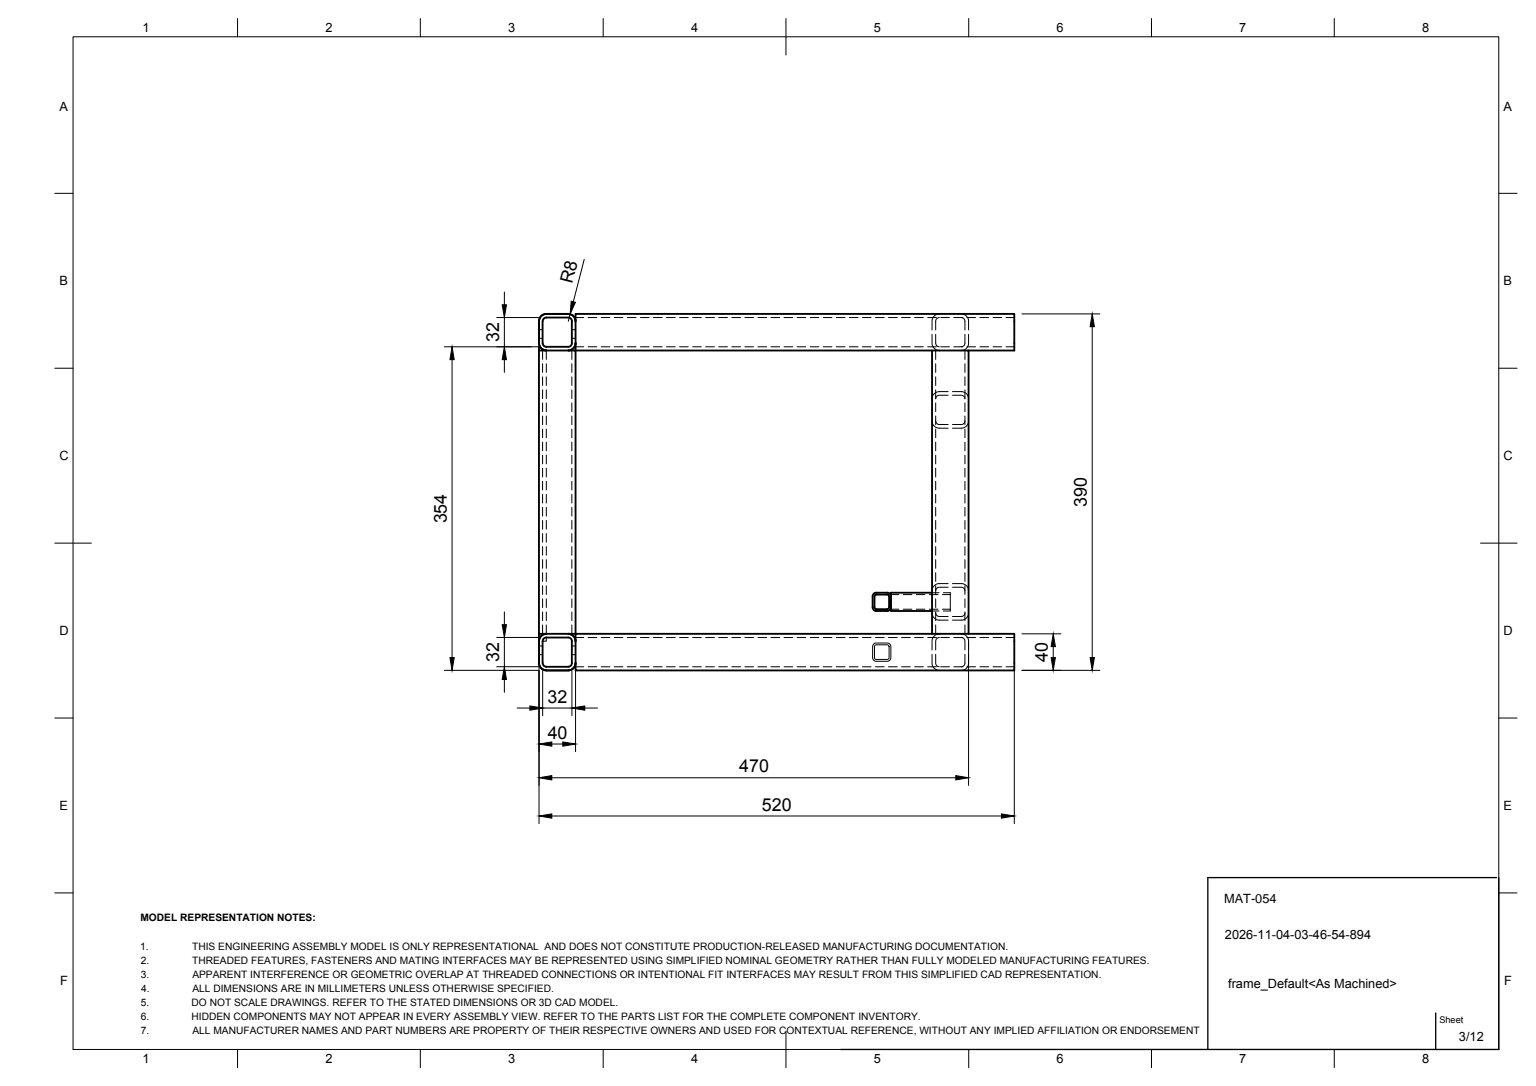
ISO-10303-21;
HEADER;
FILE_DESCRIPTION (('STEP AP214'),
    '1' );
FILE_NAME ('frame_Default<As Machined>.step',
    '2026-10-21T17:50:41',
    ( '' ),
    ( '' ),
    'SwSTEP 2.0',
    'SolidWorks 2026',
    '' );
FILE_SCHEMA (( 'AUTOMOTIVE_DESIGN' ));
ENDSEC;

DATA;
#1=CARTESIAN_POINT ( 'NONE',  ( -499.9999999999999432, -137.0000000000000000, -155.0000000000000000 ) ) ;
#4=CARTESIAN_POINT ( 'NONE',  ( -19.99999999999998934, 134.9999999999999432, -162.9999999999999432 ) ) ;
#6=DIRECTION ( 'NONE',  ( -0.000000000000000000, 0.000000000000000000, -1.000000000000000000 ) ) ;
#10=LINE ( 'NONE', #8370, #25873 ) ;
#17=CIRCLE ( 'NONE', #34681, 7.999999999999979572 ) ;
#21=LINE ( 'NONE', #19262, #12243 ) ;
#22=EDGE_CURVE ( 'NONE', #26361, #15713, #881, .T. ) ;
#25=LINE ( 'NONE', #27253, #34000 ) ;
#26=AXIS2_PLACEMENT_3D ( 'NONE', #32504, #14502, #28009 ) ;
#28=ORIENTED_EDGE ( 'NONE', *, *, #27270, .T. ) ;
#29=LINE ( 'NONE', #564, #14605 ) ;
#34=CARTESIAN_POINT ( 'NONE',  ( -449.9999999999999432, 137.0000000000000000, -175.0000000000000000 ) ) ;
#35=VERTEX_POINT ( 'NONE', #17374 ) ;
#37=DIRECTION ( 'NONE',  ( 0.000000000000000000, 1.000000000000000000, -3.421138828918010427E-49 ) ) ;
#39=ADVANCED_FACE ( 'NONE', ( #31052 ), #33181, .F. ) ;
#42=DIRECTION ( 'NONE',  ( 0.000000000000000000, -1.000000000000000000, -2.465190328815662439E-32 ) ) ;
#43=AXIS2_PLACEMENT_3D ( 'NONE', #14582, #6360, #9220 ) ;
#45=DIRECTION ( 'NONE',  ( 0.000000000000000000, -5.053935297177146739E-49, -1.000000000000000000 ) ) ;
#47=SHAPE_REPRESENTATION ( 'frame_Default<As Machined>', ( #28566 ), #4098 ) ;
#49=EDGE_LOOP ( 'NONE', ( #24690, #13383, #3512, #29102 ) ) ;
#51=CARTESIAN_POINT ( 'NONE',  ( 11.99999999999999645, 124.9999999999999716, 194.9999999999999716 ) ) ;
#52=DIRECTION ( 'NONE',  ( 1.000000000000000000, 0.000000000000000000, -1.848892746611746966E-32 ) ) ;
#60=ORIENTED_EDGE ( 'NONE', *, *, #3732, .F. ) ;
#61=DIRECTION ( 'NONE',  ( 0.000000000000000000, 6.123233995736766036E-17, 1.000000000000000000 ) ) ;
#63=ORIENTED_EDGE ( 'NONE', *, *, #23072, .F. ) ;
#68=EDGE_CURVE ( 'NONE', #14854, #22599, #23039, .T. ) ;
#73=ORIENTED_EDGE ( 'NONE', *, *, #26819, .F. ) ;
#74=DIRECTION ( 'NONE',  ( 0.000000000000000000, 0.000000000000000000, -1.000000000000000000 ) ) ;
#79=DIRECTION ( 'NONE',  ( 1.000000000000000000, 0.000000000000000000, -1.848892746611746966E-32 ) ) ;
#80=CIRCLE ( 'NONE', #11440, 7.999999999999979572 ) ;
#81=CARTESIAN_POINT ( 'NONE',  ( -365.0000000000000000, 118.9999999999999716, 130.0000000000000000 ) ) ;
#83=AXIS2_PLACEMENT_3D ( 'NONE', #4281, #34723, #15702 ) ;
#84=AXIS2_PLACEMENT_3D ( 'NONE', #29650, #6301, #461 ) ;
#87=DIRECTION ( 'NONE',  ( 0.000000000000000000, 1.310824597558155437E-49, 1.000000000000000000 ) ) ;
#90=ORIENTED_EDGE ( 'NONE', *, *, #18503, .T. ) ;
#91=FACE_OUTER_BOUND ( 'NONE', #10797, .T. ) ;
#93=CARTESIAN_POINT ( 'NONE',  ( -418.0000000000000000, -112.9999999999999858, -174.9999999999999716 ) ) ;
#94=CARTESIAN_POINT ( 'NONE',  ( -499.9999999999999432, 112.9999999999999574, 159.0000000000000000 ) ) ;
#96=VECTOR ( 'NONE', #6013, 1000.000000000000000 ) ;
#97=ORIENTED_EDGE ( 'NONE', *, *, #12534, .F. ) ;
#100=MANIFOLD_SOLID_BREP ( 'Square tube 40 X 40 X 4(1)[12]', #34815 ) ;
#101=ORIENTED_EDGE ( 'NONE', *, *, #29088, .F. ) ;
#103=AXIS2_PLACEMENT_3D ( 'NONE', #2451, #30043, #5636 ) ;
#104=AXIS2_PLACEMENT_3D ( 'NONE', #26124, #29507, #9931 ) ;
#106=CARTESIAN_POINT ( 'NONE',  ( -449.9999999999999432, -112.9999999999999858, -155.0000000000000000 ) ) ;
#108=VERTEX_POINT ( 'NONE', #26214 ) ;
#118=ORIENTED_EDGE ( 'NONE', *, *, #1367, .F. ) ;
#120=CARTESIAN_POINT ( 'NONE',  ( -418.0000000000000000, -105.0000000000000142, -73.99999999999998579 ) ) ;
#127=CARTESIAN_POINT ( 'NONE',  ( 11.99999999999999645, 124.9999999999999716, 190.9999999999999716 ) ) ;
#128=EDGE_LOOP ( 'NONE', ( #27295, #34610, #28913, #17445 ) ) ;
#130=EDGE_CURVE ( 'NONE', #18108, #30234, #23613, .T. ) ;
#132=CARTESIAN_POINT ( 'NONE',  ( -499.9999999999999432, 140.9999999999999716, -162.9999999999999716 ) ) ;
#135=CARTESIAN_POINT ( 'NONE',  ( -441.9999999999999432, -104.9999999999999716, -190.9999999999999716 ) ) ;
#139=ORIENTED_EDGE ( 'NONE', *, *, #14829, .T. ) ;
#140=CARTESIAN_POINT ( 'NONE',  ( -12.00000000000001066, -124.9999999999999432, -162.9999999999999432 ) ) ;
#143=VERTEX_POINT ( 'NONE', #21234 ) ;
#160=ORIENTED_EDGE ( 'NONE', *, *, #17632, .T. ) ;
#162=ORIENTED_EDGE ( 'NONE', *, *, #7088, .T. ) ;
#165=ADVANCED_FACE ( 'NONE', ( #4848 ), #1498, .F. ) ;
#166=DIRECTION ( 'NONE',  ( 1.000000000000000000, 0.000000000000000000, -1.232595164407831220E-32 ) ) ;
#169=VERTEX_POINT ( 'NONE', #10028 ) ;
#170=ADVANCED_FACE ( 'NONE', ( #26571 ), #17893, .T. ) ;
#172=DIRECTION ( 'NONE',  ( 0.000000000000000000, 1.310824597558155437E-49, 1.000000000000000000 ) ) ;
#173=VERTEX_POINT ( 'NONE', #23733 ) ;
#174=DIRECTION ( 'NONE',  ( -0.000000000000000000, 1.000000000000000000, -0.000000000000000000 ) ) ;
#178=ORIENTED_EDGE ( 'NONE', *, *, #30215, .F. ) ;
#181=VERTEX_POINT ( 'NONE', #21756 ) ;
#196=VERTEX_POINT ( 'NONE', #27097 ) ;
#203=CARTESIAN_POINT ( 'NONE',  ( -349.0000000000000000, 134.9999999999999716, 113.9999999999999858 ) ) ;
#204=FACE_OUTER_BOUND ( 'NONE', #17444, .T. ) ;
#208=ADVANCED_FACE ( 'NONE', ( #18929 ), #2537, .T. ) ;
#209=EDGE_CURVE ( 'NONE', #25754, #24825, #34950, .T. ) ;
#210=AXIS2_PLACEMENT_3D ( 'NONE', #14613, #8714, #19766 ) ;
#211=CARTESIAN_POINT ( 'NONE',  ( -15.99999999999998579, 124.9999999999999716, 162.9999999999999716 ) ) ;
#213=CYLINDRICAL_SURFACE ( 'NONE', #21558, 7.999999999999979572 ) ;
#216=ORIENTED_EDGE ( 'NONE', *, *, #5166, .F. ) ;
#217=CYLINDRICAL_SURFACE ( 'NONE', #9558, 3.999999999999976019 ) ;
#219=CARTESIAN_POINT ( 'NONE',  ( -500.0000000000000000, -137.0000000000000000, 190.9999999999999716 ) ) ;
#221=( NAMED_UNIT ( * ) PLANE_ANGLE_UNIT ( ) SI_UNIT ( $, .RADIAN. ) );
#228=ORIENTED_EDGE ( 'NONE', *, *, #6017, .T. ) ;
#229=DIRECTION ( 'NONE',  ( 1.000000000000000000, 0.000000000000000000, 0.000000000000000000 ) ) ;
#231=EDGE_CURVE ( 'NONE', #21456, #4465, #34436, .T. ) ;
#234=EDGE_CURVE ( 'NONE', #30170, #27211, #3153, .T. ) ;
#235=CIRCLE ( 'NONE', #12751, 3.999999999999976019 ) ;
#236=ORIENTED_EDGE ( 'NONE', *, *, #29739, .F. ) ;
#239=AXIS2_PLACEMENT_3D ( 'NONE', #27640, #18947, #27283 ) ;
#240=EDGE_CURVE ( 'NONE', #16352, #20441, #2589, .T. ) ;
#241=ORIENTED_EDGE ( 'NONE', *, *, #17416, .F. ) ;
#242=ORIENTED_EDGE ( 'NONE', *, *, #21753, .F. ) ;
#248=AXIS2_PLACEMENT_3D ( 'NONE', #6880, #17771, #4383 ) ;
#249=DIRECTION ( 'NONE',  ( -1.000000000000000000, 0.000000000000000000, 0.000000000000000000 ) ) ;
#250=CARTESIAN_POINT ( 'NONE',  ( -500.0000000000000000, 112.9999999999999574, 155.0000000000000000 ) ) ;
#259=ORIENTED_EDGE ( 'NONE', *, *, #5135, .T. ) ;
#260=ORIENTED_EDGE ( 'NONE', *, *, #32935, .F. ) ;
#262=VECTOR ( 'NONE', #31181, 1000.000000000000000 ) ;
#265=EDGE_LOOP ( 'NONE', ( #34746, #139, #23845, #12635, #26310, #31196, #6266, #393 ) ) ;
#266=CARTESIAN_POINT ( 'NONE',  ( 15.99999999999998579, 4.559999999999908127, 168.2400000000000091 ) ) ;
#281=CARTESIAN_POINT ( 'NONE',  ( -499.9999999999999432, -137.0000000000000000, -190.9999999999999716 ) ) ;
#284=EDGE_LOOP ( 'NONE', ( #25209, #30307, #21311, #18042 ) ) ;
#285=VECTOR ( 'NONE', #12711, 1000.000000000000000 ) ;
#287=VECTOR ( 'NONE', #30917, 1000.000000000000000 ) ;
#290=CARTESIAN_POINT ( 'NONE',  ( -418.0000000000000000, 113.0000000000000000, 154.9999999999999716 ) ) ;
#295=CARTESIAN_POINT ( 'NONE',  ( -445.9999999999999432, -137.0000000000000000, 154.9999999999999716 ) ) ;
#296=DIRECTION ( 'NONE',  ( 0.000000000000000000, 1.000000000000000000, 0.000000000000000000 ) ) ;
#299=ORIENTED_EDGE ( 'NONE', *, *, #29304, .T. ) ;
#300=DIRECTION ( 'NONE',  ( 1.000000000000000000, 3.040835319149746528E-31, 1.232595164407830946E-32 ) ) ;
#302=CARTESIAN_POINT ( 'NONE',  ( -12.00000000000001066, -109.0000000000000142, 155.0000000000000000 ) ) ;
#304=VECTOR ( 'NONE', #8203, 1000.000000000000000 ) ;
#309=VECTOR ( 'NONE', #16304, 1000.000000000000000 ) ;
#313=ORIENTED_EDGE ( 'NONE', *, *, #17871, .T. ) ;
#315=ORIENTED_EDGE ( 'NONE', *, *, #26179, .T. ) ;
#316=VECTOR ( 'NONE', #20254, 1000.000000000000000 ) ;
#317=VECTOR ( 'NONE', #9866, 1000.000000000000000 ) ;
#321=CARTESIAN_POINT ( 'NONE',  ( 11.99999999999999645, -124.9999999999999432, -154.9999999999999716 ) ) ;
#322=AXIS2_PLACEMENT_3D ( 'NONE', #10565, #32080, #10742 ) ;
#330=DIRECTION ( 'NONE',  ( 0.000000000000000000, -1.224646799147353207E-16, 1.000000000000000000 ) ) ;
#333=EDGE_LOOP ( 'NONE', ( #9601, #2215, #28741, #29275, #5602, #22316, #13085, #21357 ) ) ;
#337=AXIS2_PLACEMENT_3D ( 'NONE', #12188, #9323, #17539 ) ;
#338=PLANE ( 'NONE',  #21235 ) ;
#345=ORIENTED_EDGE ( 'NONE', *, *, #32175, .T. ) ;
#347=DIRECTION ( 'NONE',  ( 0.000000000000000000, -1.000000000000000000, -2.465190328815662439E-32 ) ) ;
#351=ORIENTED_EDGE ( 'NONE', *, *, #29532, .T. ) ;
#352=ORIENTED_EDGE ( 'NONE', *, *, #24437, .F. ) ;
#354=ORIENTED_EDGE ( 'NONE', *, *, #15930, .T. ) ;
#355=CARTESIAN_POINT ( 'NONE',  ( -20.00000000000007461, 104.9999999999999858, -162.9999999999999716 ) ) ;
#356=CARTESIAN_POINT ( 'NONE',  ( -414.0000000000000568, -124.9999999999999858, -77.99999999999997158 ) ) ;
#358=EDGE_LOOP ( 'NONE', ( #6537, #22025, #25095, #26334 ) ) ;
#359=CIRCLE ( 'NONE', #19122, 3.999999999999976019 ) ;
#362=DIRECTION ( 'NONE',  ( -0.000000000000000000, 1.000000000000000000, -0.000000000000000000 ) ) ;
#365=DIRECTION ( 'NONE',  ( 0.000000000000000000, 1.000000000000000000, 5.145227585319922065E-49 ) ) ;
#366=DIRECTION ( 'NONE',  ( 0.000000000000000000, 0.000000000000000000, 1.000000000000000000 ) ) ;
#367=EDGE_CURVE ( 'NONE', #31738, #21426, #28743, .T. ) ;
#368=LINE ( 'NONE', #5152, #16717 ) ;
#370=CARTESIAN_POINT ( 'NONE',  ( -19.99999999999998934, 144.9999999999999147, 162.9999999999999716 ) ) ;
#372=PLANE ( 'NONE',  #748 ) ;
#373=EDGE_CURVE ( 'NONE', #12936, #16352, #14295, .T. ) ;
#377=LINE ( 'NONE', #5513, #1804 ) ;
#386=CARTESIAN_POINT ( 'NONE',  ( -349.0000000000000000, -125.0000000000000284, 168.9999999999999716 ) ) ;
#387=AXIS2_PLACEMENT_3D ( 'NONE', #34628, #13273, #5228 ) ;
#388=CARTESIAN_POINT ( 'NONE',  ( -499.9999999999999432, 136.9999999999999432, -159.0000000000000000 ) ) ;
#390=DIRECTION ( 'NONE',  ( 0.000000000000000000, 0.000000000000000000, -1.000000000000000000 ) ) ;
#392=VERTEX_POINT ( 'NONE', #6605 ) ;
#393=ORIENTED_EDGE ( 'NONE', *, *, #6508, .T. ) ;
#395=CARTESIAN_POINT ( 'NONE',  ( -355.0000000000000000, 132.9999999999999716, 113.9999999999999858 ) ) ;
#396=AXIS2_PLACEMENT_3D ( 'NONE', #7173, #18412, #15218 ) ;
#397=LINE ( 'NONE', #6768, #1059 ) ;
#398=CARTESIAN_POINT ( 'NONE',  ( -499.9999999999999432, -137.0000000000000000, -159.0000000000000000 ) ) ;
#402=CARTESIAN_POINT ( 'NONE',  ( -363.0000000000000000, -135.0000000000000000, 114.0000000000000000 ) ) ;
#406=VECTOR ( 'NONE', #1614, 1000.000000000000000 ) ;
#407=DIRECTION ( 'NONE',  ( 0.000000000000000000, 6.123233995736766036E-17, 1.000000000000000000 ) ) ;
#411=CARTESIAN_POINT ( 'NONE',  ( -20.00000000000004619, -124.9999999999999432, -194.9999999999999432 ) ) ;
#413=DIRECTION ( 'NONE',  ( 1.000000000000000000, -0.000000000000000000, 0.000000000000000000 ) ) ;
#414=FACE_OUTER_BOUND ( 'NONE', #24829, .T. ) ;
#418=EDGE_CURVE ( 'NONE', #32157, #25965, #6244, .T. ) ;
#421=ORIENTED_EDGE ( 'NONE', *, *, #373, .F. ) ;
#423=VERTEX_POINT ( 'NONE', #6428 ) ;
#426=EDGE_CURVE ( 'NONE', #7666, #28875, #25652, .T. ) ;
#429=CARTESIAN_POINT ( 'NONE',  ( -418.0000000000000000, 124.9999999999999432, -162.9999999999999716 ) ) ;
#430=PLANE ( 'NONE',  #10872 ) ;
#440=EDGE_CURVE ( 'NONE', #10023, #18562, #30296, .T. ) ;
#443=DIRECTION ( 'NONE',  ( -0.000000000000000000, 1.000000000000000000, -0.000000000000000000 ) ) ;
#451=AXIS2_PLACEMENT_3D ( 'NONE', #17742, #12395, #1529 ) ;
#454=PLANE ( 'NONE',  #18923 ) ;
#457=ORIENTED_EDGE ( 'NONE', *, *, #17828, .T. ) ;
#459=ADVANCED_FACE ( 'NONE', ( #16977 ), #27625, .T. ) ;
#460=DIRECTION ( 'NONE',  ( -1.000000000000000000, 0.000000000000000000, -1.300283923313630633E-47 ) ) ;
#461=DIRECTION ( 'NONE',  ( -1.000000000000000000, 0.000000000000000000, 0.000000000000000000 ) ) ;
#463=ORIENTED_EDGE ( 'NONE', *, *, #15359, .T. ) ;
#464=AXIS2_PLACEMENT_3D ( 'NONE', #20405, #28583, #17576 ) ;
#465=ORIENTED_EDGE ( 'NONE', *, *, #4049, .T. ) ;
#468=ORIENTED_EDGE ( 'NONE', *, *, #12591, .T. ) ;
#470=CARTESIAN_POINT ( 'NONE',  ( -445.9999999999999432, 105.0000000000000000, -77.99999999999997158 ) ) ;
#473=CARTESIAN_POINT ( 'NONE',  ( -499.9999999999999432, 112.9999999999999574, -159.0000000000000000 ) ) ;
#476=CYLINDRICAL_SURFACE ( 'NONE', #3727, 7.999999999999979572 ) ;
#481=VECTOR ( 'NONE', #14446, 1000.000000000000000 ) ;
#490=CARTESIAN_POINT ( 'NONE',  ( -414.0000000000000568, 105.0000000000000000, 132.0000000000000000 ) ) ;
#493=VERTEX_POINT ( 'NONE', #26528 ) ;
#495=DIRECTION ( 'NONE',  ( 0.000000000000000000, 2.309213040847544338E-50, 1.000000000000000000 ) ) ;
#496=EDGE_LOOP ( 'NONE', ( #8671, #8496, #20597, #12284 ) ) ;
#497=DIRECTION ( 'NONE',  ( -5.546364386991661285E-52, 0.000000000000000000, -1.000000000000000000 ) ) ;
#499=VECTOR ( 'NONE', #8880, 1000.000000000000000 ) ;
#502=DIRECTION ( 'NONE',  ( 1.000000000000000000, 0.000000000000000000, -1.232595164407831220E-32 ) ) ;
#503=PLANE ( 'NONE',  #5402 ) ;
#510=FACE_OUTER_BOUND ( 'NONE', #7829, .T. ) ;
#512=LINE ( 'NONE', #33420, #24339 ) ;
#516=ORIENTED_EDGE ( 'NONE', *, *, #603, .F. ) ;
#518=ORIENTED_EDGE ( 'NONE', *, *, #18226, .F. ) ;
#519=DIRECTION ( 'NONE',  ( 0.000000000000000000, 1.131431318426415506E-52, 1.000000000000000000 ) ) ;
#520=ADVANCED_FACE ( 'NONE', ( #26170 ), #21018, .T. ) ;
#521=CARTESIAN_POINT ( 'NONE',  ( -20.00000000000007461, 112.9999999999999574, 162.9999999999999716 ) ) ;
#525=CIRCLE ( 'NONE', #16796, 7.999999999999979572 ) ;
#529=ORIENTED_EDGE ( 'NONE', *, *, #33922, .T. ) ;
#530=CYLINDRICAL_SURFACE ( 'NONE', #3882, 4.000000000000003553 ) ;
#531=CYLINDRICAL_SURFACE ( 'NONE', #29653, 7.999999999999979572 ) ;
#533=VECTOR ( 'NONE', #26637, 1000.000000000000000 ) ;
#534=ORIENTED_EDGE ( 'NONE', *, *, #6126, .F. ) ;
#540=PLANE ( 'NONE',  #20688 ) ;
#541=AXIS2_PLACEMENT_3D ( 'NONE', #20921, #31768, #29104 ) ;
#542=CARTESIAN_POINT ( 'NONE',  ( -499.9999999999999432, -113.0000000000000000, -162.9999999999999716 ) ) ;
#545=ORIENTED_EDGE ( 'NONE', *, *, #1677, .T. ) ;
#553=EDGE_CURVE ( 'NONE', #7666, #18883, #20841, .T. ) ;
#554=ORIENTED_EDGE ( 'NONE', *, *, #3009, .T. ) ;
#555=DIRECTION ( 'NONE',  ( 0.000000000000000000, 1.000000000000000000, 5.145227585319922065E-49 ) ) ;
#558=AXIS2_PLACEMENT_3D ( 'NONE', #28352, #26018, #20687 ) ;
#560=FACE_OUTER_BOUND ( 'NONE', #15965, .T. ) ;
#561=CARTESIAN_POINT ( 'NONE',  ( -410.0000000000000568, 104.9999999999999858, -175.0000000000000000 ) ) ;
#563=ORIENTED_EDGE ( 'NONE', *, *, #30172, .T. ) ;
#564=CARTESIAN_POINT ( 'NONE',  ( -499.9999999999999432, 136.9999999999999432, -155.0000000000000000 ) ) ;
#567=DIRECTION ( 'NONE',  ( 1.000000000000000000, 0.000000000000000000, 0.000000000000000000 ) ) ;
#568=DIRECTION ( 'NONE',  ( 0.000000000000000000, -1.000000000000000000, 0.000000000000000000 ) ) ;
#569=ORIENTED_EDGE ( 'NONE', *, *, #971, .T. ) ;
#571=DIRECTION ( 'NONE',  ( 1.000000000000000000, 0.000000000000000000, -1.848892746611746966E-32 ) ) ;
#573=ORIENTED_EDGE ( 'NONE', *, *, #23821, .T. ) ;
#574=LINE ( 'NONE', #16262, #35090 ) ;
#575=CARTESIAN_POINT ( 'NONE',  ( -418.0000000000000000, -145.0000000000000000, -175.0000000000000000 ) ) ;
#576=EDGE_CURVE ( 'NONE', #19034, #23318, #12495, .T. ) ;
#577=CARTESIAN_POINT ( 'NONE',  ( -499.9999999999999432, 136.9999999999999432, -190.9999999999999716 ) ) ;
#580=DIRECTION ( 'NONE',  ( 0.000000000000000000, 1.000000000000000000, 5.145227585319922065E-49 ) ) ;
#581=ORIENTED_EDGE ( 'NONE', *, *, #14404, .F. ) ;
#582=DIRECTION ( 'NONE',  ( 0.000000000000000000, 1.310824597558155437E-49, 1.000000000000000000 ) ) ;
#586=ORIENTED_EDGE ( 'NONE', *, *, #10577, .T. ) ;
#591=VERTEX_POINT ( 'NONE', #18194 ) ;
#596=LINE ( 'NONE', #19835, #27348 ) ;
#599=FACE_OUTER_BOUND ( 'NONE', #6843, .T. ) ;
#601=LINE ( 'NONE', #17003, #7250 ) ;
#603=EDGE_CURVE ( 'NONE', #26714, #17291, #15511, .T. ) ;
#606=DIRECTION ( 'NONE',  ( -0.000000000000000000, 1.000000000000000000, -0.000000000000000000 ) ) ;
#618=CARTESIAN_POINT ( 'NONE',  ( 15.99999999999998579, 4.559999999999908127, -172.9900000000000091 ) ) ;
#621=LINE ( 'NONE', #27139, #28055 ) ;
#623=ORIENTED_EDGE ( 'NONE', *, *, #12621, .T. ) ;
#626=EDGE_CURVE ( 'NONE', #20682, #8601, #10335, .T. ) ;
#627=ORIENTED_EDGE ( 'NONE', *, *, #29512, .F. ) ;
#629=CARTESIAN_POINT ( 'NONE',  ( 12.00000000000001066, -134.9999999999999716, 194.9999999999999716 ) ) ;
#630=AXIS2_PLACEMENT_3D ( 'NONE', #7025, #15243, #23764 ) ;
#632=AXIS2_PLACEMENT_3D ( 'NONE', #14720, #8823, #19878 ) ;
#639=VERTEX_POINT ( 'NONE', #21379 ) ;
#643=CARTESIAN_POINT ( 'NONE',  ( 11.99999999999995559, -145.0000000000000000, 194.9999999999999716 ) ) ;
#651=STYLED_ITEM('',(#35254),#22717);
#652=LINE ( 'NONE', #11513, #1580 ) ;
#654=CARTESIAN_POINT ( 'NONE',  ( -70.00000000000000000, 75.55999999999990280, -172.9900000000000091 ) ) ;
#656=ADVANCED_FACE ( 'NONE', ( #2312 ), #27058, .F. ) ;
#658=CARTESIAN_POINT ( 'NONE',  ( 12.00000000000001066, 134.9999999999999432, -154.9999999999999716 ) ) ;
#664=LINE ( 'NONE', #5982, #1831 ) ;
#665=ORIENTED_EDGE ( 'NONE', *, *, #8099, .F. ) ;
#666=FACE_OUTER_BOUND ( 'NONE', #16803, .T. ) ;
#672=ORIENTED_EDGE ( 'NONE', *, *, #22907, .F. ) ;
#677=LINE ( 'NONE', #11000, #15466 ) ;
#678=CIRCLE ( 'NONE', #20570, 3.999999999999976019 ) ;
#687=EDGE_CURVE ( 'NONE', #28835, #181, #8010, .T. ) ;
#688=VECTOR ( 'NONE', #24666, 1000.000000000000000 ) ;
#690=DIRECTION ( 'NONE',  ( -1.000000000000000000, 8.433758354584418579E-81, -1.232595164407830946E-32 ) ) ;
#692=ORIENTED_EDGE ( 'NONE', *, *, #2681, .F. ) ;
#695=PRODUCT ( 'frame_Default<As Machined>', 'frame_Default<As Machined>', '', ( #11065 ) ) ;
#697=CIRCLE ( 'NONE', #1800, 4.750000000000004441 ) ;
#699=AXIS2_PLACEMENT_3D ( 'NONE', #32555, #29554, #17888 ) ;
#703=AXIS2_PLACEMENT_3D ( 'NONE', #2442, #2103, #14812 ) ;
#705=DIRECTION ( 'NONE',  ( 0.000000000000000000, 0.000000000000000000, 1.000000000000000000 ) ) ;
#707=VERTEX_POINT ( 'NONE', #16225 ) ;
#709=( NAMED_UNIT ( * ) PLANE_ANGLE_UNIT ( ) SI_UNIT ( $, .RADIAN. ) );
#711=ORIENTED_EDGE ( 'NONE', *, *, #4540, .T. ) ;
#714=CARTESIAN_POINT ( 'NONE',  ( -500.0000000000000000, -113.0000000000000000, 194.9999999999999716 ) ) ;
#718=ORIENTED_EDGE ( 'NONE', *, *, #26278, .T. ) ;
#721=EDGE_CURVE ( 'NONE', #11831, #17160, #30086, .T. ) ;
#722=ORIENTED_EDGE ( 'NONE', *, *, #5518, .F. ) ;
#726=VERTEX_POINT ( 'NONE', #16403 ) ;
#727=ORIENTED_EDGE ( 'NONE', *, *, #801, .T. ) ;
#728=DIRECTION ( 'NONE',  ( 0.000000000000000000, 1.000000000000000000, 0.000000000000000000 ) ) ;
#734=CARTESIAN_POINT ( 'NONE',  ( -500.0000000000000000, -137.0000000000000000, 187.0000000000000000 ) ) ;
#735=CARTESIAN_POINT ( 'NONE',  ( -500.0000000000000000, -137.0000000000000000, 159.0000000000000000 ) ) ;
#737=ORIENTED_EDGE ( 'NONE', *, *, #1707, .T. ) ;
#739=DIRECTION ( 'NONE',  ( 1.000000000000000000, 0.000000000000000000, 0.000000000000000000 ) ) ;
#745=CYLINDRICAL_SURFACE ( 'NONE', #8305, 7.999999999999979572 ) ;
#746=DIRECTION ( 'NONE',  ( -1.000000000000000000, 0.000000000000000000, -1.300283923313630633E-47 ) ) ;
#748=AXIS2_PLACEMENT_3D ( 'NONE', #8542, #14074, #33456 ) ;
#753=PLANE ( 'NONE',  #13835 ) ;
#759=CARTESIAN_POINT ( 'NONE',  ( -363.0000000000000000, -135.0000000000000000, 114.0000000000000000 ) ) ;
#760=DIRECTION ( 'NONE',  ( -0.000000000000000000, -5.145227585319922065E-49, -1.000000000000000000 ) ) ;
#761=EDGE_CURVE ( 'NONE', #19084, #9157, #24545, .T. ) ;
#763=VERTEX_POINT ( 'NONE', #5153 ) ;
#768=VECTOR ( 'NONE', #8009, 1000.000000000000000 ) ;
#770=CARTESIAN_POINT ( 'NONE',  ( -442.0000000000000000, -125.0000000000000000, -105.9999999999999574 ) ) ;
#773=CARTESIAN_POINT ( 'NONE',  ( -499.9999999999999432, -113.0000000000000000, -162.9999999999999716 ) ) ;
#774=ORIENTED_EDGE ( 'NONE', *, *, #8706, .F. ) ;
#775=LINE ( 'NONE', #34040, #30580 ) ;
#777=ORIENTED_EDGE ( 'NONE', *, *, #34334, .F. ) ;
#778=ORIENTED_EDGE ( 'NONE', *, *, #32742, .T. ) ;
#779=FACE_OUTER_BOUND ( 'NONE', #30050, .T. ) ;
#780=DIRECTION ( 'NONE',  ( 0.000000000000000000, 1.000000000000000000, 5.145227585319922065E-49 ) ) ;
#782=DIRECTION ( 'NONE',  ( 0.000000000000000000, 1.000000000000000000, 2.465190328815662439E-32 ) ) ;
#783=PLANE ( 'NONE',  #1217 ) ;
#785=CARTESIAN_POINT ( 'NONE',  ( -20.00000000000007461, 136.9999999999999432, 190.9999999999999716 ) ) ;
#788=ORIENTED_EDGE ( 'NONE', *, *, #21266, .F. ) ;
#789=CARTESIAN_POINT ( 'NONE',  ( -499.9999999999999432, 112.9999999999999574, 190.9999999999999716 ) ) ;
#793=LINE ( 'NONE', #15037, #16102 ) ;
#794=AXIS2_PLACEMENT_3D ( 'NONE', #34240, #4849, #18070 ) ;
#800=FACE_OUTER_BOUND ( 'NONE', #12597, .T. ) ;
#801=EDGE_CURVE ( 'NONE', #5991, #17491, #18552, .T. ) ;
#809=EDGE_CURVE ( 'NONE', #1130, #16248, #20815, .T. ) ;
#813=ORIENTED_EDGE ( 'NONE', *, *, #20854, .T. ) ;
#817=EDGE_CURVE ( 'NONE', #591, #27019, #22610, .T. ) ;
#819=LINE ( 'NONE', #5782, #3363 ) ;
#820=AXIS2_PLACEMENT_3D ( 'NONE', #3238, #14113, #27797 ) ;
#823=ORIENTED_EDGE ( 'NONE', *, *, #1952, .F. ) ;
#825=AXIS2_PLACEMENT_3D ( 'NONE', #30486, #20162, #31187 ) ;
#829=DIRECTION ( 'NONE',  ( 0.000000000000000000, 0.000000000000000000, -1.000000000000000000 ) ) ;
#832=LINE ( 'NONE', #5974, #7684 ) ;
#836=CARTESIAN_POINT ( 'NONE',  ( -15.99999999999998579, 136.9999999999999716, -175.0000000000000284 ) ) ;
#837=DIRECTION ( 'NONE',  ( 0.000000000000000000, 1.000000000000000000, 1.224646799147353207E-16 ) ) ;
#838=ORIENTED_EDGE ( 'NONE', *, *, #33279, .T. ) ;
#841=DIRECTION ( 'NONE',  ( 0.000000000000000000, -1.000000000000000000, 6.123233995736766036E-17 ) ) ;
#842=VERTEX_POINT ( 'NONE', #31436 ) ;
#844=CARTESIAN_POINT ( 'NONE',  ( -365.0000000000000000, 130.9999999999999716, 111.9999999999999858 ) ) ;
#847=CARTESIAN_POINT ( 'NONE',  ( -349.0000000000000000, 134.9999999999999716, 126.0000000000000000 ) ) ;
#849=ORIENTED_EDGE ( 'NONE', *, *, #21052, .T. ) ;
#851=FACE_OUTER_BOUND ( 'NONE', #26589, .T. ) ;
#854=VECTOR ( 'NONE', #2989, 1000.000000000000000 ) ;
#857=ADVANCED_FACE ( 'NONE', ( #30253 ), #22251, .F. ) ;
#862=CARTESIAN_POINT ( 'NONE',  ( -430.0000000000000000, -119.0000000000000000, 111.9999999999999858 ) ) ;
#864=CIRCLE ( 'NONE', #19071, 4.000000000000003553 ) ;
#867=ORIENTED_EDGE ( 'NONE', *, *, #33939, .F. ) ;
#868=ORIENTED_EDGE ( 'NONE', *, *, #240, .F. ) ;
#871=VECTOR ( 'NONE', #29284, 1000.000000000000000 ) ;
#873=DIRECTION ( 'NONE',  ( 1.000000000000000000, 0.000000000000000000, 0.000000000000000000 ) ) ;
#874=DIRECTION ( 'NONE',  ( 0.000000000000000000, 0.000000000000000000, 1.000000000000000000 ) ) ;
#875=FACE_OUTER_BOUND ( 'NONE', #18381, .T. ) ;
#877=ORIENTED_EDGE ( 'NONE', *, *, #2719, .T. ) ;
#878=AXIS2_PLACEMENT_3D ( 'NONE', #15837, #32184, #18849 ) ;
#879=DIRECTION ( 'NONE',  ( 0.000000000000000000, 0.000000000000000000, -1.000000000000000000 ) ) ;
#881=CIRCLE ( 'NONE', #13382, 4.750000000000004441 ) ;
#882=EDGE_CURVE ( 'NONE', #28417, #9255, #19687, .T. ) ;
#883=CARTESIAN_POINT ( 'NONE',  ( -442.0000000000000000, -124.9999999999999858, -77.99999999999997158 ) ) ;
#884=DIRECTION ( 'NONE',  ( 0.000000000000000000, 0.000000000000000000, -1.000000000000000000 ) ) ;
#887=EDGE_CURVE ( 'NONE', #24475, #21957, #33276, .T. ) ;
#888=FACE_OUTER_BOUND ( 'NONE', #22918, .T. ) ;
#889=CYLINDRICAL_SURFACE ( 'NONE', #9256, 3.999999999999976019 ) ;
#890=VERTEX_POINT ( 'NONE', #25929 ) ;
#892=CARTESIAN_POINT ( 'NONE',  ( 15.99999999999998579, -137.0000000000000000, -155.0000000000000284 ) ) ;
#895=VECTOR ( 'NONE', #17120, 1000.000000000000000 ) ;
#897=DIRECTION ( 'NONE',  ( 0.000000000000000000, 0.000000000000000000, 1.000000000000000000 ) ) ;
#898=AXIS2_PLACEMENT_3D ( 'NONE', #26736, #2349, #13228 ) ;
#899=ORIENTED_EDGE ( 'NONE', *, *, #20430, .F. ) ;
#901=EDGE_CURVE ( 'NONE', #33356, #2161, #3374, .T. ) ;
#904=VERTEX_POINT ( 'NONE', #6207 ) ;
#905=AXIS2_PLACEMENT_3D ( 'NONE', #32431, #24589, #8050 ) ;
#910=ORIENTED_EDGE ( 'NONE', *, *, #5324, .F. ) ;
#911=CARTESIAN_POINT ( 'NONE',  ( -365.0000000000000000, -117.0000000000000000, 113.9999999999999858 ) ) ;
#914=CARTESIAN_POINT ( 'NONE',  ( -363.0000000000000000, -135.0000000000000000, 126.0000000000000000 ) ) ;
#918=CARTESIAN_POINT ( 'NONE',  ( -449.9999999999999432, -124.9999999999999716, 132.0000000000000000 ) ) ;
#920=DIRECTION ( 'NONE',  ( 0.000000000000000000, 0.000000000000000000, -1.000000000000000000 ) ) ;
#921=CARTESIAN_POINT ( 'NONE',  ( -449.9999999999999432, -125.0000000000000000, 187.0000000000000000 ) ) ;
#922=DIRECTION ( 'NONE',  ( 1.000000000000000000, -0.000000000000000000, 0.000000000000000000 ) ) ;
#924=EDGE_CURVE ( 'NONE', #20300, #23023, #4196, .T. ) ;
#927=CARTESIAN_POINT ( 'NONE',  ( -19.99999999999998934, 124.9999999999999716, 155.0000000000000000 ) ) ;
#928=ORIENTED_EDGE ( 'NONE', *, *, #4882, .F. ) ;
#931=CARTESIAN_POINT ( 'NONE',  ( -499.9999999999999432, 136.9999999999999432, -159.0000000000000000 ) ) ;
#935=AXIS2_PLACEMENT_3D ( 'NONE', #4865, #34789, #15576 ) ;
#941=DIRECTION ( 'NONE',  ( -1.000000000000000000, 0.000000000000000000, 0.000000000000000000 ) ) ;
#944=ORIENTED_EDGE ( 'NONE', *, *, #27551, .T. ) ;
#945=CIRCLE ( 'NONE', #12819, 4.000000000000003553 ) ;
#948=CARTESIAN_POINT ( 'NONE',  ( -12.00000000000001066, 104.9999999999999858, -155.0000000000000000 ) ) ;
#953=VECTOR ( 'NONE', #12900, 1000.000000000000000 ) ;
#955=ORIENTED_EDGE ( 'NONE', *, *, #9993, .T. ) ;
#957=DIRECTION ( 'NONE',  ( 0.000000000000000000, 0.000000000000000000, -1.000000000000000000 ) ) ;
#958=EDGE_LOOP ( 'NONE', ( #8878, #27960, #18209, #24992 ) ) ;
#959=ORIENTED_EDGE ( 'NONE', *, *, #2723, .T. ) ;
#961=DIRECTION ( 'NONE',  ( -1.000000000000000000, 0.000000000000000000, 0.000000000000000000 ) ) ;
#966=CARTESIAN_POINT ( 'NONE',  ( -12.00000000000003908, -134.9999999999999716, -154.9999999999999716 ) ) ;
#967=ORIENTED_EDGE ( 'NONE', *, *, #21553, .T. ) ;
#969=AXIS2_PLACEMENT_3D ( 'NONE', #27218, #29899, #2828 ) ;
#970=DIRECTION ( 'NONE',  ( 1.000000000000000000, 0.000000000000000000, -1.232595164407831220E-32 ) ) ;
#971=EDGE_CURVE ( 'NONE', #5416, #26553, #2066, .T. ) ;
#973=ORIENTED_EDGE ( 'NONE', *, *, #9241, .T. ) ;
#974=DIRECTION ( 'NONE',  ( -0.000000000000000000, 1.000000000000000000, 0.000000000000000000 ) ) ;
#977=PLANE ( 'NONE',  #12699 ) ;
#978=DIRECTION ( 'NONE',  ( 1.000000000000000000, 0.000000000000000000, 0.000000000000000000 ) ) ;
#980=VERTEX_POINT ( 'NONE', #12938 ) ;
#983=PLANE ( 'NONE',  #23120 ) ;
#986=FACE_OUTER_BOUND ( 'NONE', #14814, .T. ) ;
#988=ORIENTED_EDGE ( 'NONE', *, *, #13058, .F. ) ;
#993=CARTESIAN_POINT ( 'NONE',  ( -445.9999999999999432, 104.9999999999999858, -162.9999999999999716 ) ) ;
#995=VERTEX_POINT ( 'NONE', #18457 ) ;
#1000=LINE ( 'NONE', #22721, #30171 ) ;
#1001=VERTEX_POINT ( 'NONE', #4369 ) ;
#1005=DIRECTION ( 'NONE',  ( 1.000000000000000000, -0.000000000000000000, -0.000000000000000000 ) ) ;
#1007=EDGE_CURVE ( 'NONE', #10470, #34124, #5457, .T. ) ;
#1014=ORIENTED_EDGE ( 'NONE', *, *, #28076, .T. ) ;
#1016=LINE ( 'NONE', #17232, #19707 ) ;
#1017=DIRECTION ( 'NONE',  ( 0.000000000000000000, 1.310824597558155437E-49, 1.000000000000000000 ) ) ;
#1019=EDGE_LOOP ( 'NONE', ( #8379, #30017, #22732, #21816 ) ) ;
#1020=AXIS2_PLACEMENT_3D ( 'NONE', #3481, #19182, #27167 ) ;
#1025=EDGE_CURVE ( 'NONE', #26862, #18446, #31608, .T. ) ;
#1027=ORIENTED_EDGE ( 'NONE', *, *, #16202, .T. ) ;
#1028=DIRECTION ( 'NONE',  ( -3.040835319149746090E-31, -1.000000000000000000, 3.748118910144520367E-63 ) ) ;
#1031=VERTEX_POINT ( 'NONE', #26619 ) ;
#1034=ORIENTED_EDGE ( 'NONE', *, *, #29447, .F. ) ;
#1035=FACE_BOUND ( 'NONE', #9089, .T. ) ;
#1036=FACE_OUTER_BOUND ( 'NONE', #26947, .T. ) ;
#1038=VECTOR ( 'NONE', #10976, 1000.000000000000000 ) ;
#1042=ORIENTED_EDGE ( 'NONE', *, *, #9870, .T. ) ;
#1044=ORIENTED_EDGE ( 'NONE', *, *, #6337, .F. ) ;
#1046=PLANE ( 'NONE',  #15456 ) ;
#1047=AXIS2_PLACEMENT_3D ( 'NONE', #8394, #6728, #13919 ) ;
#1055=EDGE_CURVE ( 'NONE', #26315, #29922, #21463, .T. ) ;
#1058=DIRECTION ( 'NONE',  ( -1.000000000000000000, -3.469446951953834515E-18, 0.000000000000000000 ) ) ;
#1059=VECTOR ( 'NONE', #20484, 1000.000000000000000 ) ;
#1068=LINE ( 'NONE', #892, #6351 ) ;
#1069=CARTESIAN_POINT ( 'NONE',  ( 19.99999999999998224, 134.9999999999998863, 187.0000000000000000 ) ) ;
#1070=CIRCLE ( 'NONE', #29493, 4.750000000000004441 ) ;
#1072=DIRECTION ( 'NONE',  ( -1.000000000000000000, 0.000000000000000000, -1.300283923313630633E-47 ) ) ;
#1073=CARTESIAN_POINT ( 'NONE',  ( 19.99999999999998224, 134.9999999999999432, -186.9999999999999716 ) ) ;
#1076=ORIENTED_EDGE ( 'NONE', *, *, #23191, .F. ) ;
#1086=DIRECTION ( 'NONE',  ( -1.000000000000000000, 0.000000000000000000, 0.000000000000000000 ) ) ;
#1092=DIRECTION ( 'NONE',  ( -1.000000000000000000, 0.000000000000000000, 0.000000000000000000 ) ) ;
#1094=DIRECTION ( 'NONE',  ( 0.000000000000000000, 1.131431318426415506E-52, 1.000000000000000000 ) ) ;
#1095=VERTEX_POINT ( 'NONE', #3288 ) ;
#1107=CARTESIAN_POINT ( 'NONE',  ( -418.0000000000000000, 105.0000000000000000, -69.99999999999998579 ) ) ;
#1109=CARTESIAN_POINT ( 'NONE',  ( 19.99999999999998224, 134.9999999999998863, 187.0000000000000000 ) ) ;
#1111=ORIENTED_EDGE ( 'NONE', *, *, #27207, .F. ) ;
#1115=ORIENTED_EDGE ( 'NONE', *, *, #13293, .F. ) ;
#1117=MANIFOLD_SOLID_BREP ( 'Trim/Extend7[2]', #17953 ) ;
#1118=ORIENTED_EDGE ( 'NONE', *, *, #5241, .F. ) ;
#1120=EDGE_CURVE ( 'NONE', #3592, #3718, #32998, .T. ) ;
#1128=EDGE_CURVE ( 'NONE', #20858, #2088, #19713, .T. ) ;
#1130=VERTEX_POINT ( 'NONE', #8097 ) ;
#1131=FACE_OUTER_BOUND ( 'NONE', #17761, .T. ) ;
#1133=EDGE_LOOP ( 'NONE', ( #18626, #22635, #27907, #4390 ) ) ;
#1136=EDGE_CURVE ( 'NONE', #1031, #6516, #13984, .T. ) ;
#1138=CARTESIAN_POINT ( 'NONE',  ( 19.99999999999998934, 75.55999999999990280, 168.2400000000000091 ) ) ;
#1141=ORIENTED_EDGE ( 'NONE', *, *, #31612, .T. ) ;
#1142=DIRECTION ( 'NONE',  ( 1.000000000000000000, 0.000000000000000000, 0.000000000000000000 ) ) ;
#1144=ADVANCED_FACE ( 'NONE', ( #8622 ), #16847, .T. ) ;
#1145=DIRECTION ( 'NONE',  ( 0.000000000000000000, -1.000000000000000000, 6.123233995736766036E-17 ) ) ;
#1147=CARTESIAN_POINT ( 'NONE',  ( -363.0000000000000000, -125.0000000000000284, 168.9999999999999716 ) ) ;
#1154=VERTEX_POINT ( 'NONE', #20032 ) ;
#1155=DIRECTION ( 'NONE',  ( 0.000000000000000000, 1.131431318426415506E-52, 1.000000000000000000 ) ) ;
#1157=LINE ( 'NONE', #19859, #27644 ) ;
#1158=ORIENTED_EDGE ( 'NONE', *, *, #23185, .T. ) ;
#1161=EDGE_CURVE ( 'NONE', #29789, #12936, #20296, .T. ) ;
#1163=ORIENTED_EDGE ( 'NONE', *, *, #33703, .T. ) ;
#1167=CYLINDRICAL_SURFACE ( 'NONE', #24085, 2.000000000000001776 ) ;
#1168=VECTOR ( 'NONE', #26116, 1000.000000000000000 ) ;
#1170=DIRECTION ( 'NONE',  ( 0.000000000000000000, 1.000000000000000000, -3.374343856708137958E-53 ) ) ;
#1171=CYLINDRICAL_SURFACE ( 'NONE', #632, 7.999999999999979572 ) ;
#1174=CARTESIAN_POINT ( 'NONE',  ( -365.0000000000000000, -125.0000000000000000, 130.0000000000000000 ) ) ;
#1175=CARTESIAN_POINT ( 'NONE',  ( -365.0000000000000000, 124.9999999999999432, 168.9999999999999716 ) ) ;
#1177=LINE ( 'NONE', #20748, #30629 ) ;
#1178=FACE_OUTER_BOUND ( 'NONE', #24175, .T. ) ;
#1180=CIRCLE ( 'NONE', #15390, 4.750000000000004441 ) ;
#1181=DIRECTION ( 'NONE',  ( 0.000000000000000000, 0.000000000000000000, 1.000000000000000000 ) ) ;
#1182=ORIENTED_EDGE ( 'NONE', *, *, #5883, .F. ) ;
#1186=FACE_OUTER_BOUND ( 'NONE', #18294, .T. ) ;
#1188=CYLINDRICAL_SURFACE ( 'NONE', #33151, 7.999999999999979572 ) ;
#1189=EDGE_LOOP ( 'NONE', ( #29261, #25620, #10327, #29887 ) ) ;
#1190=CIRCLE ( 'NONE', #33002, 3.999999999999976019 ) ;
#1192=DIRECTION ( 'NONE',  ( 0.000000000000000000, 0.000000000000000000, 1.000000000000000000 ) ) ;
#1193=VECTOR ( 'NONE', #14137, 1000.000000000000000 ) ;
#1199=EDGE_CURVE ( 'NONE', #9586, #15011, #14704, .T. ) ;
#1200=ORIENTED_EDGE ( 'NONE', *, *, #8308, .T. ) ;
#1201=ADVANCED_FACE ( 'NONE', ( #800 ), #983, .T. ) ;
#1202=AXIS2_PLACEMENT_3D ( 'NONE', #18750, #32418, #8038 ) ;
#1208=ORIENTED_EDGE ( 'NONE', *, *, #8140, .F. ) ;
#1210=DIRECTION ( 'NONE',  ( 0.000000000000000000, 0.000000000000000000, 1.000000000000000000 ) ) ;
#1211=CARTESIAN_POINT ( 'NONE',  ( -12.00000000000001066, -124.9999999999999432, -154.9999999999999716 ) ) ;
#1212=DIRECTION ( 'NONE',  ( 0.000000000000000000, 0.000000000000000000, 1.000000000000000000 ) ) ;
#1214=VERTEX_POINT ( 'NONE', #1505 ) ;
#1217=AXIS2_PLACEMENT_3D ( 'NONE', #8786, #19668, #24975 ) ;
#1228=CYLINDRICAL_SURFACE ( 'NONE', #34024, 3.999999999999976019 ) ;
#1230=ORIENTED_EDGE ( 'NONE', *, *, #16119, .T. ) ;
#1233=AXIS2_PLACEMENT_3D ( 'NONE', #17065, #502, #30744 ) ;
#1234=CARTESIAN_POINT ( 'NONE',  ( -500.0000000000000000, -113.0000000000000000, 162.9999999999999716 ) ) ;
#1235=VERTEX_POINT ( 'NONE', #11854 ) ;
#1240=CARTESIAN_POINT ( 'NONE',  ( -365.0000000000000000, -125.0000000000000284, 181.0000000000000000 ) ) ;
#1242=PLANE ( 'NONE',  #3525 ) ;
#1243=EDGE_CURVE ( 'NONE', #14225, #17403, #32769, .T. ) ;
#1245=CIRCLE ( 'NONE', #12552, 3.999999999999976019 ) ;
#1248=EDGE_CURVE ( 'NONE', #32323, #27667, #1157, .T. ) ;
#1252=AXIS2_PLACEMENT_3D ( 'NONE', #26130, #7779, #13322 ) ;
#1257=CIRCLE ( 'NONE', #25693, 2.000000000000001776 ) ;
#1258=ORIENTED_EDGE ( 'NONE', *, *, #33383, .F. ) ;
#1260=CARTESIAN_POINT ( 'NONE',  ( -442.0000000000000000, 104.9999999999999858, -194.9999999999999716 ) ) ;
#1264=CARTESIAN_POINT ( 'NONE',  ( -499.9999999999999432, 136.9999999999999432, 159.0000000000000000 ) ) ;
#1265=ORIENTED_EDGE ( 'NONE', *, *, #24062, .T. ) ;
#1266=ORIENTED_EDGE ( 'NONE', *, *, #34069, .F. ) ;
#1271=DIRECTION ( 'NONE',  ( 0.000000000000000000, -1.000000000000000000, 0.000000000000000000 ) ) ;
#1274=ORIENTED_EDGE ( 'NONE', *, *, #32043, .F. ) ;
#1279=DIRECTION ( 'NONE',  ( 0.000000000000000000, 0.000000000000000000, -1.000000000000000000 ) ) ;
#1283=LINE ( 'NONE', #12153, #22975 ) ;
#1285=EDGE_LOOP ( 'NONE', ( #25859, #17008, #10345, #31825 ) ) ;
#1287=FACE_OUTER_BOUND ( 'NONE', #34679, .T. ) ;
#1289=ORIENTED_EDGE ( 'NONE', *, *, #2239, .T. ) ;
#1290=VERTEX_POINT ( 'NONE', #12025 ) ;
#1295=ORIENTED_EDGE ( 'NONE', *, *, #18930, .T. ) ;
#1296=VERTEX_POINT ( 'NONE', #3457 ) ;
#1298=CARTESIAN_POINT ( 'NONE',  ( -349.0000000000000000, -125.0000000000000284, 183.0000000000000000 ) ) ;
#1303=AXIS2_PLACEMENT_3D ( 'NONE', #31389, #29379, #10696 ) ;
#1304=DIRECTION ( 'NONE',  ( -1.000000000000000000, 0.000000000000000000, -0.000000000000000000 ) ) ;
#1306=AXIS2_PLACEMENT_3D ( 'NONE', #10338, #21198, #18723 ) ;
#1311=CARTESIAN_POINT ( 'NONE',  ( 11.99999999999999645, 124.9999999999999716, 159.0000000000000000 ) ) ;
#1317=CARTESIAN_POINT ( 'NONE',  ( -430.0000000000000000, 134.9999999999999716, 113.9999999999999858 ) ) ;
#1318=CARTESIAN_POINT ( 'NONE',  ( -355.0000000000000000, -133.0000000000000000, 126.0000000000000000 ) ) ;
#1319=ORIENTED_EDGE ( 'NONE', *, *, #1542, .F. ) ;
#1320=CARTESIAN_POINT ( 'NONE',  ( -449.9999999999999432, 137.0000000000000000, 154.9999999999999716 ) ) ;
#1322=ADVANCED_FACE ( 'NONE', ( #2195 ), #1844, .T. ) ;
#1323=DIRECTION ( 'NONE',  ( 0.000000000000000000, 1.000000000000000000, 0.000000000000000000 ) ) ;
#1324=ADVANCED_FACE ( 'NONE', ( #2364 ), #23223, .T. ) ;
#1328=AXIS2_PLACEMENT_3D ( 'NONE', #32076, #7695, #24061 ) ;
#1329=DIRECTION ( 'NONE',  ( -1.000000000000000000, 0.000000000000000000, 0.000000000000000000 ) ) ;
#1330=ORIENTED_EDGE ( 'NONE', *, *, #22566, .F. ) ;
#1331=DIRECTION ( 'NONE',  ( 0.000000000000000000, 3.374343856708137958E-53, -1.000000000000000000 ) ) ;
#1332=DIRECTION ( 'NONE',  ( 1.000000000000000000, 0.000000000000000000, 0.000000000000000000 ) ) ;
#1334=EDGE_CURVE ( 'NONE', #13964, #33838, #28902, .T. ) ;
#1339=DIRECTION ( 'NONE',  ( 0.000000000000000000, 0.000000000000000000, 1.000000000000000000 ) ) ;
#1340=VERTEX_POINT ( 'NONE', #32088 ) ;
#1342=EDGE_CURVE ( 'NONE', #7970, #11639, #23738, .T. ) ;
#1345=ORIENTED_EDGE ( 'NONE', *, *, #882, .F. ) ;
#1346=ORIENTED_EDGE ( 'NONE', *, *, #16683, .F. ) ;
#1349=CIRCLE ( 'NONE', #21810, 3.999999999999948042 ) ;
#1350=CARTESIAN_POINT ( 'NONE',  ( -418.0000000000000000, -105.0000000000000142, 187.0000000000000000 ) ) ;
#1353=EDGE_LOOP ( 'NONE', ( #34446, #22061, #26302, #9004 ) ) ;
#1354=CARTESIAN_POINT ( 'NONE',  ( -445.9999999999999432, -105.0000000000000142, 162.9999999999999716 ) ) ;
#1355=CARTESIAN_POINT ( 'NONE',  ( -20.00000000000007461, 136.9999999999999432, -190.9999999999999716 ) ) ;
#1358=DIRECTION ( 'NONE',  ( 0.000000000000000000, 0.000000000000000000, 1.000000000000000000 ) ) ;
#1360=CARTESIAN_POINT ( 'NONE',  ( -418.0000000000000000, 105.0000000000000142, 100.0000000000000000 ) ) ;
#1367=EDGE_CURVE ( 'NONE', #30447, #11932, #26058, .T. ) ;
#1369=ORIENTED_EDGE ( 'NONE', *, *, #2507, .F. ) ;
#1372=ORIENTED_EDGE ( 'NONE', *, *, #9870, .F. ) ;
#1373=DIRECTION ( 'NONE',  ( 0.000000000000000000, 0.000000000000000000, -1.000000000000000000 ) ) ;
#1375=VECTOR ( 'NONE', #18478, 1000.000000000000000 ) ;
#1378=DIRECTION ( 'NONE',  ( 1.000000000000000000, 0.000000000000000000, -1.232595164407831220E-32 ) ) ;
#1379=ORIENTED_EDGE ( 'NONE', *, *, #10516, .F. ) ;
#1381=VECTOR ( 'NONE', #8053, 1000.000000000000000 ) ;
#1385=CARTESIAN_POINT ( 'NONE',  ( 15.99999999999998579, 124.9999999999999716, 162.9999999999999716 ) ) ;
#1388=LINE ( 'NONE', #25763, #25846 ) ;
#1393=ORIENTED_EDGE ( 'NONE', *, *, #33177, .F. ) ;
#1394=EDGE_CURVE ( 'NONE', #10216, #12264, #31736, .T. ) ;
#1396=PLANE ( 'NONE',  #30792 ) ;
#1397=DIRECTION ( 'NONE',  ( 3.469446951953832974E-18, 1.000000000000000000, 7.888609052210116302E-31 ) ) ;
#1398=FACE_OUTER_BOUND ( 'NONE', #17490, .T. ) ;
#1399=DIRECTION ( 'NONE',  ( 0.000000000000000000, 0.000000000000000000, 1.000000000000000000 ) ) ;
#1402=VECTOR ( 'NONE', #25282, 1000.000000000000000 ) ;
#1407=DIRECTION ( 'NONE',  ( 0.000000000000000000, 0.000000000000000000, 1.000000000000000000 ) ) ;
#1410=CIRCLE ( 'NONE', #825, 2.000000000000001776 ) ;
#1413=EDGE_CURVE ( 'NONE', #19123, #17691, #15746, .T. ) ;
#1414=DIRECTION ( 'NONE',  ( -1.000000000000000000, 0.000000000000000000, -5.546364386991661285E-52 ) ) ;
#1416=CARTESIAN_POINT ( 'NONE',  ( -442.0000000000000000, -104.9999999999999858, -162.9999999999999716 ) ) ;
#1419=CARTESIAN_POINT ( 'NONE',  ( -349.0000000000000000, -125.0000000000000284, 185.0000000000000000 ) ) ;
#1420=ORIENTED_EDGE ( 'NONE', *, *, #11174, .F. ) ;
#1424=ORIENTED_EDGE ( 'NONE', *, *, #6964, .T. ) ;
#1427=DIRECTION ( 'NONE',  ( 1.000000000000000000, 0.000000000000000000, 0.000000000000000000 ) ) ;
#1430=ORIENTED_EDGE ( 'NONE', *, *, #9780, .F. ) ;
#1432=DIRECTION ( 'NONE',  ( -1.000000000000000000, 0.000000000000000000, -1.300283923313630633E-47 ) ) ;
#1436=ORIENTED_EDGE ( 'NONE', *, *, #15716, .T. ) ;
#1437=DIRECTION ( 'NONE',  ( -1.000000000000000000, -3.469446951953834515E-18, 0.000000000000000000 ) ) ;
#1438=EDGE_CURVE ( 'NONE', #17376, #31755, #29433, .T. ) ;
#1447=EDGE_CURVE ( 'NONE', #11922, #29621, #20724, .T. ) ;
#1448=CIRCLE ( 'NONE', #28152, 3.999999999999976019 ) ;
#1449=FACE_OUTER_BOUND ( 'NONE', #28871, .T. ) ;
#1451=DIRECTION ( 'NONE',  ( 0.000000000000000000, 0.000000000000000000, -1.000000000000000000 ) ) ;
#1456=DIRECTION ( 'NONE',  ( -3.040835319149746528E-31, -1.000000000000000000, 0.000000000000000000 ) ) ;
#1458=ORIENTED_EDGE ( 'NONE', *, *, #6369, .F. ) ;
#1463=EDGE_CURVE ( 'NONE', #1478, #31329, #13244, .T. ) ;
#1469=VERTEX_POINT ( 'NONE', #11098 ) ;
#1471=DIRECTION ( 'NONE',  ( -1.000000000000000000, 0.000000000000000000, 0.000000000000000000 ) ) ;
#1472=VECTOR ( 'NONE', #15375, 1000.000000000000000 ) ;
#1475=DIRECTION ( 'NONE',  ( 1.000000000000000000, 0.000000000000000000, 0.000000000000000000 ) ) ;
#1478=VERTEX_POINT ( 'NONE', #19120 ) ;
#1482=VECTOR ( 'NONE', #26705, 1000.000000000000000 ) ;
#1483=CARTESIAN_POINT ( 'NONE',  ( -19.99999999999998934, 4.559999999999908127, 168.2400000000000091 ) ) ;
#1486=VERTEX_POINT ( 'NONE', #16272 ) ;
#1487=CARTESIAN_POINT ( 'NONE',  ( -12.00000000000001066, 124.9999999999999716, 155.0000000000000000 ) ) ;
#1488=PLANE ( 'NONE',  #19097 ) ;
#1489=CIRCLE ( 'NONE', #19689, 3.999999999999976019 ) ;
#1492=DIRECTION ( 'NONE',  ( 0.000000000000000000, 0.000000000000000000, -1.000000000000000000 ) ) ;
#1496=CARTESIAN_POINT ( 'NONE',  ( -20.00000000000007461, -113.0000000000000000, -162.9999999999999716 ) ) ;
#1498=PLANE ( 'NONE',  #16806 ) ;
#1499=ADVANCED_FACE ( 'NONE', ( #10571 ), #13591, .F. ) ;
#1505=CARTESIAN_POINT ( 'NONE',  ( -19.99999999999998934, -112.9999999999999858, 155.0000000000000000 ) ) ;
#1507=CARTESIAN_POINT ( 'NONE',  ( -20.00000000000001776, -137.0000000000000000, -154.9999999999999716 ) ) ;
#1509=ORIENTED_EDGE ( 'NONE', *, *, #24538, .T. ) ;
#1514=ORIENTED_EDGE ( 'NONE', *, *, #9603, .F. ) ;
#1516=CARTESIAN_POINT ( 'NONE',  ( 19.99999999999998224, -115.0000000000000000, -158.9999999999999716 ) ) ;
#1518=EDGE_CURVE ( 'NONE', #32367, #19566, #21944, .T. ) ;
#1520=ADVANCED_FACE ( 'NONE', ( #29958, #16092 ), #2544, .T. ) ;
#1521=AXIS2_PLACEMENT_3D ( 'NONE', #13047, #32065, #5357 ) ;
#1529=DIRECTION ( 'NONE',  ( -1.292961597001347186E-16, 0.000000000000000000, 1.000000000000000000 ) ) ;
#1531=DIRECTION ( 'NONE',  ( 0.000000000000000000, -7.888609052210118054E-31, -1.000000000000000000 ) ) ;
#1534=DIRECTION ( 'NONE',  ( -0.000000000000000000, -0.000000000000000000, -1.000000000000000000 ) ) ;
#1535=DIRECTION ( 'NONE',  ( 0.000000000000000000, -1.000000000000000000, -2.465190328815662439E-32 ) ) ;
#1538=LINE ( 'NONE', #836, #12071 ) ;
#1539=DIRECTION ( 'NONE',  ( 3.469446951953832974E-18, 1.000000000000000000, -7.888609052210118054E-31 ) ) ;
#1541=ADVANCED_FACE ( 'NONE', ( #9351 ), #11683, .T. ) ;
#1542=EDGE_CURVE ( 'NONE', #423, #15936, #25719, .T. ) ;
#1543=CARTESIAN_POINT ( 'NONE',  ( -349.0000000000000000, 124.9999999999999432, 181.0000000000000000 ) ) ;
#1545=PLANE ( 'NONE',  #20508 ) ;
#1546=EDGE_CURVE ( 'NONE', #29191, #1290, #25361, .T. ) ;
#1549=ORIENTED_EDGE ( 'NONE', *, *, #30645, .F. ) ;
#1550=CYLINDRICAL_SURFACE ( 'NONE', #16030, 3.999999999999976019 ) ;
#1551=CYLINDRICAL_SURFACE ( 'NONE', #7101, 3.999999999999976019 ) ;
#1558=CYLINDRICAL_SURFACE ( 'NONE', #28650, 3.999999999999976019 ) ;
#1562=CIRCLE ( 'NONE', #2694, 7.999999999999979572 ) ;
#1563=DIRECTION ( 'NONE',  ( 0.000000000000000000, 0.000000000000000000, -1.000000000000000000 ) ) ;
#1569=CARTESIAN_POINT ( 'NONE',  ( -499.9999999999999432, -145.0000000000000000, -162.9999999999999716 ) ) ;
#1570=EDGE_CURVE ( 'NONE', #2181, #9401, #22532, .T. ) ;
#1571=CARTESIAN_POINT ( 'NONE',  ( -345.0000000000000000, -125.0000000000000284, 126.0000000000000000 ) ) ;
#1574=LINE ( 'NONE', #28795, #6521 ) ;
#1575=DIRECTION ( 'NONE',  ( 0.000000000000000000, 0.000000000000000000, -1.000000000000000000 ) ) ;
#1576=CARTESIAN_POINT ( 'NONE',  ( -19.99999999999998934, 134.9999999999998863, 187.0000000000000000 ) ) ;
#1578=EDGE_CURVE ( 'NONE', #28711, #30135, #4167, .T. ) ;
#1580=VECTOR ( 'NONE', #9186, 1000.000000000000000 ) ;
#1583=ORIENTED_EDGE ( 'NONE', *, *, #32329, .F. ) ;
#1586=CIRCLE ( 'NONE', #11849, 7.999999999999979572 ) ;
#1588=CARTESIAN_POINT ( 'NONE',  ( -500.0000000000000000, -137.0000000000000000, 155.0000000000000000 ) ) ;
#1591=ORIENTED_EDGE ( 'NONE', *, *, #33237, .T. ) ;
#1592=CIRCLE ( 'NONE', #13512, 7.999999999999979572 ) ;
#1594=VERTEX_POINT ( 'NONE', #9691 ) ;
#1601=EDGE_CURVE ( 'NONE', #14586, #5645, #7354, .T. ) ;
#1605=DIRECTION ( 'NONE',  ( -0.000000000000000000, 1.000000000000000000, -0.000000000000000000 ) ) ;
#1608=ORIENTED_EDGE ( 'NONE', *, *, #29083, .F. ) ;
#1610=LINE ( 'NONE', #4267, #18005 ) ;
#1611=DIRECTION ( 'NONE',  ( -1.300283923313630633E-47, 0.000000000000000000, 1.000000000000000000 ) ) ;
#1612=FACE_OUTER_BOUND ( 'NONE', #15707, .T. ) ;
#1614=DIRECTION ( 'NONE',  ( -0.000000000000000000, -1.000000000000000000, -0.000000000000000000 ) ) ;
#1618=CARTESIAN_POINT ( 'NONE',  ( 15.99999999999997868, -145.0000000000000000, -186.9999999999999716 ) ) ;
#1622=FACE_OUTER_BOUND ( 'NONE', #15105, .T. ) ;
#1625=DIRECTION ( 'NONE',  ( -5.546364386991661285E-52, 0.000000000000000000, -1.000000000000000000 ) ) ;
#1627=CARTESIAN_POINT ( 'NONE',  ( -499.9999999999999432, -145.0000000000000000, -187.0000000000000000 ) ) ;
#1631=ORIENTED_EDGE ( 'NONE', *, *, #12031, .F. ) ;
#1634=MECHANICAL_DESIGN_GEOMETRIC_PRESENTATION_REPRESENTATION('',(#21543),#23797);
#1642=CIRCLE ( 'NONE', #33458, 4.000000000000003553 ) ;
#1644=ORIENTED_EDGE ( 'NONE', *, *, #4995, .F. ) ;
#1646=DIRECTION ( 'NONE',  ( 0.000000000000000000, 1.000000000000000000, 3.374343856708137958E-53 ) ) ;
#1653=LINE ( 'NONE', #31040, #5724 ) ;
#1657=PLANE ( 'NONE',  #11701 ) ;
#1665=DIRECTION ( 'NONE',  ( 1.000000000000000000, 0.000000000000000000, 0.000000000000000000 ) ) ;
#1670=CARTESIAN_POINT ( 'NONE',  ( 19.99999999999998934, -137.0000000000000000, 155.0000000000000000 ) ) ;
#1672=CARTESIAN_POINT ( 'NONE',  ( -414.0000000000000568, 124.9999999999999432, -162.9999999999999716 ) ) ;
#1673=AXIS2_PLACEMENT_3D ( 'NONE', #6817, #34409, #17706 ) ;
#1675=DIRECTION ( 'NONE',  ( 1.000000000000000000, 3.469446951953834515E-18, 0.000000000000000000 ) ) ;
#1677=EDGE_CURVE ( 'NONE', #5400, #14586, #12828, .T. ) ;
#1679=APPLICATION_CONTEXT ( 'automotive_design' ) ;
#1680=ORIENTED_EDGE ( 'NONE', *, *, #10734, .F. ) ;
#1683=VERTEX_POINT ( 'NONE', #4679 ) ;
#1685=DIRECTION ( 'NONE',  ( 0.000000000000000000, 1.000000000000000000, 5.053935297177146739E-49 ) ) ;
#1687=CARTESIAN_POINT ( 'NONE',  ( -20.00000000000007461, 136.9999999999999432, 162.9999999999999716 ) ) ;
#1688=DIRECTION ( 'NONE',  ( 0.000000000000000000, -5.053935297177146739E-49, -1.000000000000000000 ) ) ;
#1689=EDGE_CURVE ( 'NONE', #15148, #19084, #5353, .T. ) ;
#1690=EDGE_LOOP ( 'NONE', ( #7739, #345, #3044, #15845 ) ) ;
#1691=EDGE_CURVE ( 'NONE', #9401, #23007, #20725, .T. ) ;
#1692=ORIENTED_EDGE ( 'NONE', *, *, #27472, .F. ) ;
#1693=DIRECTION ( 'NONE',  ( 0.000000000000000000, 0.000000000000000000, 1.000000000000000000 ) ) ;
#1694=CARTESIAN_POINT ( 'NONE',  ( 11.99999999999995559, -145.0000000000000000, 187.0000000000000000 ) ) ;
#1695=DIRECTION ( 'NONE',  ( -5.546364386991661285E-52, 0.000000000000000000, -1.000000000000000000 ) ) ;
#1697=CARTESIAN_POINT ( 'NONE',  ( -442.0000000000000000, 124.9999999999999574, -194.9999999999999716 ) ) ;
#1698=CARTESIAN_POINT ( 'NONE',  ( -442.0000000000000000, -137.0000000000000000, -155.0000000000000000 ) ) ;
#1699=ORIENTED_EDGE ( 'NONE', *, *, #11310, .F. ) ;
#1707=EDGE_CURVE ( 'NONE', #9925, #10965, #18424, .T. ) ;
#1709=EDGE_LOOP ( 'NONE', ( #8360, #692, #21365, #8682, #1372, #28525, #28831, #21209 ) ) ;
#1713=CARTESIAN_POINT ( 'NONE',  ( -20.00000000000007461, -113.0000000000000000, -190.9999999999999716 ) ) ;
#1714=CARTESIAN_POINT ( 'NONE',  ( -499.9999999999999432, 144.9999999999999716, 187.0000000000000000 ) ) ;
#1717=CARTESIAN_POINT ( 'NONE',  ( -445.9999999999999432, -125.0000000000000000, 162.9999999999999716 ) ) ;
#1718=LINE ( 'NONE', #10084, #33852 ) ;
#1719=EDGE_LOOP ( 'NONE', ( #29333, #7728, #12429, #25576 ) ) ;
#1720=CIRCLE ( 'NONE', #8530, 7.999999999999979572 ) ;
#1724=ORIENTED_EDGE ( 'NONE', *, *, #30385, .T. ) ;
#1725=CARTESIAN_POINT ( 'NONE',  ( -499.9999999999999432, -113.0000000000000000, -159.0000000000000000 ) ) ;
#1726=DIRECTION ( 'NONE',  ( 1.000000000000000000, 0.000000000000000000, 0.000000000000000000 ) ) ;
#1728=VECTOR ( 'NONE', #27829, 1000.000000000000000 ) ;
#1729=DIRECTION ( 'NONE',  ( -1.000000000000000000, 0.000000000000000000, 0.000000000000000000 ) ) ;
#1733=ADVANCED_FACE ( 'NONE', ( #34963, #26940 ), #5393, .T. ) ;
#1734=ORIENTED_EDGE ( 'NONE', *, *, #18176, .F. ) ;
#1735=ORIENTED_EDGE ( 'NONE', *, *, #12554, .F. ) ;
#1736=DIRECTION ( 'NONE',  ( 1.000000000000000000, 3.469446951953834515E-18, 0.000000000000000000 ) ) ;
#1738=CARTESIAN_POINT ( 'NONE',  ( 19.99999999999998934, -55.00000000000000711, 154.9999999999999716 ) ) ;
#1739=DIRECTION ( 'NONE',  ( 0.000000000000000000, 0.000000000000000000, -1.000000000000000000 ) ) ;
#1743=AXIS2_PLACEMENT_3D ( 'NONE', #32287, #22148, #16647 ) ;
#1745=CARTESIAN_POINT ( 'NONE',  ( -414.0000000000000568, 113.0000000000000000, -155.0000000000000000 ) ) ;
#1746=ADVANCED_FACE ( 'NONE', ( #3255 ), #24605, .F. ) ;
#1750=DIRECTION ( 'NONE',  ( 1.000000000000000000, 0.000000000000000000, 0.000000000000000000 ) ) ;
#1751=EDGE_CURVE ( 'NONE', #23608, #11201, #16457, .T. ) ;
#1757=DIRECTION ( 'NONE',  ( 0.000000000000000000, 1.000000000000000000, 5.145227585319922065E-49 ) ) ;
#1760=FACE_BOUND ( 'NONE', #2139, .T. ) ;
#1763=ORIENTED_EDGE ( 'NONE', *, *, #31218, .T. ) ;
#1765=ORIENTED_EDGE ( 'NONE', *, *, #4038, .T. ) ;
#1780=VERTEX_POINT ( 'NONE', #2894 ) ;
#1783=CARTESIAN_POINT ( 'NONE',  ( 11.99999999999999645, -124.9999999999999432, -154.9999999999999716 ) ) ;
#1784=ORIENTED_EDGE ( 'NONE', *, *, #18783, .F. ) ;
#1787=CARTESIAN_POINT ( 'NONE',  ( 11.99999999999999645, 144.9999999999999147, 155.0000000000000000 ) ) ;
#1794=ADVANCED_FACE ( 'NONE', ( #27110 ), #24791, .T. ) ;
#1796=CARTESIAN_POINT ( 'NONE',  ( -418.0000000000000000, -124.9999999999999858, -73.99999999999998579 ) ) ;
#1800=AXIS2_PLACEMENT_3D ( 'NONE', #12982, #7969, #16185 ) ;
#1802=AXIS2_PLACEMENT_3D ( 'NONE', #23257, #14557, #11885 ) ;
#1803=AXIS2_PLACEMENT_3D ( 'NONE', #25568, #28253, #22915 ) ;
#1804=VECTOR ( 'NONE', #19250, 1000.000000000000000 ) ;
#1810=ORIENTED_EDGE ( 'NONE', *, *, #7138, .F. ) ;
#1811=ORIENTED_EDGE ( 'NONE', *, *, #24121, .F. ) ;
#1812=VERTEX_POINT ( 'NONE', #8243 ) ;
#1814=ORIENTED_EDGE ( 'NONE', *, *, #8906, .F. ) ;
#1816=CARTESIAN_POINT ( 'NONE',  ( -418.0000000000000000, -125.0000000000000000, 194.9999999999999716 ) ) ;
#1817=ORIENTED_EDGE ( 'NONE', *, *, #6051, .F. ) ;
#1818=ORIENTED_EDGE ( 'NONE', *, *, #9423, .F. ) ;
#1819=LINE ( 'NONE', #12700, #27634 ) ;
#1820=DIRECTION ( 'NONE',  ( 0.000000000000000000, -1.000000000000000000, 3.421138828918010427E-49 ) ) ;
#1826=DIRECTION ( 'NONE',  ( 0.000000000000000000, -1.000000000000000000, 0.000000000000000000 ) ) ;
#1827=DIRECTION ( 'NONE',  ( 0.000000000000000000, -1.000000000000000000, 6.123233995736766036E-17 ) ) ;
#1830=ORIENTED_EDGE ( 'NONE', *, *, #3032, .T. ) ;
#1831=VECTOR ( 'NONE', #8844, 1000.000000000000000 ) ;
#1834=LINE ( 'NONE', #13234, #29745 ) ;
#1836=CARTESIAN_POINT ( 'NONE',  ( -414.0000000000000568, -125.0000000000000000, 107.9999999999999858 ) ) ;
#1838=ADVANCED_FACE ( 'NONE', ( #30133 ), #16631, .T. ) ;
#1841=EDGE_CURVE ( 'NONE', #5027, #30076, #11284, .T. ) ;
#1842=DIRECTION ( 'NONE',  ( 0.000000000000000000, -1.000000000000000000, -2.465190328815662439E-32 ) ) ;
#1844=CYLINDRICAL_SURFACE ( 'NONE', #396, 7.999999999999979572 ) ;
#1848=VERTEX_POINT ( 'NONE', #30841 ) ;
#1849=AXIS2_PLACEMENT_3D ( 'NONE', #21766, #21427, #13769 ) ;
#1850=CIRCLE ( 'NONE', #21749, 7.999999999999979572 ) ;
#1856=DIRECTION ( 'NONE',  ( 0.000000000000000000, -1.000000000000000000, -0.000000000000000000 ) ) ;
#1858=DIRECTION ( 'NONE',  ( -1.000000000000000000, 0.000000000000000000, 0.000000000000000000 ) ) ;
#1859=ORIENTED_EDGE ( 'NONE', *, *, #23919, .F. ) ;
#1860=ORIENTED_EDGE ( 'NONE', *, *, #33232, .F. ) ;
#1861=CARTESIAN_POINT ( 'NONE',  ( -20.00000000000007461, 136.9999999999999432, 194.9999999999999716 ) ) ;
#1862=CARTESIAN_POINT ( 'NONE',  ( 11.99999999999999645, -55.00000000000000711, 162.9999999999999716 ) ) ;
#1864=CARTESIAN_POINT ( 'NONE',  ( -19.99999999999998934, -105.0000000000000142, 162.9999999999999716 ) ) ;
#1865=FACE_OUTER_BOUND ( 'NONE', #3125, .T. ) ;
#1866=ORIENTED_EDGE ( 'NONE', *, *, #9937, .F. ) ;
#1875=CARTESIAN_POINT ( 'NONE',  ( -418.0000000000000000, 109.0000000000000142, -175.0000000000000000 ) ) ;
#1885=ORIENTED_EDGE ( 'NONE', *, *, #15153, .F. ) ;
#1891=CIRCLE ( 'NONE', #29164, 7.999999999999979572 ) ;
#1893=VERTEX_POINT ( 'NONE', #948 ) ;
#1898=DIRECTION ( 'NONE',  ( 0.000000000000000000, 0.000000000000000000, -1.000000000000000000 ) ) ;
#1899=AXIS2_PLACEMENT_3D ( 'NONE', #12201, #34064, #30525 ) ;
#1900=DIRECTION ( 'NONE',  ( 0.000000000000000000, 1.310824597558155437E-49, 1.000000000000000000 ) ) ;
#1905=VECTOR ( 'NONE', #15165, 1000.000000000000000 ) ;
#1907=DIRECTION ( 'NONE',  ( -5.546364386991661285E-52, 0.000000000000000000, 1.000000000000000000 ) ) ;
#1911=CARTESIAN_POINT ( 'NONE',  ( -12.00000000000001066, -60.99999999999997158, 154.9999999999999716 ) ) ;
#1912=( NAMED_UNIT ( * ) PLANE_ANGLE_UNIT ( ) SI_UNIT ( $, .RADIAN. ) );
#1913=ORIENTED_EDGE ( 'NONE', *, *, #29312, .T. ) ;
#1914=FACE_OUTER_BOUND ( 'NONE', #15328, .T. ) ;
#1915=LINE ( 'NONE', #23642, #16620 ) ;
#1916=CYLINDRICAL_SURFACE ( 'NONE', #17762, 2.000000000000001776 ) ;
#1917=VERTEX_POINT ( 'NONE', #17343 ) ;
#1919=CARTESIAN_POINT ( 'NONE',  ( -20.00000000000001776, -109.0000000000000142, 187.0000000000000000 ) ) ;
#1921=LINE ( 'NONE', #34144, #2363 ) ;
#1923=DIRECTION ( 'NONE',  ( 0.000000000000000000, -5.145227585319922065E-49, -1.000000000000000000 ) ) ;
#1927=EDGE_CURVE ( 'NONE', #29708, #30081, #11821, .T. ) ;
#1928=CIRCLE ( 'NONE', #7613, 3.999999999999976019 ) ;
#1932=AXIS2_PLACEMENT_3D ( 'NONE', #2031, #21071, #12909 ) ;
#1933=EDGE_LOOP ( 'NONE', ( #3858, #9699, #27243, #315 ) ) ;
#1938=EDGE_CURVE ( 'NONE', #5864, #27222, #9959, .T. ) ;
#1944=VERTEX_POINT ( 'NONE', #16991 ) ;
#1948=ORIENTED_EDGE ( 'NONE', *, *, #31263, .F. ) ;
#1950=LINE ( 'NONE', #14801, #10474 ) ;
#1952=EDGE_CURVE ( 'NONE', #32238, #7140, #20145, .T. ) ;
#1953=ORIENTED_EDGE ( 'NONE', *, *, #9611, .T. ) ;
#1958=VECTOR ( 'NONE', #30308, 1000.000000000000000 ) ;
#1960=DIRECTION ( 'NONE',  ( 0.000000000000000000, 5.053935297177146739E-49, 1.000000000000000000 ) ) ;
#1970=CIRCLE ( 'NONE', #33813, 7.999999999999979572 ) ;
#1975=DIRECTION ( 'NONE',  ( 0.000000000000000000, 0.000000000000000000, -1.000000000000000000 ) ) ;
#1977=AXIS2_PLACEMENT_3D ( 'NONE', #17267, #14592, #22231 ) ;
#1979=AXIS2_PLACEMENT_3D ( 'NONE', #25827, #34190, #22993 ) ;
#1980=ORIENTED_EDGE ( 'NONE', *, *, #27672, .T. ) ;
#1981=AXIS2_PLACEMENT_3D ( 'NONE', #3376, #20293, #6747 ) ;
#1983=ORIENTED_EDGE ( 'NONE', *, *, #4996, .T. ) ;
#1986=ORIENTED_EDGE ( 'NONE', *, *, #5359, .T. ) ;
#1988=ORIENTED_EDGE ( 'NONE', *, *, #29206, .F. ) ;
#1992=ADVANCED_FACE ( 'NONE', ( #7270 ), #25133, .T. ) ;
#1996=DIRECTION ( 'NONE',  ( 0.000000000000000000, -0.000000000000000000, -1.000000000000000000 ) ) ;
#1999=DIRECTION ( 'NONE',  ( -1.000000000000000000, 0.000000000000000000, 0.000000000000000000 ) ) ;
#2000=AXIS2_PLACEMENT_3D ( 'NONE', #20065, #34275, #9891 ) ;
#2006=DIRECTION ( 'NONE',  ( -1.000000000000000000, 0.000000000000000000, -5.546364386991661285E-52 ) ) ;
#2010=ADVANCED_FACE ( 'NONE', ( #17162 ), #12824, .F. ) ;
#2012=CLOSED_SHELL ( 'NONE', ( #34325, #26112, #26388, #31073, #14924, #33339, #520, #9363, #1520, #23091, #13003, #18943, #31759, #33948, #20338, #28285, #26628, #15262 ) ) ;
#2014=LINE ( 'NONE', #13059, #20110 ) ;
#2020=ORIENTED_EDGE ( 'NONE', *, *, #34727, .T. ) ;
#2029=ORIENTED_EDGE ( 'NONE', *, *, #6051, .T. ) ;
#2030=ORIENTED_EDGE ( 'NONE', *, *, #10622, .T. ) ;
#2031=CARTESIAN_POINT ( 'NONE',  ( -12.00000000000001066, -137.0000000000000000, -155.0000000000000284 ) ) ;
#2032=VERTEX_POINT ( 'NONE', #32012 ) ;
#2034=DIRECTION ( 'NONE',  ( -5.546364386991661285E-52, 0.000000000000000000, -1.000000000000000000 ) ) ;
#2038=CIRCLE ( 'NONE', #10022, 7.999999999999979572 ) ;
#2040=FACE_OUTER_BOUND ( 'NONE', #35068, .T. ) ;
#2043=VERTEX_POINT ( 'NONE', #34883 ) ;
#2048=PLANE ( 'NONE',  #630 ) ;
#2050=ORIENTED_EDGE ( 'NONE', *, *, #31346, .T. ) ;
#2052=VECTOR ( 'NONE', #32977, 1000.000000000000000 ) ;
#2053=DIRECTION ( 'NONE',  ( 0.000000000000000000, -1.000000000000000000, -2.309213040847544338E-50 ) ) ;
#2054=LINE ( 'NONE', #34449, #3922 ) ;
#2055=EDGE_LOOP ( 'NONE', ( #30550, #34729, #25241, #13654 ) ) ;
#2057=DIRECTION ( 'NONE',  ( 1.000000000000000000, 0.000000000000000000, -0.000000000000000000 ) ) ;
#2059=FACE_OUTER_BOUND ( 'NONE', #6196, .T. ) ;
#2060=ORIENTED_EDGE ( 'NONE', *, *, #14332, .F. ) ;
#2064=ORIENTED_EDGE ( 'NONE', *, *, #25749, .F. ) ;
#2065=CARTESIAN_POINT ( 'NONE',  ( -500.0000000000000000, -109.0000000000000142, 162.9999999999999716 ) ) ;
#2066=LINE ( 'NONE', #12581, #3177 ) ;
#2068=ORIENTED_EDGE ( 'NONE', *, *, #12031, .T. ) ;
#2070=CARTESIAN_POINT ( 'NONE',  ( 11.99999999999999645, -137.0000000000000000, 155.0000000000000000 ) ) ;
#2072=VECTOR ( 'NONE', #26157, 1000.000000000000000 ) ;
#2075=ORIENTED_EDGE ( 'NONE', *, *, #29949, .F. ) ;
#2076=DIRECTION ( 'NONE',  ( 0.000000000000000000, 0.000000000000000000, 1.000000000000000000 ) ) ;
#2077=ORIENTED_EDGE ( 'NONE', *, *, #10363, .F. ) ;
#2079=CYLINDRICAL_SURFACE ( 'NONE', #24675, 4.750000000000004441 ) ;
#2080=ADVANCED_FACE ( 'NONE', ( #2647 ), #4955, .F. ) ;
#2081=CARTESIAN_POINT ( 'NONE',  ( -361.0000000000000000, -125.0000000000000284, 164.9999999999999716 ) ) ;
#2083=EDGE_CURVE ( 'NONE', #2208, #15011, #18447, .T. ) ;
#2087=ORIENTED_EDGE ( 'NONE', *, *, #26225, .T. ) ;
#2088=VERTEX_POINT ( 'NONE', #7978 ) ;
#2090=DIRECTION ( 'NONE',  ( 0.000000000000000000, 0.000000000000000000, -1.000000000000000000 ) ) ;
#2091=VECTOR ( 'NONE', #12539, 1000.000000000000000 ) ;
#2092=CARTESIAN_POINT ( 'NONE',  ( 15.99999999999998579, 4.559999999999909015, -168.2400000000000091 ) ) ;
#2094=PLANE ( 'NONE',  #104 ) ;
#2095=DIRECTION ( 'NONE',  ( 0.000000000000000000, -1.000000000000000000, 0.000000000000000000 ) ) ;
#2103=DIRECTION ( 'NONE',  ( 0.000000000000000000, 2.309213040847544338E-50, 1.000000000000000000 ) ) ;
#2105=CIRCLE ( 'NONE', #10052, 7.999999999999979572 ) ;
#2106=CARTESIAN_POINT ( 'NONE',  ( 15.99999999999998579, -124.9999999999999432, -186.9999999999999716 ) ) ;
#2111=DIRECTION ( 'NONE',  ( 1.000000000000000000, 3.469446951953834515E-18, 0.000000000000000000 ) ) ;
#2112=CARTESIAN_POINT ( 'NONE',  ( -499.9999999999999432, 112.9999999999999574, -162.9999999999999716 ) ) ;
#2120=VECTOR ( 'NONE', #21830, 1000.000000000000000 ) ;
#2121=AXIS2_PLACEMENT_3D ( 'NONE', #8045, #23887, #24240 ) ;
#2124=ORIENTED_EDGE ( 'NONE', *, *, #24437, .T. ) ;
#2125=EDGE_CURVE ( 'NONE', #17537, #5382, #32535, .T. ) ;
#2126=LINE ( 'NONE', #3647, #6152 ) ;
#2128=AXIS2_PLACEMENT_3D ( 'NONE', #4393, #12961, #1736 ) ;
#2131=ORIENTED_EDGE ( 'NONE', *, *, #19818, .T. ) ;
#2132=EDGE_LOOP ( 'NONE', ( #22132, #26725, #26763, #30796, #23754, #18166, #9844, #10548, #18223 ) ) ;
#2133=EDGE_CURVE ( 'NONE', #26553, #30412, #7059, .T. ) ;
#2134=EDGE_CURVE ( 'NONE', #20509, #30714, #33214, .T. ) ;
#2138=CARTESIAN_POINT ( 'NONE',  ( -441.9999999999999432, -105.0000000000000142, 135.9999999999999716 ) ) ;
#2139=EDGE_LOOP ( 'NONE', ( #20851, #13081, #25315, #33907, #19387, #18939, #11786, #25534 ) ) ;
#2144=DIRECTION ( 'NONE',  ( -8.433758354584418579E-81, 1.000000000000000000, 3.421138828918010427E-49 ) ) ;
#2148=CARTESIAN_POINT ( 'NONE',  ( -442.0000000000000000, -125.0000000000000000, 155.0000000000000000 ) ) ;
#2160=EDGE_LOOP ( 'NONE', ( #17517, #12192, #1027, #11996 ) ) ;
#2161=VERTEX_POINT ( 'NONE', #16902 ) ;
#2165=EDGE_LOOP ( 'NONE', ( #25285, #8276, #2405, #3867 ) ) ;
#2167=DIRECTION ( 'NONE',  ( 1.000000000000000000, 0.000000000000000000, -0.000000000000000000 ) ) ;
#2171=DIRECTION ( 'NONE',  ( -0.000000000000000000, 1.000000000000000000, -0.000000000000000000 ) ) ;
#2173=ORIENTED_EDGE ( 'NONE', *, *, #3208, .T. ) ;
#2176=CARTESIAN_POINT ( 'NONE',  ( 11.99999999999999645, 140.9999999999999716, -175.0000000000000284 ) ) ;
#2178=DIRECTION ( 'NONE',  ( -1.000000000000000000, 0.000000000000000000, 0.000000000000000000 ) ) ;
#2179=CARTESIAN_POINT ( 'NONE',  ( -442.0000000000000000, 105.0000000000000142, 100.0000000000000000 ) ) ;
#2180=DIRECTION ( 'NONE',  ( 0.000000000000000000, 1.131431318426415506E-52, 1.000000000000000000 ) ) ;
#2181=VERTEX_POINT ( 'NONE', #29884 ) ;
#2185=CARTESIAN_POINT ( 'NONE',  ( -345.0000000000000000, -125.0000000000000284, 126.0000000000000000 ) ) ;
#2188=CARTESIAN_POINT ( 'NONE',  ( -20.00000000000007461, 112.9999999999999574, 159.0000000000000000 ) ) ;
#2189=DIRECTION ( 'NONE',  ( 0.000000000000000000, 0.000000000000000000, 1.000000000000000000 ) ) ;
#2193=CYLINDRICAL_SURFACE ( 'NONE', #11633, 3.999999999999976019 ) ;
#2195=FACE_OUTER_BOUND ( 'NONE', #19836, .T. ) ;
#2197=EDGE_CURVE ( 'NONE', #6435, #26862, #5936, .T. ) ;
#2200=DIRECTION ( 'NONE',  ( 0.000000000000000000, 0.000000000000000000, 1.000000000000000000 ) ) ;
#2205=EDGE_CURVE ( 'NONE', #15586, #8663, #6504, .T. ) ;
#2208=VERTEX_POINT ( 'NONE', #33062 ) ;
#2210=FACE_BOUND ( 'NONE', #20490, .T. ) ;
#2213=DIRECTION ( 'NONE',  ( -1.000000000000000000, 0.000000000000000000, 0.000000000000000000 ) ) ;
#2214=VERTEX_POINT ( 'NONE', #22221 ) ;
#2215=ORIENTED_EDGE ( 'NONE', *, *, #2461, .F. ) ;
#2219=CARTESIAN_POINT ( 'NONE',  ( 15.99999999999998579, 112.9999999999999574, -175.0000000000000284 ) ) ;
#2223=DIRECTION ( 'NONE',  ( -0.000000000000000000, 1.000000000000000000, -0.000000000000000000 ) ) ;
#2225=ORIENTED_EDGE ( 'NONE', *, *, #7608, .T. ) ;
#2227=DIRECTION ( 'NONE',  ( 3.040835319149746090E-31, 1.000000000000000000, 0.000000000000000000 ) ) ;
#2233=CARTESIAN_POINT ( 'NONE',  ( -418.0000000000000000, -124.9999999999999716, 139.9999999999999716 ) ) ;
#2235=DIRECTION ( 'NONE',  ( 1.000000000000000000, -0.000000000000000000, -0.000000000000000000 ) ) ;
#2239=EDGE_CURVE ( 'NONE', #18709, #27398, #3345, .T. ) ;
#2246=ORIENTED_EDGE ( 'NONE', *, *, #26521, .T. ) ;
#2248=ORIENTED_EDGE ( 'NONE', *, *, #8887, .F. ) ;
#2249=CARTESIAN_POINT ( 'NONE',  ( -445.9999999999999432, 137.0000000000000000, -175.0000000000000000 ) ) ;
#2253=CYLINDRICAL_SURFACE ( 'NONE', #13690, 7.999999999999979572 ) ;
#2254=VERTEX_POINT ( 'NONE', #21863 ) ;
#2257=DIRECTION ( 'NONE',  ( -1.000000000000000000, 0.000000000000000000, 0.000000000000000000 ) ) ;
#2259=CARTESIAN_POINT ( 'NONE',  ( -418.0000000000000000, -141.0000000000000000, 154.9999999999999716 ) ) ;
#2261=PLANE ( 'NONE',  #2939 ) ;
#2262=LINE ( 'NONE', #13136, #15790 ) ;
#2265=LINE ( 'NONE', #8133, #24224 ) ;
#2271=DIRECTION ( 'NONE',  ( 0.000000000000000000, 1.000000000000000000, 0.000000000000000000 ) ) ;
#2273=FACE_OUTER_BOUND ( 'NONE', #27988, .T. ) ;
#2275=EDGE_CURVE ( 'NONE', #19944, #30605, #32892, .T. ) ;
#2276=ORIENTED_EDGE ( 'NONE', *, *, #10213, .T. ) ;
#2280=ADVANCED_FACE ( 'NONE', ( #25047, #33251 ), #5649, .T. ) ;
#2281=ORIENTED_EDGE ( 'NONE', *, *, #25267, .T. ) ;
#2286=DIRECTION ( 'NONE',  ( 0.000000000000000000, 0.000000000000000000, -1.000000000000000000 ) ) ;
#2291=CARTESIAN_POINT ( 'NONE',  ( -442.0000000000000000, 124.9999999999999432, -162.9999999999999716 ) ) ;
#2292=AXIS2_PLACEMENT_3D ( 'NONE', #17440, #20269, #11548 ) ;
#2294=DIRECTION ( 'NONE',  ( 1.000000000000000000, 0.000000000000000000, 0.000000000000000000 ) ) ;
#2297=CARTESIAN_POINT ( 'NONE',  ( -449.9999999999999432, -105.0000000000000142, -174.9999999999999716 ) ) ;
#2300=DIRECTION ( 'NONE',  ( 0.000000000000000000, 1.000000000000000000, 2.465190328815662439E-32 ) ) ;
#2301=ORIENTED_EDGE ( 'NONE', *, *, #21912, .F. ) ;
#2304=VECTOR ( 'NONE', #5071, 1000.000000000000000 ) ;
#2306=ORIENTED_EDGE ( 'NONE', *, *, #2507, .T. ) ;
#2310=DIRECTION ( 'NONE',  ( 0.000000000000000000, 1.000000000000000000, -3.374343856708137958E-53 ) ) ;
#2312=FACE_OUTER_BOUND ( 'NONE', #4217, .T. ) ;
#2315=AXIS2_PLACEMENT_3D ( 'NONE', #13091, #31932, #28752 ) ;
#2318=ADVANCED_FACE ( 'NONE', ( #30223 ), #12261, .F. ) ;
#2319=VECTOR ( 'NONE', #16286, 1000.000000000000000 ) ;
#2320=VERTEX_POINT ( 'NONE', #22755 ) ;
#2322=EDGE_CURVE ( 'NONE', #11932, #10023, #1388, .T. ) ;
#2326=EDGE_CURVE ( 'NONE', #34521, #2181, #27545, .T. ) ;
#2327=VECTOR ( 'NONE', #11791, 1000.000000000000000 ) ;
#2333=CIRCLE ( 'NONE', #11444, 7.999999999999979572 ) ;
#2338=ORIENTED_EDGE ( 'NONE', *, *, #3646, .F. ) ;
#2347=VECTOR ( 'NONE', #33690, 1000.000000000000000 ) ;
#2349=DIRECTION ( 'NONE',  ( 3.469446951953832974E-18, 1.000000000000000000, -7.888609052210118054E-31 ) ) ;
#2353=PLANE ( 'NONE',  #8708 ) ;
#2354=CARTESIAN_POINT ( 'NONE',  ( 11.99999999999999645, -109.0000000000000142, 174.9999999999999432 ) ) ;
#2358=VECTOR ( 'NONE', #8325, 1000.000000000000000 ) ;
#2361=ORIENTED_EDGE ( 'NONE', *, *, #23316, .F. ) ;
#2363=VECTOR ( 'NONE', #7257, 1000.000000000000000 ) ;
#2364=FACE_OUTER_BOUND ( 'NONE', #5108, .T. ) ;
#2365=EDGE_CURVE ( 'NONE', #23877, #12319, #23112, .T. ) ;
#2366=ORIENTED_EDGE ( 'NONE', *, *, #17822, .F. ) ;
#2367=EDGE_CURVE ( 'NONE', #7970, #14594, #30963, .T. ) ;
#2370=VERTEX_POINT ( 'NONE', #31116 ) ;
#2372=ORIENTED_EDGE ( 'NONE', *, *, #25340, .F. ) ;
#2377=EDGE_CURVE ( 'NONE', #25411, #173, #14928, .T. ) ;
#2380=DIRECTION ( 'NONE',  ( 0.000000000000000000, 0.000000000000000000, 1.000000000000000000 ) ) ;
#2383=CARTESIAN_POINT ( 'NONE',  ( -418.0000000000000000, 105.0000000000000000, -77.99999999999997158 ) ) ;
#2387=DIRECTION ( 'NONE',  ( 0.000000000000000000, 0.000000000000000000, 1.000000000000000000 ) ) ;
#2389=EDGE_LOOP ( 'NONE', ( #23753, #18036, #25360, #34828 ) ) ;
#2391=EDGE_CURVE ( 'NONE', #35, #29789, #12600, .T. ) ;
#2392=CARTESIAN_POINT ( 'NONE',  ( -19.99999999999998934, -145.0000000000000000, 162.9999999999999716 ) ) ;
#2393=CARTESIAN_POINT ( 'NONE',  ( -418.0000000000000000, -145.0000000000000000, -175.0000000000000000 ) ) ;
#2395=CARTESIAN_POINT ( 'NONE',  ( -499.9999999999999432, 140.9999999999999716, 187.0000000000000000 ) ) ;
#2398=FACE_OUTER_BOUND ( 'NONE', #27764, .T. ) ;
#2400=CARTESIAN_POINT ( 'NONE',  ( -500.0000000000000000, -105.0000000000000142, 194.9999999999999716 ) ) ;
#2405=ORIENTED_EDGE ( 'NONE', *, *, #25499, .T. ) ;
#2406=DIRECTION ( 'NONE',  ( -1.000000000000000000, 0.000000000000000000, 0.000000000000000000 ) ) ;
#2409=AXIS2_PLACEMENT_3D ( 'NONE', #19586, #33271, #9068 ) ;
#2410=ORIENTED_EDGE ( 'NONE', *, *, #19984, .F. ) ;
#2411=AXIS2_PLACEMENT_3D ( 'NONE', #17555, #1332, #12204 ) ;
#2413=AXIS2_PLACEMENT_3D ( 'NONE', #31258, #6515, #6859 ) ;
#2416=ORIENTED_EDGE ( 'NONE', *, *, #8034, .T. ) ;
#2418=ORIENTED_EDGE ( 'NONE', *, *, #3028, .F. ) ;
#2420=ORIENTED_EDGE ( 'NONE', *, *, #15759, .T. ) ;
#2426=ORIENTED_EDGE ( 'NONE', *, *, #11147, .T. ) ;
#2429=CARTESIAN_POINT ( 'NONE',  ( -445.9999999999999432, 124.9999999999999432, -162.9999999999999716 ) ) ;
#2433=FACE_OUTER_BOUND ( 'NONE', #21921, .T. ) ;
#2435=VECTOR ( 'NONE', #15082, 1000.000000000000000 ) ;
#2436=DIRECTION ( 'NONE',  ( -1.000000000000000000, 0.000000000000000000, 0.000000000000000000 ) ) ;
#2438=CARTESIAN_POINT ( 'NONE',  ( 11.99999999999999645, -124.9999999999999432, -186.9999999999999716 ) ) ;
#2442=CARTESIAN_POINT ( 'NONE',  ( -442.0000000000000000, -112.9999999999999858, 155.0000000000000000 ) ) ;
#2443=VERTEX_POINT ( 'NONE', #22927 ) ;
#2444=EDGE_CURVE ( 'NONE', #7133, #7970, #6542, .T. ) ;
#2445=CARTESIAN_POINT ( 'NONE',  ( -15.99999999999998579, -137.0000000000000000, 155.0000000000000000 ) ) ;
#2448=FACE_OUTER_BOUND ( 'NONE', #18477, .T. ) ;
#2450=ORIENTED_EDGE ( 'NONE', *, *, #5372, .T. ) ;
#2451=CARTESIAN_POINT ( 'NONE',  ( -12.00000000000001066, 112.9999999999999574, -155.0000000000000000 ) ) ;
#2457=CIRCLE ( 'NONE', #22338, 7.999999999999992895 ) ;
#2461=EDGE_CURVE ( 'NONE', #32511, #18108, #21126, .T. ) ;
#2462=ORIENTED_EDGE ( 'NONE', *, *, #14480, .F. ) ;
#2468=ORIENTED_EDGE ( 'NONE', *, *, #8263, .T. ) ;
#2470=EDGE_CURVE ( 'NONE', #6969, #19088, #21305, .T. ) ;
#2473=AXIS2_PLACEMENT_3D ( 'NONE', #17316, #14461, #30817 ) ;
#2475=CARTESIAN_POINT ( 'NONE',  ( -20.00000000000007461, 108.9999999999999858, 162.9999999999999716 ) ) ;
#2477=ORIENTED_EDGE ( 'NONE', *, *, #27413, .F. ) ;
#2480=CARTESIAN_POINT ( 'NONE',  ( -430.0000000000000000, -135.0000000000000000, 113.9999999999999858 ) ) ;
#2481=DIRECTION ( 'NONE',  ( 0.000000000000000000, -3.374343856708137958E-53, 1.000000000000000000 ) ) ;
#2482=ORIENTED_EDGE ( 'NONE', *, *, #6366, .T. ) ;
#2489=VERTEX_POINT ( 'NONE', #15447 ) ;
#2491=CARTESIAN_POINT ( 'NONE',  ( -12.00000000000001066, 136.9999999999999716, 155.0000000000000000 ) ) ;
#2495=DIRECTION ( 'NONE',  ( -0.000000000000000000, 1.000000000000000000, -0.000000000000000000 ) ) ;
#2496=VECTOR ( 'NONE', #5781, 1000.000000000000000 ) ;
#2497=ORIENTED_EDGE ( 'NONE', *, *, #17584, .T. ) ;
#2504=EDGE_CURVE ( 'NONE', #19925, #4827, #10920, .T. ) ;
#2506=DIRECTION ( 'NONE',  ( 1.000000000000000000, 0.000000000000000000, 0.000000000000000000 ) ) ;
#2507=EDGE_CURVE ( 'NONE', #4850, #28271, #16924, .T. ) ;
#2509=DIRECTION ( 'NONE',  ( -0.000000000000000000, -1.000000000000000000, -0.000000000000000000 ) ) ;
#2520=EDGE_CURVE ( 'NONE', #31799, #12400, #12928, .T. ) ;
#2528=CARTESIAN_POINT ( 'NONE',  ( -361.0000000000000000, 124.9999999999999432, 166.9999999999999716 ) ) ;
#2533=EDGE_CURVE ( 'NONE', #25357, #28271, #2777, .T. ) ;
#2534=LINE ( 'NONE', #32545, #22690 ) ;
#2535=DIRECTION ( 'NONE',  ( 1.000000000000000000, 0.000000000000000000, 0.000000000000000000 ) ) ;
#2536=CARTESIAN_POINT ( 'NONE',  ( 19.99999999999998224, 112.9999999999999574, 155.0000000000000000 ) ) ;
#2537=CYLINDRICAL_SURFACE ( 'NONE', #12853, 7.999999999999979572 ) ;
#2539=AXIS2_PLACEMENT_3D ( 'NONE', #2112, #20805, #23826 ) ;
#2541=ORIENTED_EDGE ( 'NONE', *, *, #33568, .T. ) ;
#2542=CARTESIAN_POINT ( 'NONE',  ( -12.00000000000001066, 104.9999999999999858, 154.9999999999999432 ) ) ;
#2543=CARTESIAN_POINT ( 'NONE',  ( -12.00000000000001066, -145.0000000000000000, -186.9999999999999716 ) ) ;
#2544=PLANE ( 'NONE',  #14038 ) ;
#2552=ORIENTED_EDGE ( 'NONE', *, *, #3159, .F. ) ;
#2558=VECTOR ( 'NONE', #4203, 1000.000000000000000 ) ;
#2559=DIRECTION ( 'NONE',  ( -3.040835319149746090E-31, -1.000000000000000000, 0.000000000000000000 ) ) ;
#2561=CLOSED_SHELL ( 'NONE', ( #17393, #4919, #18542, #16810, #20931, #33380, #20339, #33676, #17841, #34520, #6844, #30058, #1144, #16743, #14168, #19359, #11021, #4523 ) ) ;
#2565=ORIENTED_EDGE ( 'NONE', *, *, #19560, .F. ) ;
#2566=DIRECTION ( 'NONE',  ( 1.000000000000000000, 3.040835319149746090E-31, 1.232595164407830946E-32 ) ) ;
#2570=EDGE_LOOP ( 'NONE', ( #10804, #5901, #20792, #29362 ) ) ;
#2571=CARTESIAN_POINT ( 'NONE',  ( -499.9999999999999432, 112.9999999999999574, 159.0000000000000000 ) ) ;
#2574=VERTEX_POINT ( 'NONE', #27514 ) ;
#2578=VECTOR ( 'NONE', #26046, 1000.000000000000000 ) ;
#2579=LINE ( 'NONE', #13452, #12724 ) ;
#2581=DIRECTION ( 'NONE',  ( 0.000000000000000000, 2.309213040847544338E-50, 1.000000000000000000 ) ) ;
#2583=AXIS2_PLACEMENT_3D ( 'NONE', #20877, #1827, #13055 ) ;
#2589=CIRCLE ( 'NONE', #322, 3.999999999999982681 ) ;
#2591=ADVANCED_FACE ( 'NONE', ( #29840 ), #3129, .F. ) ;
#2597=LINE ( 'NONE', #35012, #1375 ) ;
#2607=AXIS2_PLACEMENT_3D ( 'NONE', #9022, #27704, #25022 ) ;
#2609=CARTESIAN_POINT ( 'NONE',  ( -349.0000000000000000, -125.0000000000000284, 126.0000000000000000 ) ) ;
#2612=EDGE_CURVE ( 'NONE', #2702, #19872, #5964, .T. ) ;
#2621=DIRECTION ( 'NONE',  ( -0.000000000000000000, -1.000000000000000000, -0.000000000000000000 ) ) ;
#2623=VECTOR ( 'NONE', #28744, 1000.000000000000000 ) ;
#2624=CIRCLE ( 'NONE', #22530, 7.999999999999979572 ) ;
#2627=FACE_OUTER_BOUND ( 'NONE', #6214, .T. ) ;
#2628=DIRECTION ( 'NONE',  ( 0.000000000000000000, 1.000000000000000000, -3.374343856708137958E-53 ) ) ;
#2629=CIRCLE ( 'NONE', #33914, 3.999999999999982681 ) ;
#2630=ORIENTED_EDGE ( 'NONE', *, *, #18757, .T. ) ;
#2633=CARTESIAN_POINT ( 'NONE',  ( -445.9999999999999432, 113.0000000000000000, -155.0000000000000000 ) ) ;
#2638=ORIENTED_EDGE ( 'NONE', *, *, #5711, .T. ) ;
#2641=ORIENTED_EDGE ( 'NONE', *, *, #10650, .T. ) ;
#2644=EDGE_CURVE ( 'NONE', #21537, #19872, #21820, .T. ) ;
#2645=DIRECTION ( 'NONE',  ( -0.000000000000000000, -0.000000000000000000, -1.000000000000000000 ) ) ;
#2646=EDGE_CURVE ( 'NONE', #3173, #10330, #10658, .T. ) ;
#2647=FACE_OUTER_BOUND ( 'NONE', #2650, .T. ) ;
#2650=EDGE_LOOP ( 'NONE', ( #21092, #2897, #17562, #29919 ) ) ;
#2657=ORIENTED_EDGE ( 'NONE', *, *, #5324, .T. ) ;
#2659=DIRECTION ( 'NONE',  ( 0.000000000000000000, -2.309213040847544338E-50, -1.000000000000000000 ) ) ;
#2660=VERTEX_POINT ( 'NONE', #25724 ) ;
#2663=ORIENTED_EDGE ( 'NONE', *, *, #17299, .T. ) ;
#2666=CARTESIAN_POINT ( 'NONE',  ( -499.9999999999999432, -113.0000000000000000, -162.9999999999999716 ) ) ;
#2668=EDGE_CURVE ( 'NONE', #25012, #24957, #28293, .T. ) ;
#2677=EDGE_CURVE ( 'NONE', #10047, #2660, #10588, .T. ) ;
#2678=EDGE_CURVE ( 'NONE', #3718, #31108, #1489, .T. ) ;
#2681=EDGE_CURVE ( 'NONE', #22142, #2574, #16284, .T. ) ;
#2685=ORIENTED_EDGE ( 'NONE', *, *, #7210, .T. ) ;
#2690=VERTEX_POINT ( 'NONE', #20227 ) ;
#2691=CARTESIAN_POINT ( 'NONE',  ( -414.0000000000000568, 113.0000000000000000, 154.9999999999999716 ) ) ;
#2694=AXIS2_PLACEMENT_3D ( 'NONE', #10403, #12739, #13734 ) ;
#2696=ORIENTED_EDGE ( 'NONE', *, *, #29374, .F. ) ;
#2699=PLANE ( 'NONE',  #7928 ) ;
#2702=VERTEX_POINT ( 'NONE', #28577 ) ;
#2703=AXIS2_PLACEMENT_3D ( 'NONE', #21409, #27444, #24239 ) ;
#2705=VECTOR ( 'NONE', #29725, 1000.000000000000000 ) ;
#2707=DIRECTION ( 'NONE',  ( 0.000000000000000000, 1.000000000000000000, 1.224646799147353207E-16 ) ) ;
#2710=( GEOMETRIC_REPRESENTATION_CONTEXT ( 3 ) GLOBAL_UNCERTAINTY_ASSIGNED_CONTEXT ( ( #30659 ) ) GLOBAL_UNIT_ASSIGNED_CONTEXT ( ( #18957, #29975, #29798 ) ) REPRESENTATION_CONTEXT ( 'NONE', 'WORKASPACE' ) );
#2715=DIRECTION ( 'NONE',  ( 1.000000000000000000, 0.000000000000000000, -1.232595164407831220E-32 ) ) ;
#2716=PLANE ( 'NONE',  #25146 ) ;
#2719=EDGE_CURVE ( 'NONE', #18446, #21633, #34462, .T. ) ;
#2720=AXIS2_PLACEMENT_3D ( 'NONE', #22313, #19133, #24610 ) ;
#2723=EDGE_CURVE ( 'NONE', #27344, #10477, #2038, .T. ) ;
#2726=VERTEX_POINT ( 'NONE', #22539 ) ;
#2728=ORIENTED_EDGE ( 'NONE', *, *, #28653, .T. ) ;
#2733=CARTESIAN_POINT ( 'NONE',  ( -349.0000000000000000, 134.9999999999999716, 130.0000000000000000 ) ) ;
#2734=FACE_OUTER_BOUND ( 'NONE', #7990, .T. ) ;
#2736=ORIENTED_EDGE ( 'NONE', *, *, #20942, .T. ) ;
#2740=AXIS2_PLACEMENT_3D ( 'NONE', #847, #5142, #5842 ) ;
#2741=CARTESIAN_POINT ( 'NONE',  ( -19.99999999999998934, -145.0000000000000000, -186.9999999999999716 ) ) ;
#2742=ORIENTED_EDGE ( 'NONE', *, *, #4936, .F. ) ;
#2743=CARTESIAN_POINT ( 'NONE',  ( -20.00000000000001776, -145.0000000000000000, 162.9999999999999716 ) ) ;
#2746=ORIENTED_EDGE ( 'NONE', *, *, #32285, .T. ) ;
#2750=FACE_OUTER_BOUND ( 'NONE', #30146, .T. ) ;
#2752=( GEOMETRIC_REPRESENTATION_CONTEXT ( 3 ) GLOBAL_UNCERTAINTY_ASSIGNED_CONTEXT ( ( #29100 ) ) GLOBAL_UNIT_ASSIGNED_CONTEXT ( ( #16721, #22754, #3692 ) ) REPRESENTATION_CONTEXT ( 'NONE', 'WORKASPACE' ) );
#2756=LINE ( 'NONE', #25481, #6290 ) ;
#2758=CIRCLE ( 'NONE', #22674, 7.999999999999979572 ) ;
#2762=EDGE_CURVE ( 'NONE', #28976, #3173, #19877, .T. ) ;
#2763=EDGE_CURVE ( 'NONE', #7154, #25708, #9449, .T. ) ;
#2765=CIRCLE ( 'NONE', #27773, 7.999999999999979572 ) ;
#2767=EDGE_CURVE ( 'NONE', #4014, #24757, #22889, .T. ) ;
#2771=ORIENTED_EDGE ( 'NONE', *, *, #440, .F. ) ;
#2773=CARTESIAN_POINT ( 'NONE',  ( 19.99999999999990763, -134.9999999999999716, -186.9999999999999716 ) ) ;
#2776=VECTOR ( 'NONE', #27329, 1000.000000000000000 ) ;
#2777=LINE ( 'NONE', #30015, #7204 ) ;
#2778=DIRECTION ( 'NONE',  ( -1.000000000000000000, 0.000000000000000000, 0.000000000000000000 ) ) ;
#2780=VERTEX_POINT ( 'NONE', #6313 ) ;
#2781=CARTESIAN_POINT ( 'NONE',  ( 15.99999999999998579, 124.9999999999999716, 162.9999999999999716 ) ) ;
#2782=PLANE ( 'NONE',  #18115 ) ;
#2787=CARTESIAN_POINT ( 'NONE',  ( -12.00000000000001066, -24.99999999999999289, -154.9999999999999716 ) ) ;
#2788=DIRECTION ( 'NONE',  ( 0.000000000000000000, 0.000000000000000000, -1.000000000000000000 ) ) ;
#2790=DIRECTION ( 'NONE',  ( 0.000000000000000000, 0.000000000000000000, 1.000000000000000000 ) ) ;
#2793=ORIENTED_EDGE ( 'NONE', *, *, #23749, .T. ) ;
#2795=CARTESIAN_POINT ( 'NONE',  ( 12.00000000000001066, -24.99999999999999289, -175.0000000000000000 ) ) ;
#2798=DIRECTION ( 'NONE',  ( 0.000000000000000000, 0.000000000000000000, 1.000000000000000000 ) ) ;
#2799=( GEOMETRIC_REPRESENTATION_CONTEXT ( 3 ) GLOBAL_UNCERTAINTY_ASSIGNED_CONTEXT ( ( #4875 ) ) GLOBAL_UNIT_ASSIGNED_CONTEXT ( ( #13910, #16067, #30272 ) ) REPRESENTATION_CONTEXT ( 'NONE', 'WORKASPACE' ) );
#2802=LINE ( 'NONE', #19204, #25278 ) ;
#2806=ORIENTED_EDGE ( 'NONE', *, *, #27808, .T. ) ;
#2808=ADVANCED_FACE ( 'NONE', ( #2040 ), #26416, .T. ) ;
#2810=LINE ( 'NONE', #32193, #22381 ) ;
#2813=DIRECTION ( 'NONE',  ( -0.000000000000000000, -0.000000000000000000, 1.000000000000000000 ) ) ;
#2822=DIRECTION ( 'NONE',  ( 1.000000000000000000, 3.469446951953834515E-18, 0.000000000000000000 ) ) ;
#2828=DIRECTION ( 'NONE',  ( 0.000000000000000000, 0.000000000000000000, -1.000000000000000000 ) ) ;
#2831=LINE ( 'NONE', #22065, #29483 ) ;
#2832=CARTESIAN_POINT ( 'NONE',  ( -19.99999999999998934, 4.559999999999908127, 172.9900000000000091 ) ) ;
#2833=ORIENTED_EDGE ( 'NONE', *, *, #18375, .F. ) ;
#2834=EDGE_CURVE ( 'NONE', #1944, #995, #15679, .T. ) ;
#2836=EDGE_CURVE ( 'NONE', #23824, #10179, #4314, .T. ) ;
#2840=DIRECTION ( 'NONE',  ( 0.000000000000000000, 0.000000000000000000, 1.000000000000000000 ) ) ;
#2842=EDGE_CURVE ( 'NONE', #7715, #26754, #12556, .T. ) ;
#2845=CARTESIAN_POINT ( 'NONE',  ( -70.00000000000000000, 4.559999999999909015, -168.2400000000000091 ) ) ;
#2847=LINE ( 'NONE', #25263, #23474 ) ;
#2852=VERTEX_POINT ( 'NONE', #23399 ) ;
#2853=ORIENTED_EDGE ( 'NONE', *, *, #687, .T. ) ;
#2859=CARTESIAN_POINT ( 'NONE',  ( -499.9999999999999432, 136.9999999999999432, 190.9999999999999716 ) ) ;
#2865=CARTESIAN_POINT ( 'NONE',  ( 19.99999999999996092, -145.0000000000000000, 187.0000000000000000 ) ) ;
#2868=DIRECTION ( 'NONE',  ( 0.000000000000000000, -1.131431318426415506E-52, -1.000000000000000000 ) ) ;
#2869=EDGE_LOOP ( 'NONE', ( #2685, #2630, #33156, #15051 ) ) ;
#2870=EDGE_CURVE ( 'NONE', #32496, #17537, #2624, .T. ) ;
#2871=CYLINDRICAL_SURFACE ( 'NONE', #14673, 7.999999999999979572 ) ;
#2876=CARTESIAN_POINT ( 'NONE',  ( -365.0000000000000000, 118.9999999999999716, 126.0000000000000000 ) ) ;
#2877=CARTESIAN_POINT ( 'NONE',  ( -418.0000000000000000, 104.9999999999999858, -190.9999999999999716 ) ) ;
#2878=AXIS2_PLACEMENT_3D ( 'NONE', #7905, #11115, #27288 ) ;
#2882=CARTESIAN_POINT ( 'NONE',  ( 12.00000000000001066, -60.99999999999997158, -175.0000000000000000 ) ) ;
#2883=ORIENTED_EDGE ( 'NONE', *, *, #11401, .T. ) ;
#2884=CYLINDRICAL_SURFACE ( 'NONE', #9910, 2.000000000000001776 ) ;
#2887=ORIENTED_EDGE ( 'NONE', *, *, #4477, .T. ) ;
#2889=DIRECTION ( 'NONE',  ( 0.000000000000000000, -0.000000000000000000, 1.000000000000000000 ) ) ;
#2894=CARTESIAN_POINT ( 'NONE',  ( -15.99999999999998579, -112.9999999999999858, 155.0000000000000000 ) ) ;
#2897=ORIENTED_EDGE ( 'NONE', *, *, #29209, .F. ) ;
#2902=DIRECTION ( 'NONE',  ( 0.000000000000000000, 1.000000000000000000, -6.123233995736766036E-17 ) ) ;
#2903=ORIENTED_EDGE ( 'NONE', *, *, #5568, .T. ) ;
#2904=EDGE_LOOP ( 'NONE', ( #15588, #30122, #18559, #17838, #24354, #19701, #13019, #12225 ) ) ;
#2911=EDGE_CURVE ( 'NONE', #1214, #23491, #10589, .T. ) ;
#2916=ORIENTED_EDGE ( 'NONE', *, *, #2762, .T. ) ;
#2923=CARTESIAN_POINT ( 'NONE',  ( -12.00000000000001066, 108.9999999999999858, -155.0000000000000000 ) ) ;
#2925=CYLINDRICAL_SURFACE ( 'NONE', #29753, 4.750000000000004441 ) ;
#2931=ORIENTED_EDGE ( 'NONE', *, *, #19549, .F. ) ;
#2932=DIRECTION ( 'NONE',  ( 0.000000000000000000, 6.123233995736766036E-17, 1.000000000000000000 ) ) ;
#2935=ORIENTED_EDGE ( 'NONE', *, *, #22794, .F. ) ;
#2937=CIRCLE ( 'NONE', #18870, 4.750000000000004441 ) ;
#2939=AXIS2_PLACEMENT_3D ( 'NONE', #15458, #15637, #17973 ) ;
#2940=ORIENTED_EDGE ( 'NONE', *, *, #28958, .T. ) ;
#2941=LINE ( 'NONE', #33197, #22039 ) ;
#2944=ORIENTED_EDGE ( 'NONE', *, *, #3910, .F. ) ;
#2945=DIRECTION ( 'NONE',  ( 0.000000000000000000, 1.000000000000000000, 1.224646799147353207E-16 ) ) ;
#2952=CARTESIAN_POINT ( 'NONE',  ( -12.00000000000001066, 134.9999999999999432, -194.9999999999999432 ) ) ;
#2955=EDGE_CURVE ( 'NONE', #1469, #26315, #11742, .T. ) ;
#2956=LINE ( 'NONE', #13830, #688 ) ;
#2957=CARTESIAN_POINT ( 'NONE',  ( -499.9999999999999432, -145.0000000000000000, -162.9999999999999716 ) ) ;
#2964=VECTOR ( 'NONE', #7710, 1000.000000000000000 ) ;
#2965=CARTESIAN_POINT ( 'NONE',  ( -418.0000000000000000, 105.0000000000000142, 190.9999999999999716 ) ) ;
#2970=LINE ( 'NONE', #22737, #10981 ) ;
#2974=ADVANCED_FACE ( 'NONE', ( #21610 ), #5736, .T. ) ;
#2975=ADVANCED_FACE ( 'NONE', ( #8776 ), #30138, .F. ) ;
#2977=FACE_OUTER_BOUND ( 'NONE', #33721, .T. ) ;
#2979=DIRECTION ( 'NONE',  ( 0.000000000000000000, 1.000000000000000000, 1.224646799147353207E-16 ) ) ;
#2980=ORIENTED_EDGE ( 'NONE', *, *, #16202, .F. ) ;
#2981=ORIENTED_EDGE ( 'NONE', *, *, #26787, .T. ) ;
#2983=DIRECTION ( 'NONE',  ( 0.000000000000000000, 1.000000000000000000, -3.374343856708137958E-53 ) ) ;
#2984=ORIENTED_EDGE ( 'NONE', *, *, #6255, .F. ) ;
#2987=DIRECTION ( 'NONE',  ( 1.000000000000000000, 0.000000000000000000, 0.000000000000000000 ) ) ;
#2988=AXIS2_PLACEMENT_3D ( 'NONE', #20111, #28631, #4236 ) ;
#2989=DIRECTION ( 'NONE',  ( 0.000000000000000000, -5.145227585319922065E-49, -1.000000000000000000 ) ) ;
#2990=FACE_OUTER_BOUND ( 'NONE', #284, .T. ) ;
#2993=ORIENTED_EDGE ( 'NONE', *, *, #30891, .F. ) ;
#3003=ADVANCED_FACE ( 'NONE', ( #8599 ), #16463, .F. ) ;
#3004=DIRECTION ( 'NONE',  ( 0.000000000000000000, 1.000000000000000000, 5.145227585319922065E-49 ) ) ;
#3007=FACE_OUTER_BOUND ( 'NONE', #7328, .T. ) ;
#3008=VECTOR ( 'NONE', #8091, 1000.000000000000000 ) ;
#3009=EDGE_CURVE ( 'NONE', #27667, #1340, #19302, .T. ) ;
#3013=DIRECTION ( 'NONE',  ( 0.000000000000000000, 0.000000000000000000, -1.000000000000000000 ) ) ;
#3014=LINE ( 'NONE', #5151, #27952 ) ;
#3018=AXIS2_PLACEMENT_3D ( 'NONE', #5628, #8319, #9907 ) ;
#3019=CIRCLE ( 'NONE', #26322, 3.999999999999976019 ) ;
#3021=DIRECTION ( 'NONE',  ( 1.000000000000000000, -0.000000000000000000, -0.000000000000000000 ) ) ;
#3022=DIRECTION ( 'NONE',  ( 0.000000000000000000, 0.000000000000000000, -1.000000000000000000 ) ) ;
#3023=EDGE_CURVE ( 'NONE', #1296, #15995, #27724, .T. ) ;
#3024=EDGE_LOOP ( 'NONE', ( #7604, #23300, #11770, #18423 ) ) ;
#3028=EDGE_CURVE ( 'NONE', #24189, #20636, #1586, .T. ) ;
#3032=EDGE_CURVE ( 'NONE', #11066, #32798, #27159, .T. ) ;
#3035=VERTEX_POINT ( 'NONE', #30315 ) ;
#3037=FACE_OUTER_BOUND ( 'NONE', #19799, .T. ) ;
#3042=VECTOR ( 'NONE', #25346, 1000.000000000000000 ) ;
#3043=ORIENTED_EDGE ( 'NONE', *, *, #1161, .T. ) ;
#3044=ORIENTED_EDGE ( 'NONE', *, *, #16790, .F. ) ;
#3045=CIRCLE ( 'NONE', #4736, 2.000000000000001776 ) ;
#3049=PLANE ( 'NONE',  #34766 ) ;
#3054=PLANE ( 'NONE',  #7835 ) ;
#3056=EDGE_CURVE ( 'NONE', #15311, #11473, #13431, .T. ) ;
#3059=LINE ( 'NONE', #2354, #15537 ) ;
#3060=CARTESIAN_POINT ( 'NONE',  ( -365.0000000000000000, -125.0000000000000284, 113.9999999999999858 ) ) ;
#3063=DIRECTION ( 'NONE',  ( 0.000000000000000000, -3.374343856708137958E-53, 1.000000000000000000 ) ) ;
#3064=ORIENTED_EDGE ( 'NONE', *, *, #17544, .T. ) ;
#3065=LINE ( 'NONE', #29956, #7640 ) ;
#3068=CIRCLE ( 'NONE', #18995, 7.999999999999979572 ) ;
#3069=ORIENTED_EDGE ( 'NONE', *, *, #16942, .T. ) ;
#3072=ORIENTED_EDGE ( 'NONE', *, *, #9962, .F. ) ;
#3076=ORIENTED_EDGE ( 'NONE', *, *, #5235, .F. ) ;
#3077=DIRECTION ( 'NONE',  ( 0.000000000000000000, 0.000000000000000000, 1.000000000000000000 ) ) ;
#3084=DIRECTION ( 'NONE',  ( 1.000000000000000000, 0.000000000000000000, 0.000000000000000000 ) ) ;
#3086=EDGE_LOOP ( 'NONE', ( #32462, #24424, #33087, #4205 ) ) ;
#3093=VERTEX_POINT ( 'NONE', #6448 ) ;
#3095=CARTESIAN_POINT ( 'NONE',  ( -499.9999999999999432, 140.9999999999999716, -187.0000000000000000 ) ) ;
#3097=VECTOR ( 'NONE', #30299, 1000.000000000000000 ) ;
#3098=DIRECTION ( 'NONE',  ( 1.000000000000000000, 0.000000000000000000, 0.000000000000000000 ) ) ;
#3104=VERTEX_POINT ( 'NONE', #25675 ) ;
#3105=CYLINDRICAL_SURFACE ( 'NONE', #30906, 8.000000000000007105 ) ;
#3107=EDGE_CURVE ( 'NONE', #22599, #24075, #33688, .T. ) ;
#3108=DIRECTION ( 'NONE',  ( 1.000000000000000000, 3.469446951953834515E-18, 0.000000000000000000 ) ) ;
#3112=DIRECTION ( 'NONE',  ( 0.000000000000000000, 0.000000000000000000, 1.000000000000000000 ) ) ;
#3115=ADVANCED_FACE ( 'NONE', ( #1131 ), #31031, .T. ) ;
#3117=ORIENTED_EDGE ( 'NONE', *, *, #20580, .T. ) ;
#3118=ADVANCED_FACE ( 'NONE', ( #22678 ), #28181, .T. ) ;
#3119=EDGE_CURVE ( 'NONE', #890, #14045, #22494, .T. ) ;
#3120=AXIS2_PLACEMENT_3D ( 'NONE', #7840, #2495, #18722 ) ;
#3123=DIRECTION ( 'NONE',  ( 0.000000000000000000, -0.000000000000000000, -1.000000000000000000 ) ) ;
#3125=EDGE_LOOP ( 'NONE', ( #3616, #32924, #1986, #12687 ) ) ;
#3127=AXIS2_PLACEMENT_3D ( 'NONE', #25343, #17192, #28023 ) ;
#3128=CARTESIAN_POINT ( 'NONE',  ( -442.0000000000000000, 105.0000000000000142, -109.9999999999999574 ) ) ;
#3129=PLANE ( 'NONE',  #15213 ) ;
#3132=ORIENTED_EDGE ( 'NONE', *, *, #16191, .F. ) ;
#3135=CARTESIAN_POINT ( 'NONE',  ( -410.0000000000000568, -125.0000000000000000, -101.9999999999999858 ) ) ;
#3137=AXIS2_PLACEMENT_3D ( 'NONE', #9823, #34037, #11824 ) ;
#3140=FACE_OUTER_BOUND ( 'NONE', #12161, .T. ) ;
#3147=ORIENTED_EDGE ( 'NONE', *, *, #25539, .T. ) ;
#3149=CYLINDRICAL_SURFACE ( 'NONE', #3018, 4.750000000000004441 ) ;
#3152=DIRECTION ( 'NONE',  ( 0.000000000000000000, -1.000000000000000000, 0.000000000000000000 ) ) ;
#3153=CIRCLE ( 'NONE', #15676, 4.000000000000003553 ) ;
#3155=EDGE_CURVE ( 'NONE', #29056, #20661, #14844, .T. ) ;
#3159=EDGE_CURVE ( 'NONE', #16454, #2208, #775, .T. ) ;
#3164=DIRECTION ( 'NONE',  ( 0.000000000000000000, 6.123233995736766036E-17, 1.000000000000000000 ) ) ;
#3165=EDGE_CURVE ( 'NONE', #24095, #11612, #9550, .T. ) ;
#3173=VERTEX_POINT ( 'NONE', #3606 ) ;
#3174=ORIENTED_EDGE ( 'NONE', *, *, #4000, .T. ) ;
#3177=VECTOR ( 'NONE', #23782, 1000.000000000000000 ) ;
#3180=CARTESIAN_POINT ( 'NONE',  ( -19.99999999999998934, 134.9999999999999432, -186.9999999999999716 ) ) ;
#3186=DIRECTION ( 'NONE',  ( 0.000000000000000000, 1.000000000000000000, 5.053935297177146739E-49 ) ) ;
#3187=FACE_OUTER_BOUND ( 'NONE', #22845, .T. ) ;
#3188=ORIENTED_EDGE ( 'NONE', *, *, #16496, .F. ) ;
#3195=CARTESIAN_POINT ( 'NONE',  ( -12.00000000000001066, -24.99999999999999289, -154.9999999999999716 ) ) ;
#3198=CARTESIAN_POINT ( 'NONE',  ( 19.99999999999996092, -134.9999999999999716, 187.0000000000000000 ) ) ;
#3200=DIRECTION ( 'NONE',  ( -0.000000000000000000, 1.000000000000000000, -0.000000000000000000 ) ) ;
#3201=VECTOR ( 'NONE', #14521, 1000.000000000000000 ) ;
#3207=VERTEX_POINT ( 'NONE', #8962 ) ;
#3208=EDGE_CURVE ( 'NONE', #13474, #14034, #10695, .T. ) ;
#3211=EDGE_CURVE ( 'NONE', #27122, #27900, #17528, .T. ) ;
#3212=CARTESIAN_POINT ( 'NONE',  ( -410.0000000000000568, 104.9999999999999858, -162.9999999999999716 ) ) ;
#3216=DIRECTION ( 'NONE',  ( 0.000000000000000000, 0.000000000000000000, 1.000000000000000000 ) ) ;
#3219=DIRECTION ( 'NONE',  ( -1.000000000000000000, -3.040835319149746090E-31, -1.232595164407830946E-32 ) ) ;
#3221=ORIENTED_EDGE ( 'NONE', *, *, #29312, .F. ) ;
#3226=CARTESIAN_POINT ( 'NONE',  ( 11.99999999999999645, -145.0000000000000000, 162.9999999999999716 ) ) ;
#3233=ORIENTED_EDGE ( 'NONE', *, *, #10411, .F. ) ;
#3234=CARTESIAN_POINT ( 'NONE',  ( -449.9999999999999432, -124.9999999999999858, -77.99999999999997158 ) ) ;
#3236=FACE_OUTER_BOUND ( 'NONE', #2160, .T. ) ;
#3238=CARTESIAN_POINT ( 'NONE',  ( 12.00000000000001066, -32.99999999999997158, -154.9999999999999716 ) ) ;
#3240=EDGE_CURVE ( 'NONE', #8469, #14037, #25142, .T. ) ;
#3244=CARTESIAN_POINT ( 'NONE',  ( -418.0000000000000568, -109.0000000000000142, 155.0000000000000000 ) ) ;
#3246=CARTESIAN_POINT ( 'NONE',  ( -355.0000000000000000, -131.0000000000000000, 113.9999999999999858 ) ) ;
#3248=ORIENTED_EDGE ( 'NONE', *, *, #16108, .F. ) ;
#3249=VECTOR ( 'NONE', #31970, 1000.000000000000000 ) ;
#3252=EDGE_CURVE ( 'NONE', #20130, #8592, #31876, .T. ) ;
#3255=FACE_OUTER_BOUND ( 'NONE', #18591, .T. ) ;
#3256=ORIENTED_EDGE ( 'NONE', *, *, #24538, .F. ) ;
#3257=ORIENTED_EDGE ( 'NONE', *, *, #5123, .T. ) ;
#3258=DIRECTION ( 'NONE',  ( 1.000000000000000000, 0.000000000000000000, 0.000000000000000000 ) ) ;
#3259=CIRCLE ( 'NONE', #16353, 7.999999999999979572 ) ;
#3266=CARTESIAN_POINT ( 'NONE',  ( -499.9999999999999432, 136.9999999999999432, -162.9999999999999716 ) ) ;
#3270=DIRECTION ( 'NONE',  ( 1.000000000000000000, 0.000000000000000000, 0.000000000000000000 ) ) ;
#3271=ORIENTED_EDGE ( 'NONE', *, *, #18711, .F. ) ;
#3279=CARTESIAN_POINT ( 'NONE',  ( -445.9999999999999432, 124.9999999999999432, -162.9999999999999716 ) ) ;
#3284=AXIS2_PLACEMENT_3D ( 'NONE', #11994, #17350, #6801 ) ;
#3285=DIRECTION ( 'NONE',  ( 1.000000000000000000, 0.000000000000000000, -1.848892746611746966E-32 ) ) ;
#3287=DIRECTION ( 'NONE',  ( 0.000000000000000000, 1.000000000000000000, 5.145227585319922065E-49 ) ) ;
#3288=CARTESIAN_POINT ( 'NONE',  ( -449.9999999999999432, 113.0000000000000000, -155.0000000000000000 ) ) ;
#3289=EDGE_CURVE ( 'NONE', #14902, #13276, #32848, .T. ) ;
#3290=VECTOR ( 'NONE', #2707, 1000.000000000000000 ) ;
#3291=VECTOR ( 'NONE', #25073, 1000.000000000000000 ) ;
#3292=ORIENTED_EDGE ( 'NONE', *, *, #10438, .T. ) ;
#3295=ORIENTED_EDGE ( 'NONE', *, *, #23823, .F. ) ;
#3303=DIRECTION ( 'NONE',  ( -5.546364386991661285E-52, 0.000000000000000000, -1.000000000000000000 ) ) ;
#3304=DIRECTION ( 'NONE',  ( 0.000000000000000000, 1.000000000000000000, 1.310824597558155437E-49 ) ) ;
#3310=PLANE ( 'NONE',  #31019 ) ;
#3311=CARTESIAN_POINT ( 'NONE',  ( -500.0000000000000000, -145.0000000000000000, 155.0000000000000000 ) ) ;
#3315=VECTOR ( 'NONE', #11339, 1000.000000000000000 ) ;
#3316=CARTESIAN_POINT ( 'NONE',  ( -442.0000000000000000, 104.9999999999999858, -155.0000000000000000 ) ) ;
#3317=PLANE ( 'NONE',  #28821 ) ;
#3319=VECTOR ( 'NONE', #11736, 1000.000000000000000 ) ;
#3327=EDGE_CURVE ( 'NONE', #3779, #6940, #4412, .T. ) ;
#3332=VECTOR ( 'NONE', #25017, 1000.000000000000000 ) ;
#3338=AXIS2_PLACEMENT_3D ( 'NONE', #17255, #14580, #5824 ) ;
#3343=AXIS2_PLACEMENT_3D ( 'NONE', #4745, #18314, #26127 ) ;
#3345=LINE ( 'NONE', #11014, #7083 ) ;
#3349=ORIENTED_EDGE ( 'NONE', *, *, #32285, .F. ) ;
#3352=CARTESIAN_POINT ( 'NONE',  ( -499.9999999999999432, 140.9999999999999716, 187.0000000000000000 ) ) ;
#3354=VECTOR ( 'NONE', #21223, 1000.000000000000000 ) ;
#3355=EDGE_LOOP ( 'NONE', ( #19479, #17384, #22883, #25319 ) ) ;
#3356=ORIENTED_EDGE ( 'NONE', *, *, #32473, .F. ) ;
#3358=ORIENTED_EDGE ( 'NONE', *, *, #8908, .T. ) ;
#3360=CARTESIAN_POINT ( 'NONE',  ( -499.9999999999999432, 108.9999999999999858, 187.0000000000000000 ) ) ;
#3361=CARTESIAN_POINT ( 'NONE',  ( 11.99999999999999645, -124.9999999999999432, -154.9999999999999716 ) ) ;
#3363=VECTOR ( 'NONE', #22538, 1000.000000000000000 ) ;
#3364=ORIENTED_EDGE ( 'NONE', *, *, #28648, .F. ) ;
#3368=ORIENTED_EDGE ( 'NONE', *, *, #1367, .T. ) ;
#3371=( NAMED_UNIT ( * ) SI_UNIT ( $, .STERADIAN. ) SOLID_ANGLE_UNIT ( ) );
#3372=CARTESIAN_POINT ( 'NONE',  ( -20.00000000000007461, 108.9999999999999858, -187.0000000000000000 ) ) ;
#3374=LINE ( 'NONE', #714, #27619 ) ;
#3376=CARTESIAN_POINT ( 'NONE',  ( -499.9999999999999432, -137.0000000000000000, -194.9999999999999716 ) ) ;
#3377=CARTESIAN_POINT ( 'NONE',  ( -361.0000000000000000, -125.0000000000000284, 164.9999999999999716 ) ) ;
#3378=EDGE_LOOP ( 'NONE', ( #14733, #5601, #22053, #17205 ) ) ;
#3379=VECTOR ( 'NONE', #4134, 1000.000000000000000 ) ;
#3382=ORIENTED_EDGE ( 'NONE', *, *, #12489, .F. ) ;
#3387=ORIENTED_EDGE ( 'NONE', *, *, #10175, .T. ) ;
#3388=DIRECTION ( 'NONE',  ( -0.000000000000000000, 1.000000000000000000, -0.000000000000000000 ) ) ;
#3390=VECTOR ( 'NONE', #6877, 1000.000000000000000 ) ;
#3394=ORIENTED_EDGE ( 'NONE', *, *, #20566, .T. ) ;
#3395=ORIENTED_EDGE ( 'NONE', *, *, #7047, .F. ) ;
#3403=DIRECTION ( 'NONE',  ( 0.000000000000000000, 0.000000000000000000, -1.000000000000000000 ) ) ;
#3405=EDGE_CURVE ( 'NONE', #5775, #19234, #13557, .T. ) ;
#3407=FACE_OUTER_BOUND ( 'NONE', #30676, .T. ) ;
#3414=ORIENTED_EDGE ( 'NONE', *, *, #34154, .F. ) ;
#3415=DIRECTION ( 'NONE',  ( 1.000000000000000000, 0.000000000000000000, -1.848892746611746966E-32 ) ) ;
#3418=AXIS2_PLACEMENT_3D ( 'NONE', #16063, #32404, #23869 ) ;
#3419=EDGE_LOOP ( 'NONE', ( #34031, #18703, #22977, #1042 ) ) ;
#3423=ORIENTED_EDGE ( 'NONE', *, *, #24255, .T. ) ;
#3424=ORIENTED_EDGE ( 'NONE', *, *, #34181, .T. ) ;
#3425=DIRECTION ( 'NONE',  ( 1.000000000000000000, 0.000000000000000000, -1.232595164407831220E-32 ) ) ;
#3433=VECTOR ( 'NONE', #34847, 1000.000000000000000 ) ;
#3434=CYLINDRICAL_SURFACE ( 'NONE', #15232, 7.999999999999979572 ) ;
#3439=VECTOR ( 'NONE', #34121, 1000.000000000000000 ) ;
#3440=CARTESIAN_POINT ( 'NONE',  ( -361.0000000000000000, 134.9999999999999716, 113.9999999999999858 ) ) ;
#3442=ORIENTED_EDGE ( 'NONE', *, *, #32221, .T. ) ;
#3444=CARTESIAN_POINT ( 'NONE',  ( 0.000000000000000000, -55.00000000000000711, -154.9999999999999716 ) ) ;
#3448=( LENGTH_UNIT ( ) NAMED_UNIT ( * ) SI_UNIT ( .MILLI., .METRE. ) );
#3449=VECTOR ( 'NONE', #34223, 1000.000000000000000 ) ;
#3452=DIRECTION ( 'NONE',  ( 0.000000000000000000, -1.000000000000000000, 3.421138828918010427E-49 ) ) ;
#3453=AXIS2_PLACEMENT_3D ( 'NONE', #18456, #10784, #24285 ) ;
#3457=CARTESIAN_POINT ( 'NONE',  ( 12.00000000000001066, 144.9999999999999716, -155.0000000000000000 ) ) ;
#3461=AXIS2_PLACEMENT_3D ( 'NONE', #12744, #34444, #26425 ) ;
#3462=ORIENTED_EDGE ( 'NONE', *, *, #32045, .T. ) ;
#3463=EDGE_CURVE ( 'NONE', #9737, #34245, #25, .T. ) ;
#3473=ADVANCED_FACE ( 'NONE', ( #204 ), #21735, .T. ) ;
#3477=VERTEX_POINT ( 'NONE', #16068 ) ;
#3480=CARTESIAN_POINT ( 'NONE',  ( -349.0000000000000000, -125.0000000000000284, 185.0000000000000000 ) ) ;
#3481=CARTESIAN_POINT ( 'NONE',  ( 11.99999999999999645, 112.9999999999999574, 155.0000000000000000 ) ) ;
#3487=DIRECTION ( 'NONE',  ( 0.000000000000000000, 0.000000000000000000, -1.000000000000000000 ) ) ;
#3488=DIRECTION ( 'NONE',  ( -0.000000000000000000, -0.000000000000000000, 1.000000000000000000 ) ) ;
#3489=LINE ( 'NONE', #33031, #24934 ) ;
#3492=CARTESIAN_POINT ( 'NONE',  ( -20.00000000000007461, 108.9999999999999858, -162.9999999999999716 ) ) ;
#3494=DIRECTION ( 'NONE',  ( 1.000000000000000000, -0.000000000000000000, -0.000000000000000000 ) ) ;
#3500=LINE ( 'NONE', #6697, #30980 ) ;
#3504=CIRCLE ( 'NONE', #103, 3.999999999999976019 ) ;
#3507=CARTESIAN_POINT ( 'NONE',  ( -19.99999999999998934, -137.0000000000000000, 174.9999999999999432 ) ) ;
#3508=CARTESIAN_POINT ( 'NONE',  ( -363.0000000000000000, -125.0000000000000284, 181.0000000000000000 ) ) ;
#3512=ORIENTED_EDGE ( 'NONE', *, *, #30901, .T. ) ;
#3520=ORIENTED_EDGE ( 'NONE', *, *, #1136, .F. ) ;
#3524=LINE ( 'NONE', #15110, #21685 ) ;
#3525=AXIS2_PLACEMENT_3D ( 'NONE', #28640, #17290, #20463 ) ;
#3527=LINE ( 'NONE', #14766, #9119 ) ;
#3528=CIRCLE ( 'NONE', #27979, 4.750000000000004441 ) ;
#3531=DIRECTION ( 'NONE',  ( 0.000000000000000000, -1.000000000000000000, -1.131431318426415506E-52 ) ) ;
#3533=ORIENTED_EDGE ( 'NONE', *, *, #26277, .F. ) ;
#3534=ADVANCED_FACE ( 'NONE', ( #30275 ), #30103, .T. ) ;
#3538=ORIENTED_EDGE ( 'NONE', *, *, #5675, .T. ) ;
#3539=DIRECTION ( 'NONE',  ( 0.000000000000000000, 2.465190328815661892E-32, 1.000000000000000000 ) ) ;
#3545=DIRECTION ( 'NONE',  ( 1.000000000000000000, 0.000000000000000000, 0.000000000000000000 ) ) ;
#3546=CYLINDRICAL_SURFACE ( 'NONE', #27335, 3.999999999999976019 ) ;
#3547=CARTESIAN_POINT ( 'NONE',  ( -499.9999999999999432, -137.0000000000000000, -187.0000000000000000 ) ) ;
#3551=ORIENTED_EDGE ( 'NONE', *, *, #14484, .F. ) ;
#3554=ORIENTED_EDGE ( 'NONE', *, *, #25628, .F. ) ;
#3557=EDGE_CURVE ( 'NONE', #19034, #11831, #23790, .T. ) ;
#3558=CARTESIAN_POINT ( 'NONE',  ( -20.00000000000004619, -134.9999999999999716, -162.9999999999999432 ) ) ;
#3560=FACE_OUTER_BOUND ( 'NONE', #4914, .T. ) ;
#3563=DIRECTION ( 'NONE',  ( -1.000000000000000000, 0.000000000000000000, -0.000000000000000000 ) ) ;
#3569=LINE ( 'NONE', #918, #32756 ) ;
#3570=CARTESIAN_POINT ( 'NONE',  ( -449.9999999999999432, -112.9999999999999858, 155.0000000000000000 ) ) ;
#3571=FACE_OUTER_BOUND ( 'NONE', #24598, .T. ) ;
#3573=ORIENTED_EDGE ( 'NONE', *, *, #14589, .F. ) ;
#3577=CIRCLE ( 'NONE', #25767, 3.999999999999976019 ) ;
#3580=DIRECTION ( 'NONE',  ( 0.000000000000000000, 0.000000000000000000, 1.000000000000000000 ) ) ;
#3583=CARTESIAN_POINT ( 'NONE',  ( 11.99999999999999645, -145.0000000000000000, 194.9999999999999716 ) ) ;
#3584=UNCERTAINTY_MEASURE_WITH_UNIT (LENGTH_MEASURE( 1.000000000000000082E-05 ), #34719, 'distance_accuracy_value', 'NONE');
#3588=CARTESIAN_POINT ( 'NONE',  ( -442.0000000000000000, 105.0000000000000142, 104.0000000000000142 ) ) ;
#3590=VERTEX_POINT ( 'NONE', #17656 ) ;
#3592=VERTEX_POINT ( 'NONE', #1264 ) ;
#3598=VECTOR ( 'NONE', #16576, 1000.000000000000000 ) ;
#3599=ORIENTED_EDGE ( 'NONE', *, *, #15508, .F. ) ;
#3603=EDGE_CURVE ( 'NONE', #10950, #22914, #30987, .T. ) ;
#3604=CYLINDRICAL_SURFACE ( 'NONE', #32656, 3.999999999999976019 ) ;
#3606=CARTESIAN_POINT ( 'NONE',  ( 11.99999999999995559, -145.0000000000000000, 155.0000000000000000 ) ) ;
#3607=DIRECTION ( 'NONE',  ( 1.000000000000000000, 0.000000000000000000, 0.000000000000000000 ) ) ;
#3612=ADVANCED_FACE ( 'NONE', ( #14273 ), #6589, .T. ) ;
#3615=FACE_OUTER_BOUND ( 'NONE', #22346, .T. ) ;
#3616=ORIENTED_EDGE ( 'NONE', *, *, #26274, .F. ) ;
#3619=LINE ( 'NONE', #14152, #31231 ) ;
#3621=DIRECTION ( 'NONE',  ( 1.000000000000000000, 0.000000000000000000, -1.232595164407831220E-32 ) ) ;
#3625=FACE_OUTER_BOUND ( 'NONE', #11815, .T. ) ;
#3626=DIRECTION ( 'NONE',  ( 0.000000000000000000, -1.000000000000000000, 6.123233995736766036E-17 ) ) ;
#3627=VECTOR ( 'NONE', #28725, 1000.000000000000000 ) ;
#3628=AXIS2_PLACEMENT_3D ( 'NONE', #4941, #24162, #10654 ) ;
#3631=CARTESIAN_POINT ( 'NONE',  ( 15.99999999999998579, 136.9999999999999716, -175.0000000000000284 ) ) ;
#3636=ORIENTED_EDGE ( 'NONE', *, *, #27071, .F. ) ;
#3639=ORIENTED_EDGE ( 'NONE', *, *, #34607, .T. ) ;
#3644=CARTESIAN_POINT ( 'NONE',  ( -15.99999999999998579, 4.559999999999908127, -172.9900000000000091 ) ) ;
#3646=EDGE_CURVE ( 'NONE', #17680, #27112, #22974, .T. ) ;
#3647=CARTESIAN_POINT ( 'NONE',  ( -442.0000000000000000, -104.9999999999999574, -155.0000000000000000 ) ) ;
#3653=ORIENTED_EDGE ( 'NONE', *, *, #32935, .T. ) ;
#3659=DIRECTION ( 'NONE',  ( 1.000000000000000000, 0.000000000000000000, 5.546364386991661285E-52 ) ) ;
#3661=DIRECTION ( 'NONE',  ( 0.000000000000000000, 0.000000000000000000, -1.000000000000000000 ) ) ;
#3662=CARTESIAN_POINT ( 'NONE',  ( 19.99999999999998934, 136.9999999999999716, -155.0000000000000000 ) ) ;
#3663=DIRECTION ( 'NONE',  ( 1.000000000000000000, 0.000000000000000000, -1.848892746611746966E-32 ) ) ;
#3667=DIRECTION ( 'NONE',  ( 0.000000000000000000, 1.000000000000000000, 5.053935297177146739E-49 ) ) ;
#3671=AXIS2_PLACEMENT_3D ( 'NONE', #4170, #31411, #6491 ) ;
#3672=CARTESIAN_POINT ( 'NONE',  ( 19.99999999999990763, -134.9999999999999716, -186.9999999999999716 ) ) ;
#3675=VECTOR ( 'NONE', #27004, 1000.000000000000000 ) ;
#3681=ORIENTED_EDGE ( 'NONE', *, *, #11147, .F. ) ;
#3684=CARTESIAN_POINT ( 'NONE',  ( -15.99999999999998579, 112.9999999999999574, -175.0000000000000284 ) ) ;
#3687=ORIENTED_EDGE ( 'NONE', *, *, #6923, .T. ) ;
#3690=ORIENTED_EDGE ( 'NONE', *, *, #18711, .T. ) ;
#3692=( NAMED_UNIT ( * ) SI_UNIT ( $, .STERADIAN. ) SOLID_ANGLE_UNIT ( ) );
#3693=AXIS2_PLACEMENT_3D ( 'NONE', #17303, #22449, #25453 ) ;
#3694=CARTESIAN_POINT ( 'NONE',  ( 11.99999999999999645, -137.0000000000000000, -155.0000000000000284 ) ) ;
#3696=EDGE_CURVE ( 'NONE', #33799, #13964, #14978, .T. ) ;
#3699=ORIENTED_EDGE ( 'NONE', *, *, #29984, .T. ) ;
#3700=ORIENTED_EDGE ( 'NONE', *, *, #30328, .F. ) ;
#3701=AXIS2_PLACEMENT_3D ( 'NONE', #6331, #24852, #16879 ) ;
#3703=VECTOR ( 'NONE', #5056, 1000.000000000000000 ) ;
#3706=FACE_OUTER_BOUND ( 'NONE', #29667, .T. ) ;
#3714=CLOSED_SHELL ( 'NONE', ( #22016, #20429, #24539, #11919, #12502, #26875, #2975, #26753, #28834, #30494, #27955, #27899, #23485, #34594, #21993, #30627, #17140, #15035 ) ) ;
#3715=DIRECTION ( 'NONE',  ( 1.232595164407830946E-32, 3.421138828918010427E-49, -1.000000000000000000 ) ) ;
#3716=DIRECTION ( 'NONE',  ( 1.000000000000000000, 0.000000000000000000, 0.000000000000000000 ) ) ;
#3717=ORIENTED_EDGE ( 'NONE', *, *, #34677, .T. ) ;
#3718=VERTEX_POINT ( 'NONE', #25283 ) ;
#3719=DIRECTION ( 'NONE',  ( -1.000000000000000000, 0.000000000000000000, 1.232595164407831220E-32 ) ) ;
#3720=LINE ( 'NONE', #4407, #4675 ) ;
#3721=EDGE_LOOP ( 'NONE', ( #22976, #9582, #32549, #4228, #33066, #13179, #15785, #9486 ) ) ;
#3722=CARTESIAN_POINT ( 'NONE',  ( -365.0000000000000000, 114.9999999999999716, 126.0000000000000000 ) ) ;
#3727=AXIS2_PLACEMENT_3D ( 'NONE', #11338, #12738, #4349 ) ;
#3732=EDGE_CURVE ( 'NONE', #11647, #1683, #27190, .T. ) ;
#3734=ADVANCED_FACE ( 'NONE', ( #18532 ), #18349, .T. ) ;
#3735=ORIENTED_EDGE ( 'NONE', *, *, #7983, .T. ) ;
#3738=ORIENTED_EDGE ( 'NONE', *, *, #12637, .T. ) ;
#3739=VECTOR ( 'NONE', #16799, 1000.000000000000000 ) ;
#3742=CARTESIAN_POINT ( 'NONE',  ( 19.99999999999998934, 4.559999999999908127, 168.2400000000000091 ) ) ;
#3749=ORIENTED_EDGE ( 'NONE', *, *, #34705, .F. ) ;
#3750=ORIENTED_EDGE ( 'NONE', *, *, #16051, .T. ) ;
#3757=DIRECTION ( 'NONE',  ( 0.000000000000000000, 1.000000000000000000, 1.224646799147353207E-16 ) ) ;
#3758=DIRECTION ( 'NONE',  ( 0.000000000000000000, 0.000000000000000000, 1.000000000000000000 ) ) ;
#3760=EDGE_LOOP ( 'NONE', ( #23980, #2746, #26761, #10875 ) ) ;
#3761=VECTOR ( 'NONE', #27406, 1000.000000000000000 ) ;
#3763=CARTESIAN_POINT ( 'NONE',  ( -499.9999999999999432, 136.9999999999999432, 190.9999999999999716 ) ) ;
#3768=ADVANCED_FACE ( 'NONE', ( #9624 ), #4433, .F. ) ;
#3769=CARTESIAN_POINT ( 'NONE',  ( -442.0000000000000000, -124.9999999999999716, 132.0000000000000000 ) ) ;
#3771=ORIENTED_EDGE ( 'NONE', *, *, #209, .T. ) ;
#3772=CARTESIAN_POINT ( 'NONE',  ( -499.9999999999999432, -137.0000000000000000, -187.0000000000000000 ) ) ;
#3775=EDGE_LOOP ( 'NONE', ( #3699, #28391 ) ) ;
#3777=VECTOR ( 'NONE', #3621, 1000.000000000000000 ) ;
#3779=VERTEX_POINT ( 'NONE', #26154 ) ;
#3785=DIRECTION ( 'NONE',  ( -0.000000000000000000, 0.000000000000000000, 1.000000000000000000 ) ) ;
#3788=ORIENTED_EDGE ( 'NONE', *, *, #14682, .F. ) ;
#3792=CARTESIAN_POINT ( 'NONE',  ( -12.00000000000001066, -137.0000000000000000, -155.0000000000000284 ) ) ;
#3797=CARTESIAN_POINT ( 'NONE',  ( -361.0000000000000000, 124.9999999999999432, 168.9999999999999716 ) ) ;
#3798=EDGE_LOOP ( 'NONE', ( #3814, #27015, #28184, #20013 ) ) ;
#3800=CARTESIAN_POINT ( 'NONE',  ( -19.99999999999998934, -134.9999999999999716, 187.0000000000000000 ) ) ;
#3801=ADVANCED_FACE ( 'NONE', ( #25811 ), #12308, .T. ) ;
#3803=CARTESIAN_POINT ( 'NONE',  ( -442.0000000000000000, -105.0000000000000142, -105.9999999999999574 ) ) ;
#3811=DIRECTION ( 'NONE',  ( -1.000000000000000000, 0.000000000000000000, -0.000000000000000000 ) ) ;
#3814=ORIENTED_EDGE ( 'NONE', *, *, #7486, .T. ) ;
#3815=CIRCLE ( 'NONE', #23724, 4.750000000000004441 ) ;
#3816=CIRCLE ( 'NONE', #4954, 3.999999999999976019 ) ;
#3817=ORIENTED_EDGE ( 'NONE', *, *, #31883, .F. ) ;
#3819=ORIENTED_EDGE ( 'NONE', *, *, #15759, .F. ) ;
#3821=CARTESIAN_POINT ( 'NONE',  ( -349.0000000000000000, -125.0000000000000284, 181.0000000000000000 ) ) ;
#3825=FACE_OUTER_BOUND ( 'NONE', #4403, .T. ) ;
#3831=LINE ( 'NONE', #33743, #30069 ) ;
#3832=CARTESIAN_POINT ( 'NONE',  ( -418.0000000000000000, -105.0000000000000142, 162.9999999999999716 ) ) ;
#3835=CARTESIAN_POINT ( 'NONE',  ( -70.00000000000000000, 75.55999999999990280, 168.2400000000000091 ) ) ;
#3837=CARTESIAN_POINT ( 'NONE',  ( 15.99999999999997868, 136.9999999999999716, -155.0000000000000000 ) ) ;
#3842=AXIS2_PLACEMENT_3D ( 'NONE', #32775, #27614, #14104 ) ;
#3858=ORIENTED_EDGE ( 'NONE', *, *, #3032, .F. ) ;
#3864=CARTESIAN_POINT ( 'NONE',  ( -12.00000000000003908, -134.9999999999999716, -186.9999999999999716 ) ) ;
#3866=LINE ( 'NONE', #14758, #22204 ) ;
#3867=ORIENTED_EDGE ( 'NONE', *, *, #34646, .T. ) ;
#3868=ORIENTED_EDGE ( 'NONE', *, *, #28445, .F. ) ;
#3869=CIRCLE ( 'NONE', #9585, 7.999999999999979572 ) ;
#3871=CARTESIAN_POINT ( 'NONE',  ( -349.0000000000000000, -135.0000000000000000, 111.9999999999999858 ) ) ;
#3874=CARTESIAN_POINT ( 'NONE',  ( 11.99999999999999645, 144.9999999999999716, -175.0000000000000284 ) ) ;
#3875=DIRECTION ( 'NONE',  ( 0.000000000000000000, -0.000000000000000000, 1.000000000000000000 ) ) ;
#3878=CARTESIAN_POINT ( 'NONE',  ( -430.0000000000000000, -119.0000000000000000, 113.9999999999999858 ) ) ;
#3879=EDGE_LOOP ( 'NONE', ( #30099, #2641, #11280, #34208 ) ) ;
#3880=DIRECTION ( 'NONE',  ( 0.000000000000000000, 0.000000000000000000, -1.000000000000000000 ) ) ;
#3882=AXIS2_PLACEMENT_3D ( 'NONE', #16215, #174, #11029 ) ;
#3887=ORIENTED_EDGE ( 'NONE', *, *, #3909, .T. ) ;
#3890=DIRECTION ( 'NONE',  ( -8.673617379884057166E-16, 0.000000000000000000, -1.000000000000000000 ) ) ;
#3896=DIRECTION ( 'NONE',  ( -1.000000000000000000, 0.000000000000000000, 0.000000000000000000 ) ) ;
#3903=EDGE_CURVE ( 'NONE', #26143, #25412, #25513, .T. ) ;
#3904=CARTESIAN_POINT ( 'NONE',  ( -365.0000000000000000, 118.9999999999999716, 109.9999999999999858 ) ) ;
#3909=EDGE_CURVE ( 'NONE', #23491, #25411, #18156, .T. ) ;
#3910=EDGE_CURVE ( 'NONE', #26361, #34601, #2534, .T. ) ;
#3913=DIRECTION ( 'NONE',  ( 1.000000000000000000, 0.000000000000000000, 5.546364386991661285E-52 ) ) ;
#3916=ORIENTED_EDGE ( 'NONE', *, *, #7351, .T. ) ;
#3919=CARTESIAN_POINT ( 'NONE',  ( -430.0000000000000000, 118.9999999999999716, 130.0000000000000000 ) ) ;
#3922=VECTOR ( 'NONE', #4359, 1000.000000000000000 ) ;
#3923=CARTESIAN_POINT ( 'NONE',  ( -499.9999999999999432, 136.9999999999999432, -187.0000000000000000 ) ) ;
#3926=DIRECTION ( 'NONE',  ( -2.736911063134582149E-48, 7.888609052210118054E-31, 1.000000000000000000 ) ) ;
#3927=FACE_OUTER_BOUND ( 'NONE', #5183, .T. ) ;
#3929=CARTESIAN_POINT ( 'NONE',  ( -445.9999999999999432, -105.0000000000000142, 162.9999999999999716 ) ) ;
#3930=DIRECTION ( 'NONE',  ( -1.000000000000000000, 0.000000000000000000, 0.000000000000000000 ) ) ;
#3932=EDGE_CURVE ( 'NONE', #23023, #15358, #2765, .T. ) ;
#3933=DIRECTION ( 'NONE',  ( 0.000000000000000000, 1.000000000000000000, 5.053935297177146739E-49 ) ) ;
#3936=CYLINDRICAL_SURFACE ( 'NONE', #13907, 7.999999999999979572 ) ;
#3938=VECTOR ( 'NONE', #10720, 1000.000000000000000 ) ;
#3941=ORIENTED_EDGE ( 'NONE', *, *, #5755, .F. ) ;
#3944=ORIENTED_EDGE ( 'NONE', *, *, #30322, .F. ) ;
#3947=DIRECTION ( 'NONE',  ( 0.000000000000000000, 0.000000000000000000, -1.000000000000000000 ) ) ;
#3948=EDGE_CURVE ( 'NONE', #21689, #3592, #32313, .T. ) ;
#3953=PLANE ( 'NONE',  #26798 ) ;
#3954=ORIENTED_EDGE ( 'NONE', *, *, #6812, .F. ) ;
#3955=ORIENTED_EDGE ( 'NONE', *, *, #12742, .F. ) ;
#3958=FACE_OUTER_BOUND ( 'NONE', #9532, .T. ) ;
#3959=DIRECTION ( 'NONE',  ( 1.000000000000000000, 0.000000000000000000, -1.848892746611746966E-32 ) ) ;
#3963=CARTESIAN_POINT ( 'NONE',  ( -442.0000000000000000, -125.0000000000000000, -109.9999999999999574 ) ) ;
#3965=DIRECTION ( 'NONE',  ( 0.000000000000000000, 0.000000000000000000, -1.000000000000000000 ) ) ;
#3969=LINE ( 'NONE', #14155, #34822 ) ;
#3970=CARTESIAN_POINT ( 'NONE',  ( -500.0000000000000000, -109.0000000000000142, 187.0000000000000000 ) ) ;
#3979=DIRECTION ( 'NONE',  ( 0.000000000000000000, 0.000000000000000000, -1.000000000000000000 ) ) ;
#3980=ORIENTED_EDGE ( 'NONE', *, *, #32786, .F. ) ;
#3984=EDGE_LOOP ( 'NONE', ( #5832, #24451, #13414, #26486 ) ) ;
#3988=LINE ( 'NONE', #23396, #20731 ) ;
#3989=EDGE_CURVE ( 'NONE', #3035, #2043, #33392, .T. ) ;
#3996=EDGE_LOOP ( 'NONE', ( #3117, #19286, #33918, #24462 ) ) ;
#4000=EDGE_CURVE ( 'NONE', #14760, #32651, #14371, .T. ) ;
#4002=CARTESIAN_POINT ( 'NONE',  ( -418.0000000000000000, -105.0000000000000142, -77.99999999999997158 ) ) ;
#4003=DIRECTION ( 'NONE',  ( -1.000000000000000000, 0.000000000000000000, 0.000000000000000000 ) ) ;
#4006=CARTESIAN_POINT ( 'NONE',  ( -442.0000000000000000, 105.0000000000000142, 104.0000000000000142 ) ) ;
#4011=DIRECTION ( 'NONE',  ( 0.000000000000000000, -5.053935297177146739E-49, -1.000000000000000000 ) ) ;
#4013=CARTESIAN_POINT ( 'NONE',  ( -349.0000000000000000, -125.0000000000000284, 168.9999999999999716 ) ) ;
#4014=VERTEX_POINT ( 'NONE', #14549 ) ;
#4018=AXIS2_PLACEMENT_3D ( 'NONE', #34084, #31922, #2213 ) ;
#4020=DIRECTION ( 'NONE',  ( 0.000000000000000000, 0.000000000000000000, 1.000000000000000000 ) ) ;
#4023=AXIS2_PLACEMENT_3D ( 'NONE', #5496, #30242, #24893 ) ;
#4026=ADVANCED_FACE ( 'NONE', ( #12053 ), #25376, .T. ) ;
#4028=ORIENTED_EDGE ( 'NONE', *, *, #22404, .T. ) ;
#4029=CARTESIAN_POINT ( 'NONE',  ( -442.0000000000000000, 105.0000000000000142, -105.9999999999999574 ) ) ;
#4031=LINE ( 'NONE', #24305, #19265 ) ;
#4035=ORIENTED_EDGE ( 'NONE', *, *, #33177, .T. ) ;
#4036=ORIENTED_EDGE ( 'NONE', *, *, #2377, .F. ) ;
#4038=EDGE_CURVE ( 'NONE', #32731, #5950, #1177, .T. ) ;
#4039=LINE ( 'NONE', #21654, #4959 ) ;
#4041=AXIS2_PLACEMENT_3D ( 'NONE', #23533, #1304, #18214 ) ;
#4046=DIRECTION ( 'NONE',  ( 1.000000000000000000, 0.000000000000000000, 5.546364386991661285E-52 ) ) ;
#4049=EDGE_CURVE ( 'NONE', #30605, #28861, #33464, .T. ) ;
#4052=ORIENTED_EDGE ( 'NONE', *, *, #24210, .T. ) ;
#4054=VECTOR ( 'NONE', #1058, 1000.000000000000000 ) ;
#4055=AXIS2_PLACEMENT_3D ( 'NONE', #24335, #10829, #18681 ) ;
#4057=VECTOR ( 'NONE', #1378, 1000.000000000000000 ) ;
#4061=FACE_OUTER_BOUND ( 'NONE', #34468, .T. ) ;
#4062=CARTESIAN_POINT ( 'NONE',  ( -12.00000000000001243, 134.9999999999998863, 194.9999999999999716 ) ) ;
#4065=DIRECTION ( 'NONE',  ( 0.000000000000000000, 1.131431318426415506E-52, 1.000000000000000000 ) ) ;
#4068=ORIENTED_EDGE ( 'NONE', *, *, #2083, .F. ) ;
#4070=ORIENTED_EDGE ( 'NONE', *, *, #16062, .T. ) ;
#4071=STYLED_ITEM('',(#35254),#34697);
#4077=STYLED_ITEM('',(#35254),#22940);
#4078=FACE_OUTER_BOUND ( 'NONE', #8648, .T. ) ;
#4080=EDGE_CURVE ( 'NONE', #4999, #28476, #4180, .T. ) ;
#4086=EDGE_CURVE ( 'NONE', #18640, #26094, #6324, .T. ) ;
#4088=CARTESIAN_POINT ( 'NONE',  ( -15.99999999999998579, 112.9999999999999574, 155.0000000000000000 ) ) ;
#4093=ORIENTED_EDGE ( 'NONE', *, *, #19106, .F. ) ;
#4094=CARTESIAN_POINT ( 'NONE',  ( 11.99999999999999645, -55.00000000000002132, 162.9999999999999716 ) ) ;
#4095=LINE ( 'NONE', #575, #30784 ) ;
#4096=EDGE_CURVE ( 'NONE', #25358, #9066, #28584, .T. ) ;
#4098=( GEOMETRIC_REPRESENTATION_CONTEXT ( 3 ) GLOBAL_UNCERTAINTY_ASSIGNED_CONTEXT ( ( #25613 ) ) GLOBAL_UNIT_ASSIGNED_CONTEXT ( ( #8063, #29960, #10386 ) ) REPRESENTATION_CONTEXT ( 'NONE', 'WORKASPACE' ) );
#4101=AXIS2_PLACEMENT_3D ( 'NONE', #27486, #32467, #87 ) ;
#4104=CYLINDRICAL_SURFACE ( 'NONE', #28079, 7.999999999999979572 ) ;
#4106=EDGE_LOOP ( 'NONE', ( #34387, #8961, #21574, #7753 ) ) ;
#4108=CARTESIAN_POINT ( 'NONE',  ( -414.0000000000000568, -104.9999999999999716, -187.0000000000000000 ) ) ;
#4109=EDGE_CURVE ( 'NONE', #2043, #30447, #5597, .T. ) ;
#4115=EDGE_CURVE ( 'NONE', #12833, #20076, #34266, .T. ) ;
#4118=ORIENTED_EDGE ( 'NONE', *, *, #15716, .F. ) ;
#4119=VERTEX_POINT ( 'NONE', #20234 ) ;
#4125=CIRCLE ( 'NONE', #30289, 7.999999999999979572 ) ;
#4130=EDGE_CURVE ( 'NONE', #5771, #34350, #20406, .T. ) ;
#4131=CIRCLE ( 'NONE', #9283, 3.999999999999976019 ) ;
#4133=PLANE ( 'NONE',  #32867 ) ;
#4134=DIRECTION ( 'NONE',  ( -2.154935995002245207E-17, -0.000000000000000000, -1.000000000000000000 ) ) ;
#4135=EDGE_CURVE ( 'NONE', #26110, #27224, #20058, .T. ) ;
#4137=DIRECTION ( 'NONE',  ( 0.000000000000000000, 1.310824597558155437E-49, 1.000000000000000000 ) ) ;
#4138=ORIENTED_EDGE ( 'NONE', *, *, #18585, .T. ) ;
#4141=LINE ( 'NONE', #1318, #6224 ) ;
#4151=VERTEX_POINT ( 'NONE', #12398 ) ;
#4155=EDGE_CURVE ( 'NONE', #27008, #20630, #525, .T. ) ;
#4157=EDGE_CURVE ( 'NONE', #9482, #31417, #3831, .T. ) ;
#4158=VECTOR ( 'NONE', #14740, 1000.000000000000000 ) ;
#4162=EDGE_CURVE ( 'NONE', #15683, #21641, #4456, .T. ) ;
#4163=ORIENTED_EDGE ( 'NONE', *, *, #1578, .F. ) ;
#4166=ORIENTED_EDGE ( 'NONE', *, *, #30180, .F. ) ;
#4167=LINE ( 'NONE', #33376, #20218 ) ;
#4168=ORIENTED_EDGE ( 'NONE', *, *, #2322, .F. ) ;
#4170=CARTESIAN_POINT ( 'NONE',  ( -355.0000000000000000, -131.0000000000000000, 126.0000000000000000 ) ) ;
#4176=ORIENTED_EDGE ( 'NONE', *, *, #27559, .T. ) ;
#4177=FACE_OUTER_BOUND ( 'NONE', #4106, .T. ) ;
#4180=LINE ( 'NONE', #7024, #24359 ) ;
#4185=CIRCLE ( 'NONE', #13304, 3.999999999999976019 ) ;
#4186=AXIS2_PLACEMENT_3D ( 'NONE', #26311, #31818, #1923 ) ;
#4190=FACE_OUTER_BOUND ( 'NONE', #9934, .T. ) ;
#4191=CARTESIAN_POINT ( 'NONE',  ( -499.9999999999999432, -145.0000000000000000, -187.0000000000000000 ) ) ;
#4192=ORIENTED_EDGE ( 'NONE', *, *, #7606, .F. ) ;
#4195=CARTESIAN_POINT ( 'NONE',  ( -20.00000000000001776, -113.0000000000000000, 162.9999999999999716 ) ) ;
#4196=LINE ( 'NONE', #28599, #17996 ) ;
#4197=CARTESIAN_POINT ( 'NONE',  ( -418.0000000000000000, 105.0000000000000142, 187.0000000000000000 ) ) ;
#4198=EDGE_CURVE ( 'NONE', #3093, #27516, #4691, .T. ) ;
#4201=VERTEX_POINT ( 'NONE', #10061 ) ;
#4203=DIRECTION ( 'NONE',  ( -0.000000000000000000, -1.000000000000000000, -0.000000000000000000 ) ) ;
#4204=EDGE_LOOP ( 'NONE', ( #19728, #10031, #465, #31777, #8470, #32755, #90, #28432 ) ) ;
#4205=ORIENTED_EDGE ( 'NONE', *, *, #27074, .T. ) ;
#4206=AXIS2_PLACEMENT_3D ( 'NONE', #29210, #1456, #4280 ) ;
#4211=CARTESIAN_POINT ( 'NONE',  ( -12.00000000000001066, 144.9999999999999716, -162.9999999999999432 ) ) ;
#4213=DIRECTION ( 'NONE',  ( 0.000000000000000000, 0.000000000000000000, -1.000000000000000000 ) ) ;
#4214=DIRECTION ( 'NONE',  ( 1.000000000000000000, 0.000000000000000000, 0.000000000000000000 ) ) ;
#4215=PLANE ( 'NONE',  #18808 ) ;
#4217=EDGE_LOOP ( 'NONE', ( #20947, #3687, #25310, #12057 ) ) ;
#4219=ORIENTED_EDGE ( 'NONE', *, *, #31323, .T. ) ;
#4222=DIRECTION ( 'NONE',  ( -0.000000000000000000, 1.000000000000000000, -0.000000000000000000 ) ) ;
#4226=CARTESIAN_POINT ( 'NONE',  ( -20.00000000000007461, 136.9999999999999432, -162.9999999999999716 ) ) ;
#4228=ORIENTED_EDGE ( 'NONE', *, *, #15554, .T. ) ;
#4236=DIRECTION ( 'NONE',  ( -1.000000000000000000, 0.000000000000000000, 0.000000000000000000 ) ) ;
#4240=CARTESIAN_POINT ( 'NONE',  ( -430.0000000000000000, 130.9999999999999716, 113.9999999999999858 ) ) ;
#4243=LINE ( 'NONE', #10295, #22447 ) ;
#4245=ADVANCED_FACE ( 'NONE', ( #32286 ), #21267, .T. ) ;
#4246=ORIENTED_EDGE ( 'NONE', *, *, #31612, .F. ) ;
#4254=DIRECTION ( 'NONE',  ( 0.000000000000000000, 0.000000000000000000, -1.000000000000000000 ) ) ;
#4263=LINE ( 'NONE', #4432, #18465 ) ;
#4266=ORIENTED_EDGE ( 'NONE', *, *, #16350, .T. ) ;
#4267=CARTESIAN_POINT ( 'NONE',  ( -12.00000000000001243, 134.9999999999999432, -154.9999999999999716 ) ) ;
#4277=LINE ( 'NONE', #4613, #1905 ) ;
#4280=DIRECTION ( 'NONE',  ( 0.000000000000000000, 0.000000000000000000, -1.000000000000000000 ) ) ;
#4281=CARTESIAN_POINT ( 'NONE',  ( -355.0000000000000000, -135.0000000000000000, 126.0000000000000000 ) ) ;
#4286=EDGE_CURVE ( 'NONE', #33838, #28629, #19301, .T. ) ;
#4287=VERTEX_POINT ( 'NONE', #1864 ) ;
#4290=ORIENTED_EDGE ( 'NONE', *, *, #10214, .F. ) ;
#4295=EDGE_LOOP ( 'NONE', ( #7356, #9666, #24294, #16465 ) ) ;
#4296=ORIENTED_EDGE ( 'NONE', *, *, #4439, .F. ) ;
#4298=CIRCLE ( 'NONE', #28178, 7.999999999999979572 ) ;
#4304=ORIENTED_EDGE ( 'NONE', *, *, #33067, .F. ) ;
#4306=LINE ( 'NONE', #25682, #6157 ) ;
#4307=VECTOR ( 'NONE', #35083, 1000.000000000000000 ) ;
#4308=LINE ( 'NONE', #31207, #18756 ) ;
#4310=DIRECTION ( 'NONE',  ( 0.000000000000000000, 2.309213040847544338E-50, 1.000000000000000000 ) ) ;
#4314=CIRCLE ( 'NONE', #25999, 4.750000000000004441 ) ;
#4315=FACE_OUTER_BOUND ( 'NONE', #14554, .T. ) ;
#4318=DIRECTION ( 'NONE',  ( 1.000000000000000000, 3.469446951953834515E-18, 0.000000000000000000 ) ) ;
#4321=CARTESIAN_POINT ( 'NONE',  ( -347.0000000000000000, -135.0000000000000000, 114.0000000000000000 ) ) ;
#4323=VECTOR ( 'NONE', #6410, 1000.000000000000000 ) ;
#4326=CARTESIAN_POINT ( 'NONE',  ( -441.9999999999999432, 109.0000000000000142, -155.0000000000000000 ) ) ;
#4331=EDGE_CURVE ( 'NONE', #15148, #28176, #22147, .T. ) ;
#4336=EDGE_LOOP ( 'NONE', ( #30738, #3257, #24577, #34392 ) ) ;
#4338=EDGE_LOOP ( 'NONE', ( #32300, #31582, #259, #10240 ) ) ;
#4340=DIRECTION ( 'NONE',  ( 0.000000000000000000, 0.000000000000000000, 1.000000000000000000 ) ) ;
#4346=DIRECTION ( 'NONE',  ( -1.000000000000000000, 0.000000000000000000, 1.848892746611746966E-32 ) ) ;
#4347=ORIENTED_EDGE ( 'NONE', *, *, #32215, .T. ) ;
#4349=DIRECTION ( 'NONE',  ( 0.000000000000000000, 0.000000000000000000, 1.000000000000000000 ) ) ;
#4354=CARTESIAN_POINT ( 'NONE',  ( -363.0000000000000000, -125.0000000000000284, 168.9999999999999716 ) ) ;
#4357=EDGE_CURVE ( 'NONE', #27282, #5434, #22849, .T. ) ;
#4358=CARTESIAN_POINT ( 'NONE',  ( -12.00000000000001066, -141.0000000000000000, 174.9999999999999432 ) ) ;
#4359=DIRECTION ( 'NONE',  ( -1.000000000000000000, -3.469446951953834515E-18, 0.000000000000000000 ) ) ;
#4365=ORIENTED_EDGE ( 'NONE', *, *, #21259, .F. ) ;
#4366=CARTESIAN_POINT ( 'NONE',  ( 11.99999999999999645, -55.00000000000002132, 159.0000000000000000 ) ) ;
#4369=CARTESIAN_POINT ( 'NONE',  ( -430.0000000000000000, 118.9999999999999858, 111.9999999999999858 ) ) ;
#4370=DIRECTION ( 'NONE',  ( -0.000000000000000000, 1.000000000000000000, -0.000000000000000000 ) ) ;
#4375=CARTESIAN_POINT ( 'NONE',  ( -499.9999999999999432, 112.9999999999999574, -190.9999999999999716 ) ) ;
#4378=AXIS2_PLACEMENT_3D ( 'NONE', #17225, #3659, #11878 ) ;
#4380=VERTEX_POINT ( 'NONE', #25507 ) ;
#4382=EDGE_LOOP ( 'NONE', ( #22835, #31284, #25271, #23563, #29961, #31171, #28671, #30939 ) ) ;
#4383=DIRECTION ( 'NONE',  ( 0.000000000000000000, 0.000000000000000000, 1.000000000000000000 ) ) ;
#4385=VECTOR ( 'NONE', #1005, 1000.000000000000000 ) ;
#4386=DIRECTION ( 'NONE',  ( 0.000000000000000000, 1.000000000000000000, 5.145227585319922065E-49 ) ) ;
#4390=ORIENTED_EDGE ( 'NONE', *, *, #28648, .T. ) ;
#4393=CARTESIAN_POINT ( 'NONE',  ( -499.9999999999999432, -137.0000000000000000, -190.9999999999999716 ) ) ;
#4396=AXIS2_PLACEMENT_3D ( 'NONE', #27265, #16080, #26913 ) ;
#4397=VECTOR ( 'NONE', #1414, 1000.000000000000000 ) ;
#4400=CARTESIAN_POINT ( 'NONE',  ( -12.00000000000001066, 124.9999999999999716, 162.9999999999999716 ) ) ;
#4402=CARTESIAN_POINT ( 'NONE',  ( -418.0000000000000000, -124.9999999999999716, 139.9999999999999716 ) ) ;
#4403=EDGE_LOOP ( 'NONE', ( #14298, #34100, #23735, #8109, #27306, #23278, #16549, #34199, #20809, #21026, #31588 ) ) ;
#4406=ORIENTED_EDGE ( 'NONE', *, *, #27074, .F. ) ;
#4407=CARTESIAN_POINT ( 'NONE',  ( -445.9999999999999432, 113.0000000000000000, -175.0000000000000000 ) ) ;
#4410=CARTESIAN_POINT ( 'NONE',  ( -12.00000000000001066, 144.9999999999999147, 155.0000000000000000 ) ) ;
#4412=CIRCLE ( 'NONE', #24306, 7.999999999999979572 ) ;
#4413=CARTESIAN_POINT ( 'NONE',  ( -499.9999999999999432, -137.0000000000000000, -187.0000000000000000 ) ) ;
#4421=VERTEX_POINT ( 'NONE', #15193 ) ;
#4422=CIRCLE ( 'NONE', #34581, 4.000000000000003553 ) ;
#4427=EDGE_LOOP ( 'NONE', ( #1158, #7109, #33611, #4266 ) ) ;
#4431=EDGE_CURVE ( 'NONE', #23023, #10318, #15020, .T. ) ;
#4432=CARTESIAN_POINT ( 'NONE',  ( -15.99999999999998579, 144.9999999999999716, 162.9999999999999716 ) ) ;
#4433=CYLINDRICAL_SURFACE ( 'NONE', #13006, 3.999999999999976019 ) ;
#4436=ORIENTED_EDGE ( 'NONE', *, *, #20528, .F. ) ;
#4438=ORIENTED_EDGE ( 'NONE', *, *, #1518, .F. ) ;
#4439=EDGE_CURVE ( 'NONE', #32813, #26771, #28367, .T. ) ;
#4444=CARTESIAN_POINT ( 'NONE',  ( 19.99999999999996092, -145.0000000000000000, -186.9999999999999716 ) ) ;
#4445=ORIENTED_EDGE ( 'NONE', *, *, #17253, .T. ) ;
#4447=CARTESIAN_POINT ( 'NONE',  ( -12.00000000000001066, 136.9999999999999716, -155.0000000000000000 ) ) ;
#4448=CARTESIAN_POINT ( 'NONE',  ( -500.0000000000000000, -113.0000000000000000, 190.9999999999999716 ) ) ;
#4449=( GEOMETRIC_REPRESENTATION_CONTEXT ( 3 ) GLOBAL_UNCERTAINTY_ASSIGNED_CONTEXT ( ( #33141 ) ) GLOBAL_UNIT_ASSIGNED_CONTEXT ( ( #29332, #1912, #12795 ) ) REPRESENTATION_CONTEXT ( 'NONE', 'WORKASPACE' ) );
#4453=PLANE ( 'NONE',  #83 ) ;
#4455=CARTESIAN_POINT ( 'NONE',  ( 11.99999999999999645, 144.9999999999999716, -194.9999999999999432 ) ) ;
#4456=CIRCLE ( 'NONE', #18701, 7.999999999999979572 ) ;
#4459=ORIENTED_EDGE ( 'NONE', *, *, #29162, .F. ) ;
#4460=ORIENTED_EDGE ( 'NONE', *, *, #34428, .F. ) ;
#4464=ORIENTED_EDGE ( 'NONE', *, *, #16564, .T. ) ;
#4465=VERTEX_POINT ( 'NONE', #1138 ) ;
#4467=EDGE_CURVE ( 'NONE', #31336, #5775, #4308, .T. ) ;
#4470=VERTEX_POINT ( 'NONE', #1483 ) ;
#4471=DIRECTION ( 'NONE',  ( 1.000000000000000000, 0.000000000000000000, -1.232595164407831220E-32 ) ) ;
#4474=ORIENTED_EDGE ( 'NONE', *, *, #4439, .T. ) ;
#4477=EDGE_CURVE ( 'NONE', #20630, #26019, #9318, .T. ) ;
#4478=DIRECTION ( 'NONE',  ( 0.000000000000000000, -1.000000000000000000, 0.000000000000000000 ) ) ;
#4479=CARTESIAN_POINT ( 'NONE',  ( -363.0000000000000000, 134.9999999999999716, 113.9999999999999858 ) ) ;
#4483=LINE ( 'NONE', #10021, #1472 ) ;
#4485=EDGE_CURVE ( 'NONE', #21809, #5416, #7331, .T. ) ;
#4488=PLANE ( 'NONE',  #5978 ) ;
#4489=LINE ( 'NONE', #15204, #28043 ) ;
#4492=DIRECTION ( 'NONE',  ( -1.000000000000000000, 0.000000000000000000, -1.300283923313630633E-47 ) ) ;
#4502=EDGE_LOOP ( 'NONE', ( #15801, #16144, #1860, #32324 ) ) ;
#4505=DIRECTION ( 'NONE',  ( -0.000000000000000000, 1.000000000000000000, -0.000000000000000000 ) ) ;
#4507=VERTEX_POINT ( 'NONE', #33521 ) ;
#4508=LINE ( 'NONE', #15399, #17907 ) ;
#4512=ORIENTED_EDGE ( 'NONE', *, *, #24251, .F. ) ;
#4513=CARTESIAN_POINT ( 'NONE',  ( -430.0000000000000000, 130.9999999999999716, 130.0000000000000000 ) ) ;
#4514=CARTESIAN_POINT ( 'NONE',  ( -418.0000000000000000, -104.9999999999999858, -162.9999999999999716 ) ) ;
#4516=EDGE_CURVE ( 'NONE', #25899, #17680, #25683, .T. ) ;
#4519=ORIENTED_EDGE ( 'NONE', *, *, #16453, .F. ) ;
#4523=ADVANCED_FACE ( 'NONE', ( #25864, #12352 ), #28008, .T. ) ;
#4535=CARTESIAN_POINT ( 'NONE',  ( -12.00000000000003908, -134.9999999999999716, -194.9999999999999432 ) ) ;
#4536=EDGE_CURVE ( 'NONE', #10851, #30170, #6457, .T. ) ;
#4537=ORIENTED_EDGE ( 'NONE', *, *, #19786, .T. ) ;
#4538=CARTESIAN_POINT ( 'NONE',  ( 11.99999999999999645, 112.9999999999999574, -175.0000000000000284 ) ) ;
#4540=EDGE_CURVE ( 'NONE', #11647, #18350, #21043, .T. ) ;
#4543=ADVANCED_FACE ( 'NONE', ( #12881 ), #13049, .F. ) ;
#4550=CARTESIAN_POINT ( 'NONE',  ( -365.0000000000000000, 134.9999999999999716, 113.9999999999999858 ) ) ;
#4554=ORIENTED_EDGE ( 'NONE', *, *, #20693, .F. ) ;
#4556=EDGE_LOOP ( 'NONE', ( #25851, #5534, #27281, #33332, #4770, #18880, #25460, #30973 ) ) ;
#4559=CARTESIAN_POINT ( 'NONE',  ( -414.0000000000000000, -105.0000000000000142, -77.99999999999997158 ) ) ;
#4564=PLANE ( 'NONE',  #3343 ) ;
#4570=LINE ( 'NONE', #32173, #8080 ) ;
#4573=EDGE_LOOP ( 'NONE', ( #30707, #29959, #6658, #26541 ) ) ;
#4578=CARTESIAN_POINT ( 'NONE',  ( -12.00000000000001066, -105.0000000000000142, -154.9999999999999716 ) ) ;
#4579=DIRECTION ( 'NONE',  ( -1.000000000000000000, 0.000000000000000000, -1.300283923313630633E-47 ) ) ;
#4580=EDGE_LOOP ( 'NONE', ( #17912, #11755, #20585, #14999 ) ) ;
#4583=ORIENTED_EDGE ( 'NONE', *, *, #32660, .T. ) ;
#4588=CARTESIAN_POINT ( 'NONE',  ( -19.99999999999998934, -145.0000000000000000, 162.9999999999999716 ) ) ;
#4594=CARTESIAN_POINT ( 'NONE',  ( -365.0000000000000000, 116.9999999999999716, 126.0000000000000000 ) ) ;
#4596=AXIS2_PLACEMENT_3D ( 'NONE', #7824, #18708, #7285 ) ;
#4603=AXIS2_PLACEMENT_3D ( 'NONE', #10156, #2144, #23505 ) ;
#4604=LINE ( 'NONE', #20659, #10217 ) ;
#4607=DIRECTION ( 'NONE',  ( 0.000000000000000000, 0.000000000000000000, -1.000000000000000000 ) ) ;
#4608=VERTEX_POINT ( 'NONE', #34937 ) ;
#4610=CARTESIAN_POINT ( 'NONE',  ( -19.99999999999998934, -105.0000000000000142, 187.0000000000000000 ) ) ;
#4613=CARTESIAN_POINT ( 'NONE',  ( -15.99999999999998579, -112.9999999999999858, 155.0000000000000000 ) ) ;
#4617=LINE ( 'NONE', #7126, #12199 ) ;
#4626=VERTEX_POINT ( 'NONE', #26381 ) ;
#4627=AXIS2_PLACEMENT_3D ( 'NONE', #33035, #22196, #11173 ) ;
#4629=AXIS2_PLACEMENT_3D ( 'NONE', #12094, #22590, #33433 ) ;
#4631=EDGE_LOOP ( 'NONE', ( #28245, #8824, #2541, #6678 ) ) ;
#4635=ORIENTED_EDGE ( 'NONE', *, *, #23749, .F. ) ;
#4636=ORIENTED_EDGE ( 'NONE', *, *, #4357, .T. ) ;
#4641=CARTESIAN_POINT ( 'NONE',  ( -70.00000000000000000, 4.559999999999908127, 168.2400000000000091 ) ) ;
#4642=DIRECTION ( 'NONE',  ( 1.000000000000000000, 0.000000000000000000, 0.000000000000000000 ) ) ;
#4643=ORIENTED_EDGE ( 'NONE', *, *, #8513, .T. ) ;
#4647=DIRECTION ( 'NONE',  ( -1.000000000000000000, 0.000000000000000000, -1.300283923313630633E-47 ) ) ;
#4651=VECTOR ( 'NONE', #18769, 1000.000000000000000 ) ;
#4652=FACE_OUTER_BOUND ( 'NONE', #16681, .T. ) ;
#4657=CARTESIAN_POINT ( 'NONE',  ( -347.0000000000000000, 124.9999999999999432, 181.0000000000000000 ) ) ;
#4658=DIRECTION ( 'NONE',  ( 0.000000000000000000, 2.309213040847544338E-50, 1.000000000000000000 ) ) ;
#4659=DIRECTION ( 'NONE',  ( 0.000000000000000000, 1.131431318426415506E-52, 1.000000000000000000 ) ) ;
#4662=EDGE_CURVE ( 'NONE', #10319, #4812, #22712, .T. ) ;
#4666=CARTESIAN_POINT ( 'NONE',  ( -12.00000000000001066, -24.99999999999999289, -175.0000000000000000 ) ) ;
#4675=VECTOR ( 'NONE', #25431, 1000.000000000000000 ) ;
#4677=AXIS2_PLACEMENT_3D ( 'NONE', #23089, #12062, #4011 ) ;
#4678=ORIENTED_EDGE ( 'NONE', *, *, #12906, .T. ) ;
#4679=CARTESIAN_POINT ( 'NONE',  ( -365.0000000000000000, 130.9999999999999716, 130.0000000000000000 ) ) ;
#4681=VERTEX_POINT ( 'NONE', #16603 ) ;
#4689=CARTESIAN_POINT ( 'NONE',  ( -430.0000000000000000, 116.9999999999999858, 126.0000000000000000 ) ) ;
#4691=LINE ( 'NONE', #2219, #17594 ) ;
#4692=LINE ( 'NONE', #17927, #32446 ) ;
#4696=AXIS2_PLACEMENT_3D ( 'NONE', #3279, #11480, #10779 ) ;
#4698=ORIENTED_EDGE ( 'NONE', *, *, #21804, .T. ) ;
#4701=FACE_OUTER_BOUND ( 'NONE', #21536, .T. ) ;
#4702=ORIENTED_EDGE ( 'NONE', *, *, #22566, .T. ) ;
#4707=MECHANICAL_DESIGN_GEOMETRIC_PRESENTATION_REPRESENTATION('',(#9832),#31919);
#4709=DIRECTION ( 'NONE',  ( 0.000000000000000000, -7.888609052210118054E-31, -1.000000000000000000 ) ) ;
#4715=CARTESIAN_POINT ( 'NONE',  ( -442.0000000000000000, -125.0000000000000000, 107.9999999999999858 ) ) ;
#4718=ADVANCED_FACE ( 'NONE', ( #33123 ), #213, .T. ) ;
#4719=ORIENTED_EDGE ( 'NONE', *, *, #20729, .T. ) ;
#4725=DIRECTION ( 'NONE',  ( 0.000000000000000000, 1.000000000000000000, -6.123233995736766036E-17 ) ) ;
#4732=CARTESIAN_POINT ( 'NONE',  ( -355.0000000000000000, -119.0000000000000000, 111.9999999999999858 ) ) ;
#4736=AXIS2_PLACEMENT_3D ( 'NONE', #34364, #31343, #20839 ) ;
#4744=DIRECTION ( 'NONE',  ( 0.000000000000000000, -1.000000000000000000, -2.465190328815662439E-32 ) ) ;
#4745=CARTESIAN_POINT ( 'NONE',  ( -19.99999999999998934, 112.9999999999999574, -175.0000000000000284 ) ) ;
#4750=ORIENTED_EDGE ( 'NONE', *, *, #29800, .F. ) ;
#4758=VECTOR ( 'NONE', #12896, 1000.000000000000000 ) ;
#4759=ORIENTED_EDGE ( 'NONE', *, *, #20854, .F. ) ;
#4764=VECTOR ( 'NONE', #18171, 1000.000000000000000 ) ;
#4765=ORIENTED_EDGE ( 'NONE', *, *, #31959, .T. ) ;
#4770=ORIENTED_EDGE ( 'NONE', *, *, #25156, .F. ) ;
#4771=ADVANCED_FACE ( 'NONE', ( #32417, #29758 ), #2699, .T. ) ;
#4772=DIRECTION ( 'NONE',  ( -1.000000000000000000, 0.000000000000000000, 1.848892746611746966E-32 ) ) ;
#4778=AXIS2_PLACEMENT_3D ( 'NONE', #31836, #9623, #31498 ) ;
#4779=DIRECTION ( 'NONE',  ( 5.546364386991661285E-52, 0.000000000000000000, -1.000000000000000000 ) ) ;
#4782=CIRCLE ( 'NONE', #820, 3.999999999999976019 ) ;
#4789=LINE ( 'NONE', #7644, #33510 ) ;
#4794=CARTESIAN_POINT ( 'NONE',  ( -499.9999999999999432, 140.9999999999999716, 162.9999999999999716 ) ) ;
#4797=DIRECTION ( 'NONE',  ( -1.000000000000000000, 0.000000000000000000, 0.000000000000000000 ) ) ;
#4798=EDGE_CURVE ( 'NONE', #26810, #3104, #397, .T. ) ;
#4801=CARTESIAN_POINT ( 'NONE',  ( 11.99999999999999645, 134.9999999999999432, -194.9999999999999432 ) ) ;
#4802=AXIS2_PLACEMENT_3D ( 'NONE', #18777, #15757, #8072 ) ;
#4803=EDGE_CURVE ( 'NONE', #4465, #21456, #4810, .T. ) ;
#4804=CARTESIAN_POINT ( 'NONE',  ( -20.00000000000007461, 108.9999999999999858, 162.9999999999999716 ) ) ;
#4809=VECTOR ( 'NONE', #8695, 1000.000000000000000 ) ;
#4810=CIRCLE ( 'NONE', #28891, 4.750000000000004441 ) ;
#4812=VERTEX_POINT ( 'NONE', #22807 ) ;
#4813=AXIS2_PLACEMENT_3D ( 'NONE', #3547, #25262, #897 ) ;
#4816=CLOSED_SHELL ( 'NONE', ( #15483, #17690, #8395, #26969, #9679, #14570, #11624, #26790, #13248, #11276, #29983, #23696, #11103, #2010, #4245, #17829, #16493, #17504 ) ) ;
#4820=ORIENTED_EDGE ( 'NONE', *, *, #31504, .F. ) ;
#4827=VERTEX_POINT ( 'NONE', #22983 ) ;
#4829=VECTOR ( 'NONE', #14017, 1000.000000000000000 ) ;
#4831=CIRCLE ( 'NONE', #35001, 3.999999999999976019 ) ;
#4834=CARTESIAN_POINT ( 'NONE',  ( -442.0000000000000000, -125.0000000000000000, 104.0000000000000142 ) ) ;
#4835=ORIENTED_EDGE ( 'NONE', *, *, #5450, .T. ) ;
#4838=DIRECTION ( 'NONE',  ( -0.000000000000000000, 0.000000000000000000, 1.000000000000000000 ) ) ;
#4839=ADVANCED_FACE ( 'NONE', ( #6412 ), #28143, .F. ) ;
#4846=DIRECTION ( 'NONE',  ( -1.000000000000000000, -3.040835319149746090E-31, 1.232595164407830946E-32 ) ) ;
#4848=FACE_OUTER_BOUND ( 'NONE', #18990, .T. ) ;
#4849=DIRECTION ( 'NONE',  ( 1.000000000000000000, -0.000000000000000000, -0.000000000000000000 ) ) ;
#4850=VERTEX_POINT ( 'NONE', #4088 ) ;
#4863=CARTESIAN_POINT ( 'NONE',  ( 19.99999999999998224, 112.9999999999999574, -155.0000000000000000 ) ) ;
#4864=VECTOR ( 'NONE', #34907, 1000.000000000000000 ) ;
#4865=CARTESIAN_POINT ( 'NONE',  ( -499.9999999999999432, 112.9999999999999574, -162.9999999999999716 ) ) ;
#4867=VERTEX_POINT ( 'NONE', #3919 ) ;
#4868=EDGE_LOOP ( 'NONE', ( #29614, #34580, #26910, #1631 ) ) ;
#4874=CARTESIAN_POINT ( 'NONE',  ( -430.0000000000000000, 130.9999999999999716, 113.9999999999999858 ) ) ;
#4875=UNCERTAINTY_MEASURE_WITH_UNIT (LENGTH_MEASURE( 1.000000000000000082E-05 ), #13910, 'distance_accuracy_value', 'NONE');
#4881=EDGE_LOOP ( 'NONE', ( #15001, #7925, #11194, #15897, #26891, #20999, #12021, #554 ) ) ;
#4882=EDGE_CURVE ( 'NONE', #20393, #32015, #7352, .T. ) ;
#4888=ORIENTED_EDGE ( 'NONE', *, *, #5873, .T. ) ;
#4892=CARTESIAN_POINT ( 'NONE',  ( -12.00000000000001066, -145.0000000000000000, -162.9999999999999432 ) ) ;
#4896=FACE_OUTER_BOUND ( 'NONE', #5351, .T. ) ;
#4913=ORIENTED_EDGE ( 'NONE', *, *, #34504, .F. ) ;
#4914=EDGE_LOOP ( 'NONE', ( #7192, #16179, #12089, #27858 ) ) ;
#4916=CARTESIAN_POINT ( 'NONE',  ( -499.9999999999999432, 112.9999999999999574, 187.0000000000000000 ) ) ;
#4919=ADVANCED_FACE ( 'NONE', ( #25818 ), #17314, .F. ) ;
#4922=CARTESIAN_POINT ( 'NONE',  ( 11.99999999999999645, 144.9999999999999716, -194.9999999999999432 ) ) ;
#4923=DIRECTION ( 'NONE',  ( 0.000000000000000000, -7.888609052210118054E-31, -1.000000000000000000 ) ) ;
#4927=VECTOR ( 'NONE', #5939, 1000.000000000000000 ) ;
#4928=LINE ( 'NONE', #15824, #10602 ) ;
#4930=CARTESIAN_POINT ( 'NONE',  ( -430.0000000000000000, 132.9999999999999716, 113.9999999999999858 ) ) ;
#4931=LINE ( 'NONE', #15828, #9784 ) ;
#4935=EDGE_CURVE ( 'NONE', #13888, #35039, #14638, .T. ) ;
#4936=EDGE_CURVE ( 'NONE', #25101, #3590, #25464, .T. ) ;
#4937=CARTESIAN_POINT ( 'NONE',  ( -15.99999999999998579, -112.9999999999999858, 174.9999999999999432 ) ) ;
#4939=DIRECTION ( 'NONE',  ( 0.000000000000000000, 0.000000000000000000, -1.000000000000000000 ) ) ;
#4940=EDGE_CURVE ( 'NONE', #4151, #11554, #10140, .T. ) ;
#4941=CARTESIAN_POINT ( 'NONE',  ( -12.00000000000001066, 124.9999999999999716, 155.0000000000000000 ) ) ;
#4943=CARTESIAN_POINT ( 'NONE',  ( -347.0000000000000000, 124.9999999999999432, 168.9999999999999716 ) ) ;
#4947=EDGE_LOOP ( 'NONE', ( #30164, #18875, #27210, #25641 ) ) ;
#4948=VERTEX_POINT ( 'NONE', #3570 ) ;
#4952=DIRECTION ( 'NONE',  ( 0.000000000000000000, 0.000000000000000000, -1.000000000000000000 ) ) ;
#4953=VECTOR ( 'NONE', #12007, 1000.000000000000000 ) ;
#4954=AXIS2_PLACEMENT_3D ( 'NONE', #11617, #22468, #8221 ) ;
#4955=PLANE ( 'NONE',  #33779 ) ;
#4959=VECTOR ( 'NONE', #18655, 1000.000000000000000 ) ;
#4961=DIRECTION ( 'NONE',  ( 0.000000000000000000, 0.000000000000000000, 1.000000000000000000 ) ) ;
#4965=ORIENTED_EDGE ( 'NONE', *, *, #31449, .F. ) ;
#4968=LINE ( 'NONE', #34895, #26777 ) ;
#4969=ORIENTED_EDGE ( 'NONE', *, *, #5430, .T. ) ;
#4971=VECTOR ( 'NONE', #29657, 1000.000000000000000 ) ;
#4972=EDGE_CURVE ( 'NONE', #34245, #11988, #16489, .T. ) ;
#4977=PLANE ( 'NONE',  #19993 ) ;
#4988=ORIENTED_EDGE ( 'NONE', *, *, #27834, .F. ) ;
#4995=EDGE_CURVE ( 'NONE', #1095, #10828, #4789, .T. ) ;
#4996=EDGE_CURVE ( 'NONE', #22138, #25172, #4604, .T. ) ;
#4998=ORIENTED_EDGE ( 'NONE', *, *, #21523, .T. ) ;
#4999=VERTEX_POINT ( 'NONE', #34708 ) ;
#5001=DIRECTION ( 'NONE',  ( 0.000000000000000000, -1.000000000000000000, 2.465190328815661892E-32 ) ) ;
#5006=EDGE_LOOP ( 'NONE', ( #30955, #3980, #29530, #11072 ) ) ;
#5008=DIRECTION ( 'NONE',  ( 0.000000000000000000, 1.310824597558155437E-49, 1.000000000000000000 ) ) ;
#5011=CARTESIAN_POINT ( 'NONE',  ( -355.0000000000000000, -131.0000000000000000, 111.9999999999999858 ) ) ;
#5013=ORIENTED_EDGE ( 'NONE', *, *, #28068, .F. ) ;
#5015=CARTESIAN_POINT ( 'NONE',  ( -355.0000000000000000, -131.0000000000000000, 109.9999999999999858 ) ) ;
#5017=LINE ( 'NONE', #18921, #19773 ) ;
#5019=DIRECTION ( 'NONE',  ( 0.000000000000000000, 0.000000000000000000, 1.000000000000000000 ) ) ;
#5020=CARTESIAN_POINT ( 'NONE',  ( -442.0000000000000000, -137.0000000000000000, 154.9999999999999716 ) ) ;
#5021=VECTOR ( 'NONE', #22943, 1000.000000000000000 ) ;
#5022=CARTESIAN_POINT ( 'NONE',  ( -430.0000000000000000, 118.9999999999999716, 113.9999999999999858 ) ) ;
#5024=DIRECTION ( 'NONE',  ( 0.000000000000000000, 1.131431318426415506E-52, 1.000000000000000000 ) ) ;
#5025=AXIS2_PLACEMENT_3D ( 'NONE', #735, #11785, #19958 ) ;
#5026=LINE ( 'NONE', #7342, #3627 ) ;
#5027=VERTEX_POINT ( 'NONE', #34532 ) ;
#5028=DIRECTION ( 'NONE',  ( -1.000000000000000000, 0.000000000000000000, -5.546364386991661285E-52 ) ) ;
#5030=DIRECTION ( 'NONE',  ( 1.000000000000000000, 0.000000000000000000, 1.300283923313630633E-47 ) ) ;
#5031=CIRCLE ( 'NONE', #3338, 3.999999999999976019 ) ;
#5036=AXIS2_PLACEMENT_3D ( 'NONE', #2438, #32687, #10641 ) ;
#5041=VERTEX_POINT ( 'NONE', #34894 ) ;
#5042=ORIENTED_EDGE ( 'NONE', *, *, #32400, .T. ) ;
#5043=CARTESIAN_POINT ( 'NONE',  ( -442.0000000000000000, -105.0000000000000142, -155.0000000000000000 ) ) ;
#5044=AXIS2_PLACEMENT_3D ( 'NONE', #28411, #22896, #17227 ) ;
#5045=DIRECTION ( 'NONE',  ( 0.000000000000000000, 0.000000000000000000, 1.000000000000000000 ) ) ;
#5046=PLANE ( 'NONE',  #2878 ) ;
#5050=DIRECTION ( 'NONE',  ( 0.000000000000000000, 0.000000000000000000, -1.000000000000000000 ) ) ;
#5056=DIRECTION ( 'NONE',  ( -0.000000000000000000, -1.000000000000000000, -0.000000000000000000 ) ) ;
#5057=CARTESIAN_POINT ( 'NONE',  ( -361.0000000000000000, -125.0000000000000284, 168.9999999999999716 ) ) ;
#5058=ORIENTED_EDGE ( 'NONE', *, *, #5207, .T. ) ;
#5059=CARTESIAN_POINT ( 'NONE',  ( -20.00000000000004619, -137.0000000000000000, -187.0000000000000000 ) ) ;
#5060=CARTESIAN_POINT ( 'NONE',  ( -500.0000000000000000, -113.0000000000000000, 190.9999999999999716 ) ) ;
#5062=ORIENTED_EDGE ( 'NONE', *, *, #231, .F. ) ;
#5065=ORIENTED_EDGE ( 'NONE', *, *, #18741, .T. ) ;
#5066=DIRECTION ( 'NONE',  ( 0.000000000000000000, 1.000000000000000000, 1.224646799147353207E-16 ) ) ;
#5067=ORIENTED_EDGE ( 'NONE', *, *, #25008, .F. ) ;
#5069=CYLINDRICAL_SURFACE ( 'NONE', #28493, 3.999999999999948042 ) ;
#5071=DIRECTION ( 'NONE',  ( 0.000000000000000000, -1.000000000000000000, -1.310824597558155437E-49 ) ) ;
#5078=EDGE_CURVE ( 'NONE', #12986, #23261, #18354, .T. ) ;
#5083=ADVANCED_FACE ( 'NONE', ( #23846 ), #31673, .F. ) ;
#5087=VECTOR ( 'NONE', #12336, 1000.000000000000000 ) ;
#5088=LINE ( 'NONE', #2081, #10772 ) ;
#5092=EDGE_LOOP ( 'NONE', ( #2806, #13100, #2462, #10252 ) ) ;
#5094=FACE_OUTER_BOUND ( 'NONE', #13253, .T. ) ;
#5098=CARTESIAN_POINT ( 'NONE',  ( -361.0000000000000000, 124.9999999999999432, 164.9999999999999716 ) ) ;
#5101=DIRECTION ( 'NONE',  ( -0.000000000000000000, -1.000000000000000000, -0.000000000000000000 ) ) ;
#5107=CARTESIAN_POINT ( 'NONE',  ( -12.00000000000001066, 144.9999999999999716, 187.0000000000000000 ) ) ;
#5108=EDGE_LOOP ( 'NONE', ( #34830, #16296, #32852, #25071 ) ) ;
#5117=LINE ( 'NONE', #26844, #12069 ) ;
#5123=EDGE_CURVE ( 'NONE', #30715, #6277, #24412, .T. ) ;
#5126=CARTESIAN_POINT ( 'NONE',  ( -442.0000000000000000, 105.0000000000000000, -69.99999999999998579 ) ) ;
#5128=DIRECTION ( 'NONE',  ( 0.000000000000000000, 7.888609052210118054E-31, 1.000000000000000000 ) ) ;
#5129=ADVANCED_FACE ( 'NONE', ( #24719 ), #530, .T. ) ;
#5131=CIRCLE ( 'NONE', #11487, 7.999999999999979572 ) ;
#5135=EDGE_CURVE ( 'NONE', #22985, #26377, #26123, .T. ) ;
#5138=ORIENTED_EDGE ( 'NONE', *, *, #2842, .F. ) ;
#5142=DIRECTION ( 'NONE',  ( 0.000000000000000000, 1.000000000000000000, -6.123233995736766036E-17 ) ) ;
#5144=ORIENTED_EDGE ( 'NONE', *, *, #15905, .T. ) ;
#5145=PLANE ( 'NONE',  #7264 ) ;
#5149=ORIENTED_EDGE ( 'NONE', *, *, #28007, .T. ) ;
#5151=CARTESIAN_POINT ( 'NONE',  ( -500.0000000000000000, -141.0000000000000000, 187.0000000000000000 ) ) ;
#5152=CARTESIAN_POINT ( 'NONE',  ( -418.0000000000000000, 124.9999999999999432, -155.0000000000000000 ) ) ;
#5153=CARTESIAN_POINT ( 'NONE',  ( -12.00000000000001066, -141.0000000000000000, 155.0000000000000000 ) ) ;
#5157=LINE ( 'NONE', #13375, #26881 ) ;
#5162=ORIENTED_EDGE ( 'NONE', *, *, #6706, .F. ) ;
#5163=ORIENTED_EDGE ( 'NONE', *, *, #5759, .T. ) ;
#5165=VECTOR ( 'NONE', #5319, 1000.000000000000000 ) ;
#5166=EDGE_CURVE ( 'NONE', #34985, #30302, #27187, .T. ) ;
#5172=DIRECTION ( 'NONE',  ( 1.300283923313630633E-47, 0.000000000000000000, 1.000000000000000000 ) ) ;
#5175=VERTEX_POINT ( 'NONE', #355 ) ;
#5182=CARTESIAN_POINT ( 'NONE',  ( -12.00000000000001066, -124.9999999999999432, -154.9999999999999716 ) ) ;
#5183=EDGE_LOOP ( 'NONE', ( #28428, #12778, #10898, #34241, #29681, #32616, #19948, #11191 ) ) ;
#5184=CIRCLE ( 'NONE', #13745, 3.999999999999976019 ) ;
#5185=CARTESIAN_POINT ( 'NONE',  ( -15.99999999999998579, -124.9999999999999432, -162.9999999999999432 ) ) ;
#5187=DIRECTION ( 'NONE',  ( 1.000000000000000000, 0.000000000000000000, 0.000000000000000000 ) ) ;
#5193=EDGE_CURVE ( 'NONE', #3477, #16642, #15856, .T. ) ;
#5195=AXIS2_PLACEMENT_3D ( 'NONE', #9194, #20067, #17583 ) ;
#5198=EDGE_LOOP ( 'NONE', ( #21138, #11714, #13499, #26497 ) ) ;
#5199=CIRCLE ( 'NONE', #14338, 7.999999999999952038 ) ;
#5200=LINE ( 'NONE', #7520, #29707 ) ;
#5201=DIRECTION ( 'NONE',  ( 1.000000000000000000, 0.000000000000000000, -1.848892746611746966E-32 ) ) ;
#5202=ORIENTED_EDGE ( 'NONE', *, *, #16240, .T. ) ;
#5203=DIRECTION ( 'NONE',  ( 1.000000000000000000, 0.000000000000000000, 0.000000000000000000 ) ) ;
#5205=CIRCLE ( 'NONE', #23420, 4.000000000000003553 ) ;
#5207=EDGE_CURVE ( 'NONE', #22615, #28417, #2831, .T. ) ;
#5208=VERTEX_POINT ( 'NONE', #2480 ) ;
#5211=ORIENTED_EDGE ( 'NONE', *, *, #21013, .F. ) ;
#5214=VECTOR ( 'NONE', #22208, 1000.000000000000000 ) ;
#5227=ORIENTED_EDGE ( 'NONE', *, *, #29984, .F. ) ;
#5228=DIRECTION ( 'NONE',  ( 5.546364386991661285E-52, 0.000000000000000000, 1.000000000000000000 ) ) ;
#5234=VERTEX_POINT ( 'NONE', #29718 ) ;
#5235=EDGE_CURVE ( 'NONE', #25895, #5645, #5318, .T. ) ;
#5241=EDGE_CURVE ( 'NONE', #32323, #33070, #14144, .T. ) ;
#5243=EDGE_CURVE ( 'NONE', #22914, #29991, #19756, .T. ) ;
#5244=CIRCLE ( 'NONE', #25143, 7.999999999999979572 ) ;
#5246=VECTOR ( 'NONE', #21760, 1000.000000000000000 ) ;
#5247=VECTOR ( 'NONE', #28936, 1000.000000000000000 ) ;
#5249=ADVANCED_FACE ( 'NONE', ( #6561 ), #1228, .F. ) ;
#5254=LINE ( 'NONE', #8468, #13620 ) ;
#5256=FACE_OUTER_BOUND ( 'NONE', #27990, .T. ) ;
#5257=( LENGTH_UNIT ( ) NAMED_UNIT ( * ) SI_UNIT ( .MILLI., .METRE. ) );
#5259=DIRECTION ( 'NONE',  ( 0.000000000000000000, 0.000000000000000000, 1.000000000000000000 ) ) ;
#5260=ORIENTED_EDGE ( 'NONE', *, *, #21334, .F. ) ;
#5263=CARTESIAN_POINT ( 'NONE',  ( 11.99999999999995559, -134.9999999999999716, -186.9999999999999716 ) ) ;
#5267=CARTESIAN_POINT ( 'NONE',  ( -19.99999999999998934, -134.9999999999999716, 187.0000000000000000 ) ) ;
#5269=FACE_OUTER_BOUND ( 'NONE', #10633, .T. ) ;
#5275=LINE ( 'NONE', #35030, #6177 ) ;
#5276=ORIENTED_EDGE ( 'NONE', *, *, #25205, .T. ) ;
#5277=ADVANCED_FACE ( 'NONE', ( #19578 ), #19926, .F. ) ;
#5284=DIRECTION ( 'NONE',  ( -0.000000000000000000, 2.465190328815661892E-32, 1.000000000000000000 ) ) ;
#5285=ORIENTED_EDGE ( 'NONE', *, *, #15353, .T. ) ;
#5288=CIRCLE ( 'NONE', #11570, 3.999999999999976019 ) ;
#5292=DIRECTION ( 'NONE',  ( 0.000000000000000000, -1.000000000000000000, -0.000000000000000000 ) ) ;
#5293=ORIENTED_EDGE ( 'NONE', *, *, #6404, .T. ) ;
#5308=ORIENTED_EDGE ( 'NONE', *, *, #22945, .F. ) ;
#5313=ORIENTED_EDGE ( 'NONE', *, *, #33547, .F. ) ;
#5318=LINE ( 'NONE', #28286, #499 ) ;
#5319=DIRECTION ( 'NONE',  ( 1.000000000000000000, 0.000000000000000000, 0.000000000000000000 ) ) ;
#5323=CARTESIAN_POINT ( 'NONE',  ( -442.0000000000000000, -124.9999999999999858, -77.99999999999997158 ) ) ;
#5324=EDGE_CURVE ( 'NONE', #13597, #14760, #27745, .T. ) ;
#5328=FACE_OUTER_BOUND ( 'NONE', #14914, .T. ) ;
#5330=ADVANCED_FACE ( 'NONE', ( #25062 ), #30952, .T. ) ;
#5336=CARTESIAN_POINT ( 'NONE',  ( -19.99999999999998934, -137.0000000000000000, 190.9999999999999716 ) ) ;
#5338=EDGE_CURVE ( 'NONE', #24819, #19022, #22414, .T. ) ;
#5341=CARTESIAN_POINT ( 'NONE',  ( -442.0000000000000000, -105.0000000000000142, -101.9999999999999858 ) ) ;
#5345=ORIENTED_EDGE ( 'NONE', *, *, #25188, .F. ) ;
#5346=DIRECTION ( 'NONE',  ( 1.000000000000000000, 0.000000000000000000, -1.232595164407831220E-32 ) ) ;
#5351=EDGE_LOOP ( 'NONE', ( #30007, #2306, #13825, #13245 ) ) ;
#5353=CIRCLE ( 'NONE', #6481, 7.999999999999979572 ) ;
#5356=ORIENTED_EDGE ( 'NONE', *, *, #5609, .F. ) ;
#5357=DIRECTION ( 'NONE',  ( 0.000000000000000000, 0.000000000000000000, 1.000000000000000000 ) ) ;
#5359=EDGE_CURVE ( 'NONE', #29676, #19146, #17090, .T. ) ;
#5360=DIRECTION ( 'NONE',  ( 1.000000000000000000, -8.433758354584418579E-81, 1.232595164407830946E-32 ) ) ;
#5366=AXIS2_PLACEMENT_3D ( 'NONE', #29617, #5396, #18950 ) ;
#5372=EDGE_CURVE ( 'NONE', #6316, #2726, #24465, .T. ) ;
#5379=EDGE_CURVE ( 'NONE', #21471, #11116, #22611, .T. ) ;
#5382=VERTEX_POINT ( 'NONE', #13813 ) ;
#5384=CARTESIAN_POINT ( 'NONE',  ( -19.99999999999998934, 144.9999999999999147, 162.9999999999999716 ) ) ;
#5392=EDGE_LOOP ( 'NONE', ( #22412, #4965, #27605, #29640 ) ) ;
#5393=PLANE ( 'NONE',  #239 ) ;
#5396=DIRECTION ( 'NONE',  ( 0.000000000000000000, -1.000000000000000000, 6.123233995736766036E-17 ) ) ;
#5397=AXIS2_PLACEMENT_3D ( 'NONE', #2609, #13480, #24318 ) ;
#5398=DIRECTION ( 'NONE',  ( 0.000000000000000000, 1.000000000000000000, 1.224646799147353207E-16 ) ) ;
#5399=CARTESIAN_POINT ( 'NONE',  ( -15.99999999999998579, 75.55999999999990280, -177.7400000000000091 ) ) ;
#5400=VERTEX_POINT ( 'NONE', #16145 ) ;
#5402=AXIS2_PLACEMENT_3D ( 'NONE', #3684, #8855, #33411 ) ;
#5405=STYLED_ITEM('',(#35254),#100);
#5410=PLANE ( 'NONE',  #30667 ) ;
#5412=LINE ( 'NONE', #21277, #15665 ) ;
#5413=DIRECTION ( 'NONE',  ( 0.000000000000000000, 7.888609052210118054E-31, 1.000000000000000000 ) ) ;
#5414=LINE ( 'NONE', #32645, #3008 ) ;
#5416=VERTEX_POINT ( 'NONE', #19335 ) ;
#5417=CIRCLE ( 'NONE', #7674, 3.999999999999976019 ) ;
#5421=ORIENTED_EDGE ( 'NONE', *, *, #19538, .T. ) ;
#5422=DIRECTION ( 'NONE',  ( -3.469446951953832974E-18, -1.000000000000000000, -7.888609052210116302E-31 ) ) ;
#5423=AXIS2_PLACEMENT_3D ( 'NONE', #25512, #4838, #20707 ) ;
#5424=LINE ( 'NONE', #26796, #17129 ) ;
#5425=ORIENTED_EDGE ( 'NONE', *, *, #18757, .F. ) ;
#5430=EDGE_CURVE ( 'NONE', #31108, #13597, #16673, .T. ) ;
#5434=VERTEX_POINT ( 'NONE', #22351 ) ;
#5436=DIRECTION ( 'NONE',  ( 0.000000000000000000, 0.000000000000000000, -1.000000000000000000 ) ) ;
#5441=VECTOR ( 'NONE', #26421, 1000.000000000000000 ) ;
#5443=DIRECTION ( 'NONE',  ( 0.000000000000000000, 0.000000000000000000, 1.000000000000000000 ) ) ;
#5444=ORIENTED_EDGE ( 'NONE', *, *, #8008, .F. ) ;
#5447=DIRECTION ( 'NONE',  ( 0.000000000000000000, 0.000000000000000000, -1.000000000000000000 ) ) ;
#5448=CARTESIAN_POINT ( 'NONE',  ( -12.00000000000001066, 124.9999999999999716, 155.0000000000000000 ) ) ;
#5449=AXIS2_PLACEMENT_3D ( 'NONE', #24323, #11060, #18497 ) ;
#5450=EDGE_CURVE ( 'NONE', #4470, #27012, #2941, .T. ) ;
#5451=CARTESIAN_POINT ( 'NONE',  ( -20.00000000000007461, -109.0000000000000142, -187.0000000000000000 ) ) ;
#5452=DIRECTION ( 'NONE',  ( -1.292961597001347186E-16, 0.000000000000000000, 1.000000000000000000 ) ) ;
#5454=LINE ( 'NONE', #2787, #11229 ) ;
#5457=CIRCLE ( 'NONE', #28213, 3.999999999999976019 ) ;
#5459=CARTESIAN_POINT ( 'NONE',  ( -12.00000000000001066, -124.9999999999999432, -186.9999999999999716 ) ) ;
#5465=ORIENTED_EDGE ( 'NONE', *, *, #22209, .F. ) ;
#5476=DIRECTION ( 'NONE',  ( -1.000000000000000000, 0.000000000000000000, -1.300283923313630633E-47 ) ) ;
#5477=EDGE_LOOP ( 'NONE', ( #32552, #10131, #15350, #5421 ) ) ;
#5480=EDGE_CURVE ( 'NONE', #13630, #18484, #19768, .T. ) ;
#5485=EDGE_LOOP ( 'NONE', ( #33883, #463, #4459, #12787, #9206, #9659 ) ) ;
#5486=CARTESIAN_POINT ( 'NONE',  ( -355.0000000000000000, -131.0000000000000000, 126.0000000000000000 ) ) ;
#5488=CARTESIAN_POINT ( 'NONE',  ( -418.0000000000000568, -105.0000000000000142, 100.0000000000000000 ) ) ;
#5489=VECTOR ( 'NONE', #22593, 1000.000000000000000 ) ;
#5491=EDGE_LOOP ( 'NONE', ( #3395, #33863, #30225, #21326 ) ) ;
#5492=ORIENTED_EDGE ( 'NONE', *, *, #23666, .F. ) ;
#5493=CARTESIAN_POINT ( 'NONE',  ( -361.0000000000000000, 134.9999999999999716, 110.0000000000000000 ) ) ;
#5495=CARTESIAN_POINT ( 'NONE',  ( -418.0000000000000000, 105.0000000000000000, 132.0000000000000000 ) ) ;
#5496=CARTESIAN_POINT ( 'NONE',  ( -12.00000000000001066, 144.9999999999999716, -186.9999999999999716 ) ) ;
#5497=ORIENTED_EDGE ( 'NONE', *, *, #4162, .F. ) ;
#5502=LINE ( 'NONE', #32743, #3291 ) ;
#5504=DIRECTION ( 'NONE',  ( 0.000000000000000000, -1.000000000000000000, -2.465190328815662439E-32 ) ) ;
#5507=CARTESIAN_POINT ( 'NONE',  ( -70.00000000000000000, 75.55999999999990280, -172.9900000000000091 ) ) ;
#5509=AXIS2_PLACEMENT_3D ( 'NONE', #14246, #9067, #22420 ) ;
#5510=VECTOR ( 'NONE', #5792, 1000.000000000000000 ) ;
#5511=CIRCLE ( 'NONE', #2121, 7.999999999999979572 ) ;
#5513=CARTESIAN_POINT ( 'NONE',  ( 12.00000000000003908, -55.00000000000000711, -158.9999999999999716 ) ) ;
#5516=EDGE_LOOP ( 'NONE', ( #5786, #23663, #33910, #4036 ) ) ;
#5518=EDGE_CURVE ( 'NONE', #12319, #2702, #25436, .T. ) ;
#5520=ORIENTED_EDGE ( 'NONE', *, *, #6405, .F. ) ;
#5521=ADVANCED_FACE ( 'NONE', ( #6502 ), #23247, .T. ) ;
#5534=ORIENTED_EDGE ( 'NONE', *, *, #26429, .F. ) ;
#5535=CARTESIAN_POINT ( 'NONE',  ( -430.0000000000000000, 130.9999999999999716, 126.0000000000000000 ) ) ;
#5536=AXIS2_PLACEMENT_3D ( 'NONE', #7872, #21407, #21746 ) ;
#5540=DIRECTION ( 'NONE',  ( -1.000000000000000000, 0.000000000000000000, 0.000000000000000000 ) ) ;
#5541=FACE_OUTER_BOUND ( 'NONE', #11820, .T. ) ;
#5543=CARTESIAN_POINT ( 'NONE',  ( -418.0000000000000000, 105.0000000000000000, -73.99999999999998579 ) ) ;
#5545=FACE_OUTER_BOUND ( 'NONE', #20152, .T. ) ;
#5547=CARTESIAN_POINT ( 'NONE',  ( -499.9999999999999432, 144.9999999999999716, 187.0000000000000000 ) ) ;
#5549=DIRECTION ( 'NONE',  ( 0.000000000000000000, -1.000000000000000000, -3.374343856708137958E-53 ) ) ;
#5555=AXIS2_PLACEMENT_3D ( 'NONE', #22263, #8726, #6044 ) ;
#5557=VECTOR ( 'NONE', #11203, 1000.000000000000000 ) ;
#5559=CARTESIAN_POINT ( 'NONE',  ( -442.0000000000000000, -105.0000000000000142, -174.9999999999999716 ) ) ;
#5562=ADVANCED_FACE ( 'NONE', ( #25373 ), #33920, .T. ) ;
#5563=CARTESIAN_POINT ( 'NONE',  ( -442.0000000000000000, -112.9999999999999858, -155.0000000000000000 ) ) ;
#5565=DIRECTION ( 'NONE',  ( 0.000000000000000000, 0.000000000000000000, 1.000000000000000000 ) ) ;
#5567=ORIENTED_EDGE ( 'NONE', *, *, #20376, .F. ) ;
#5568=EDGE_CURVE ( 'NONE', #19338, #13474, #34088, .T. ) ;
#5575=ORIENTED_EDGE ( 'NONE', *, *, #17635, .T. ) ;
#5577=CARTESIAN_POINT ( 'NONE',  ( -499.9999999999999432, 112.9999999999999574, 155.0000000000000000 ) ) ;
#5580=ORIENTED_EDGE ( 'NONE', *, *, #30823, .F. ) ;
#5582=DIRECTION ( 'NONE',  ( 0.000000000000000000, -1.000000000000000000, -2.465190328815662439E-32 ) ) ;
#5586=AXIS2_PLACEMENT_3D ( 'NONE', #15098, #18300, #1898 ) ;
#5593=VERTEX_POINT ( 'NONE', #11876 ) ;
#5594=CARTESIAN_POINT ( 'NONE',  ( -347.0000000000000000, 124.9999999999999432, 181.0000000000000000 ) ) ;
#5595=DIRECTION ( 'NONE',  ( 0.000000000000000000, 0.000000000000000000, 1.000000000000000000 ) ) ;
#5596=ORIENTED_EDGE ( 'NONE', *, *, #11618, .F. ) ;
#5597=CIRCLE ( 'NONE', #24946, 7.999999999999992895 ) ;
#5598=ORIENTED_EDGE ( 'NONE', *, *, #34641, .T. ) ;
#5599=CARTESIAN_POINT ( 'NONE',  ( -499.9999999999999432, 108.9999999999999858, 162.9999999999999716 ) ) ;
#5600=LINE ( 'NONE', #35010, #28957 ) ;
#5601=ORIENTED_EDGE ( 'NONE', *, *, #31868, .T. ) ;
#5602=ORIENTED_EDGE ( 'NONE', *, *, #3405, .F. ) ;
#5603=DIRECTION ( 'NONE',  ( 1.000000000000000000, 0.000000000000000000, 0.000000000000000000 ) ) ;
#5604=EDGE_CURVE ( 'NONE', #7246, #29898, #14547, .T. ) ;
#5605=CARTESIAN_POINT ( 'NONE',  ( -355.0000000000000000, -135.0000000000000000, 126.0000000000000000 ) ) ;
#5609=EDGE_CURVE ( 'NONE', #11612, #24525, #28749, .T. ) ;
#5610=EDGE_LOOP ( 'NONE', ( #21331, #15365, #15943, #18376 ) ) ;
#5611=EDGE_CURVE ( 'NONE', #16642, #5950, #25729, .T. ) ;
#5614=CARTESIAN_POINT ( 'NONE',  ( -500.0000000000000000, -113.0000000000000000, 162.9999999999999716 ) ) ;
#5619=LINE ( 'NONE', #21658, #32253 ) ;
#5621=ORIENTED_EDGE ( 'NONE', *, *, #24211, .T. ) ;
#5625=DIRECTION ( 'NONE',  ( 1.848892746611746419E-32, 6.842277657836020854E-49, -1.000000000000000000 ) ) ;
#5626=ORIENTED_EDGE ( 'NONE', *, *, #10438, .F. ) ;
#5628=CARTESIAN_POINT ( 'NONE',  ( -70.00000000000000000, 75.55999999999990280, 172.9900000000000091 ) ) ;
#5630=FACE_OUTER_BOUND ( 'NONE', #3355, .T. ) ;
#5635=ORIENTED_EDGE ( 'NONE', *, *, #13751, .F. ) ;
#5636=DIRECTION ( 'NONE',  ( -1.000000000000000000, 0.000000000000000000, 0.000000000000000000 ) ) ;
#5639=EDGE_CURVE ( 'NONE', #26315, #22871, #14895, .T. ) ;
#5641=VECTOR ( 'NONE', #9485, 1000.000000000000000 ) ;
#5645=VERTEX_POINT ( 'NONE', #1355 ) ;
#5649=PLANE ( 'NONE',  #8796 ) ;
#5652=ADVANCED_FACE ( 'NONE', ( #8388 ), #13088, .F. ) ;
#5659=DIRECTION ( 'NONE',  ( 0.000000000000000000, 0.000000000000000000, 1.000000000000000000 ) ) ;
#5661=EDGE_LOOP ( 'NONE', ( #21149, #5062 ) ) ;
#5662=CARTESIAN_POINT ( 'NONE',  ( -499.9999999999999432, -137.0000000000000000, -162.9999999999999716 ) ) ;
#5663=ORIENTED_EDGE ( 'NONE', *, *, #28958, .F. ) ;
#5669=FACE_OUTER_BOUND ( 'NONE', #4573, .T. ) ;
#5670=CARTESIAN_POINT ( 'NONE',  ( -19.99999999999998934, -124.9999999999999432, -162.9999999999999432 ) ) ;
#5672=FACE_OUTER_BOUND ( 'NONE', #17156, .T. ) ;
#5673=CARTESIAN_POINT ( 'NONE',  ( -499.9999999999999432, 136.9999999999999432, 187.0000000000000000 ) ) ;
#5675=EDGE_CURVE ( 'NONE', #12264, #29470, #27699, .T. ) ;
#5677=EDGE_CURVE ( 'NONE', #30602, #21957, #20746, .T. ) ;
#5679=CARTESIAN_POINT ( 'NONE',  ( 15.99999999999998579, 4.559999999999908127, 172.9900000000000091 ) ) ;
#5680=( NAMED_UNIT ( * ) SI_UNIT ( $, .STERADIAN. ) SOLID_ANGLE_UNIT ( ) );
#5681=EDGE_CURVE ( 'NONE', #24390, #7431, #1562, .T. ) ;
#5682=VERTEX_POINT ( 'NONE', #30102 ) ;
#5685=ADVANCED_FACE ( 'NONE', ( #26246 ), #32763, .F. ) ;
#5686=ORIENTED_EDGE ( 'NONE', *, *, #19932, .F. ) ;
#5687=EDGE_LOOP ( 'NONE', ( #9570, #28, #3639, #21966, #13053, #19672, #1830, #5732 ) ) ;
#5693=DIRECTION ( 'NONE',  ( 0.000000000000000000, -1.000000000000000000, -1.131431318426415506E-52 ) ) ;
#5700=DIRECTION ( 'NONE',  ( -1.000000000000000000, 0.000000000000000000, -1.300283923313630633E-47 ) ) ;
#5706=DIRECTION ( 'NONE',  ( 1.000000000000000000, 0.000000000000000000, 1.300283923313630633E-47 ) ) ;
#5707=LINE ( 'NONE', #8746, #14008 ) ;
#5711=EDGE_CURVE ( 'NONE', #15141, #10000, #31677, .T. ) ;
#5720=EDGE_LOOP ( 'NONE', ( #19462, #17581 ) ) ;
#5721=CARTESIAN_POINT ( 'NONE',  ( 12.00000000000001066, -64.99999999999997158, 154.9999999999999716 ) ) ;
#5724=VECTOR ( 'NONE', #6985, 1000.000000000000000 ) ;
#5725=DIRECTION ( 'NONE',  ( 0.000000000000000000, -1.000000000000000000, 0.000000000000000000 ) ) ;
#5726=AXIS2_PLACEMENT_3D ( 'NONE', #23307, #1757, #12631 ) ;
#5732=ORIENTED_EDGE ( 'NONE', *, *, #34314, .T. ) ;
#5733=CIRCLE ( 'NONE', #28502, 7.999999999999952038 ) ;
#5734=DIRECTION ( 'NONE',  ( 0.000000000000000000, 0.000000000000000000, 1.000000000000000000 ) ) ;
#5736=CYLINDRICAL_SURFACE ( 'NONE', #33979, 7.999999999999979572 ) ;
#5745=CARTESIAN_POINT ( 'NONE',  ( -19.99999999999998934, -137.0000000000000000, 159.0000000000000000 ) ) ;
#5747=DIRECTION ( 'NONE',  ( 0.000000000000000000, 0.000000000000000000, 1.000000000000000000 ) ) ;
#5749=VECTOR ( 'NONE', #34288, 1000.000000000000000 ) ;
#5750=EDGE_CURVE ( 'NONE', #27942, #29489, #23002, .T. ) ;
#5755=EDGE_CURVE ( 'NONE', #3590, #7140, #27252, .T. ) ;
#5756=DIRECTION ( 'NONE',  ( -0.000000000000000000, 1.000000000000000000, -0.000000000000000000 ) ) ;
#5757=CARTESIAN_POINT ( 'NONE',  ( -365.0000000000000000, -117.0000000000000000, 113.9999999999999858 ) ) ;
#5758=ORIENTED_EDGE ( 'NONE', *, *, #25395, .T. ) ;
#5759=EDGE_CURVE ( 'NONE', #18227, #25758, #31927, .T. ) ;
#5760=LINE ( 'NONE', #19500, #13854 ) ;
#5764=( LENGTH_UNIT ( ) NAMED_UNIT ( * ) SI_UNIT ( .MILLI., .METRE. ) );
#5765=ORIENTED_EDGE ( 'NONE', *, *, #11059, .T. ) ;
#5771=VERTEX_POINT ( 'NONE', #1862 ) ;
#5772=ORIENTED_EDGE ( 'NONE', *, *, #11104, .F. ) ;
#5775=VERTEX_POINT ( 'NONE', #34442 ) ;
#5779=ORIENTED_EDGE ( 'NONE', *, *, #32383, .F. ) ;
#5780=VECTOR ( 'NONE', #19721, 1000.000000000000000 ) ;
#5781=DIRECTION ( 'NONE',  ( -1.000000000000000000, 0.000000000000000000, 0.000000000000000000 ) ) ;
#5782=CARTESIAN_POINT ( 'NONE',  ( 11.99999999999999645, -124.9999999999999432, -154.9999999999999716 ) ) ;
#5786=ORIENTED_EDGE ( 'NONE', *, *, #3909, .F. ) ;
#5787=CARTESIAN_POINT ( 'NONE',  ( -414.0000000000000568, -124.9999999999999716, 132.0000000000000000 ) ) ;
#5788=LINE ( 'NONE', #120, #1038 ) ;
#5790=DIRECTION ( 'NONE',  ( 0.000000000000000000, 0.000000000000000000, -1.000000000000000000 ) ) ;
#5792=DIRECTION ( 'NONE',  ( -0.000000000000000000, -1.000000000000000000, -0.000000000000000000 ) ) ;
#5794=VERTEX_POINT ( 'NONE', #4689 ) ;
#5795=DIRECTION ( 'NONE',  ( 1.000000000000000000, 3.040835319149746090E-31, 1.232595164407830946E-32 ) ) ;
#5796=LINE ( 'NONE', #27178, #27948 ) ;
#5797=EDGE_CURVE ( 'NONE', #8817, #11568, #19023, .T. ) ;
#5800=EDGE_LOOP ( 'NONE', ( #421, #10683, #17475, #32735 ) ) ;
#5803=AXIS2_PLACEMENT_3D ( 'NONE', #2543, #21595, #18935 ) ;
#5804=AXIS2_PLACEMENT_3D ( 'NONE', #13621, #11134, #32299 ) ;
#5810=EDGE_CURVE ( 'NONE', #6974, #18838, #5926, .T. ) ;
#5811=ORIENTED_EDGE ( 'NONE', *, *, #12501, .T. ) ;
#5817=ORIENTED_EDGE ( 'NONE', *, *, #23141, .F. ) ;
#5821=DIRECTION ( 'NONE',  ( 1.000000000000000000, 0.000000000000000000, -0.000000000000000000 ) ) ;
#5824=DIRECTION ( 'NONE',  ( -1.000000000000000000, 0.000000000000000000, 0.000000000000000000 ) ) ;
#5825=CIRCLE ( 'NONE', #10390, 3.999999999999976019 ) ;
#5832=ORIENTED_EDGE ( 'NONE', *, *, #29290, .F. ) ;
#5835=EDGE_CURVE ( 'NONE', #17427, #22841, #25836, .T. ) ;
#5836=LINE ( 'NONE', #33076, #4809 ) ;
#5837=EDGE_CURVE ( 'NONE', #10851, #18104, #16955, .T. ) ;
#5838=VERTEX_POINT ( 'NONE', #914 ) ;
#5839=ORIENTED_EDGE ( 'NONE', *, *, #31094, .T. ) ;
#5841=ORIENTED_EDGE ( 'NONE', *, *, #10301, .F. ) ;
#5842=DIRECTION ( 'NONE',  ( 0.000000000000000000, 0.000000000000000000, 1.000000000000000000 ) ) ;
#5852=DIRECTION ( 'NONE',  ( 0.000000000000000000, 0.000000000000000000, -1.000000000000000000 ) ) ;
#5856=EDGE_CURVE ( 'NONE', #11163, #10000, #13912, .T. ) ;
#5857=ADVANCED_FACE ( 'NONE', ( #560 ), #8733, .T. ) ;
#5858=CIRCLE ( 'NONE', #18392, 4.000000000000003553 ) ;
#5860=FACE_OUTER_BOUND ( 'NONE', #34716, .T. ) ;
#5864=VERTEX_POINT ( 'NONE', #9094 ) ;
#5865=ORIENTED_EDGE ( 'NONE', *, *, #33499, .T. ) ;
#5870=CARTESIAN_POINT ( 'NONE',  ( -442.0000000000000000, 105.0000000000000000, -77.99999999999997158 ) ) ;
#5871=CARTESIAN_POINT ( 'NONE',  ( 15.99999999999998579, -55.00000000000000711, 154.9999999999999716 ) ) ;
#5873=EDGE_CURVE ( 'NONE', #7256, #8689, #32937, .T. ) ;
#5875=EDGE_CURVE ( 'NONE', #16444, #14255, #19957, .T. ) ;
#5879=ORIENTED_EDGE ( 'NONE', *, *, #11927, .F. ) ;
#5880=VERTEX_POINT ( 'NONE', #30638 ) ;
#5881=CIRCLE ( 'NONE', #13856, 3.999999999999976019 ) ;
#5882=DIRECTION ( 'NONE',  ( 0.000000000000000000, -1.000000000000000000, 6.123233995736766036E-17 ) ) ;
#5883=EDGE_CURVE ( 'NONE', #16221, #25357, #27780, .T. ) ;
#5888=DIRECTION ( 'NONE',  ( 1.000000000000000000, 0.000000000000000000, -1.848892746611746966E-32 ) ) ;
#5890=LINE ( 'NONE', #12141, #20303 ) ;
#5891=EDGE_CURVE ( 'NONE', #9401, #24518, #14093, .T. ) ;
#5892=EDGE_LOOP ( 'NONE', ( #10072, #8196, #17320, #30908 ) ) ;
#5900=LINE ( 'NONE', #29771, #32614 ) ;
#5901=ORIENTED_EDGE ( 'NONE', *, *, #1334, .T. ) ;
#5902=FACE_OUTER_BOUND ( 'NONE', #33652, .T. ) ;
#5906=ORIENTED_EDGE ( 'NONE', *, *, #32593, .T. ) ;
#5908=AXIS2_PLACEMENT_3D ( 'NONE', #5559, #10582, #21430 ) ;
#5917=AXIS2_PLACEMENT_3D ( 'NONE', #773, #33337, #5734 ) ;
#5922=EDGE_LOOP ( 'NONE', ( #34253, #30940, #9654, #19471 ) ) ;
#5923=EDGE_LOOP ( 'NONE', ( #25751, #25025, #5313, #18495, #10692, #5356, #6545, #9302 ) ) ;
#5926=CIRCLE ( 'NONE', #30951, 4.000000000000003553 ) ;
#5928=CYLINDRICAL_SURFACE ( 'NONE', #33033, 4.000000000000003553 ) ;
#5929=ORIENTED_EDGE ( 'NONE', *, *, #10301, .T. ) ;
#5930=EDGE_LOOP ( 'NONE', ( #3414, #28127, #14004, #28219 ) ) ;
#5936=CIRCLE ( 'NONE', #8234, 7.999999999999979572 ) ;
#5938=PLANE ( 'NONE',  #4101 ) ;
#5939=DIRECTION ( 'NONE',  ( -0.000000000000000000, -0.000000000000000000, -1.000000000000000000 ) ) ;
#5941=ORIENTED_EDGE ( 'NONE', *, *, #10429, .F. ) ;
#5942=CARTESIAN_POINT ( 'NONE',  ( 11.99999999999999645, 144.9999999999999716, 159.0000000000000000 ) ) ;
#5943=ORIENTED_EDGE ( 'NONE', *, *, #18146, .T. ) ;
#5946=EDGE_LOOP ( 'NONE', ( #18306, #20248, #778, #16943 ) ) ;
#5947=DIRECTION ( 'NONE',  ( 1.000000000000000000, 0.000000000000000000, 5.546364386991661285E-52 ) ) ;
#5950=VERTEX_POINT ( 'NONE', #28829 ) ;
#5957=EDGE_LOOP ( 'NONE', ( #19222, #25936, #16658, #23581 ) ) ;
#5958=ORIENTED_EDGE ( 'NONE', *, *, #17584, .F. ) ;
#5961=EDGE_CURVE ( 'NONE', #4608, #12639, #9905, .T. ) ;
#5963=EDGE_CURVE ( 'NONE', #9255, #33691, #12307, .T. ) ;
#5964=LINE ( 'NONE', #643, #15777 ) ;
#5966=ORIENTED_EDGE ( 'NONE', *, *, #31444, .T. ) ;
#5968=DIRECTION ( 'NONE',  ( 1.000000000000000000, 0.000000000000000000, 0.000000000000000000 ) ) ;
#5971=DIRECTION ( 'NONE',  ( 0.000000000000000000, -0.000000000000000000, 1.000000000000000000 ) ) ;
#5973=VECTOR ( 'NONE', #23319, 1000.000000000000000 ) ;
#5974=CARTESIAN_POINT ( 'NONE',  ( -355.0000000000000000, -114.9999999999999858, 113.9999999999999858 ) ) ;
#5978=AXIS2_PLACEMENT_3D ( 'NONE', #6644, #974, #17542 ) ;
#5979=AXIS2_PLACEMENT_3D ( 'NONE', #28586, #1534, #22898 ) ;
#5982=CARTESIAN_POINT ( 'NONE',  ( -349.0000000000000000, -125.0000000000000284, 166.9999999999999716 ) ) ;
#5987=ORIENTED_EDGE ( 'NONE', *, *, #231, .T. ) ;
#5988=DIRECTION ( 'NONE',  ( 0.000000000000000000, -1.000000000000000000, -2.465190328815662439E-32 ) ) ;
#5989=CARTESIAN_POINT ( 'NONE',  ( -19.99999999999998934, -137.0000000000000000, 162.9999999999999716 ) ) ;
#5991=VERTEX_POINT ( 'NONE', #4594 ) ;
#5993=CARTESIAN_POINT ( 'NONE',  ( -12.00000000000001066, 136.9999999999999716, -175.0000000000000284 ) ) ;
#5994=CARTESIAN_POINT ( 'NONE',  ( -418.0000000000000000, 105.0000000000000000, 135.9999999999999716 ) ) ;
#5998=CARTESIAN_POINT ( 'NONE',  ( 19.99999999999996092, -145.0000000000000000, -186.9999999999999716 ) ) ;
#5999=VERTEX_POINT ( 'NONE', #23488 ) ;
#6002=EDGE_CURVE ( 'NONE', #26019, #34152, #1950, .T. ) ;
#6013=DIRECTION ( 'NONE',  ( 0.000000000000000000, 1.000000000000000000, 5.053935297177146739E-49 ) ) ;
#6014=CARTESIAN_POINT ( 'NONE',  ( -15.99999999999998579, -112.9999999999999858, -155.0000000000000284 ) ) ;
#6017=EDGE_CURVE ( 'NONE', #31113, #24248, #30357, .T. ) ;
#6018=EDGE_CURVE ( 'NONE', #34124, #32595, #4263, .T. ) ;
#6019=CARTESIAN_POINT ( 'NONE',  ( -365.0000000000000000, -125.0000000000000284, 130.0000000000000000 ) ) ;
#6022=EDGE_CURVE ( 'NONE', #25655, #5400, #12830, .T. ) ;
#6023=DIRECTION ( 'NONE',  ( 0.000000000000000000, 0.000000000000000000, 1.000000000000000000 ) ) ;
#6026=AXIS2_PLACEMENT_3D ( 'NONE', #28667, #20143, #14805 ) ;
#6028=CYLINDRICAL_SURFACE ( 'NONE', #2409, 7.999999999999979572 ) ;
#6030=VECTOR ( 'NONE', #8217, 1000.000000000000000 ) ;
#6031=CARTESIAN_POINT ( 'NONE',  ( -442.0000000000000000, -125.0000000000000000, 187.0000000000000000 ) ) ;
#6037=CARTESIAN_POINT ( 'NONE',  ( 19.99999999999998934, 112.9999999999999574, -175.0000000000000284 ) ) ;
#6044=DIRECTION ( 'NONE',  ( 0.000000000000000000, 0.000000000000000000, -1.000000000000000000 ) ) ;
#6046=DIRECTION ( 'NONE',  ( 0.000000000000000000, 1.000000000000000000, 1.224646799147353207E-16 ) ) ;
#6049=DIRECTION ( 'NONE',  ( 0.000000000000000000, 1.000000000000000000, 1.131431318426415506E-52 ) ) ;
#6051=EDGE_CURVE ( 'NONE', #29779, #16703, #34345, .T. ) ;
#6060=CARTESIAN_POINT ( 'NONE',  ( -499.9999999999999432, -113.0000000000000000, -155.0000000000000000 ) ) ;
#6061=DIRECTION ( 'NONE',  ( -1.000000000000000000, 0.000000000000000000, 0.000000000000000000 ) ) ;
#6064=DIRECTION ( 'NONE',  ( -2.530127506375325574E-80, 1.000000000000000000, 6.842277657836020854E-49 ) ) ;
#6068=DIRECTION ( 'NONE',  ( 0.000000000000000000, 1.000000000000000000, 5.145227585319922065E-49 ) ) ;
#6071=LINE ( 'NONE', #33849, #22931 ) ;
#6074=VECTOR ( 'NONE', #3531, 1000.000000000000000 ) ;
#6082=VECTOR ( 'NONE', #29669, 1000.000000000000000 ) ;
#6084=ORIENTED_EDGE ( 'NONE', *, *, #34966, .F. ) ;
#6088=AXIS2_PLACEMENT_3D ( 'NONE', #883, #9238, #705 ) ;
#6091=ORIENTED_EDGE ( 'NONE', *, *, #14811, .T. ) ;
#6099=DIRECTION ( 'NONE',  ( 1.000000000000000000, 3.469446951953834515E-18, 0.000000000000000000 ) ) ;
#6100=EDGE_LOOP ( 'NONE', ( #23228, #31203, #1076, #30690, #12698, #18855, #27814, #9487 ) ) ;
#6101=ORIENTED_EDGE ( 'NONE', *, *, #34373, .T. ) ;
#6102=EDGE_CURVE ( 'NONE', #14780, #24095, #31325, .T. ) ;
#6103=CARTESIAN_POINT ( 'NONE',  ( -19.99999999999998934, 75.55999999999990280, 177.7400000000000091 ) ) ;
#6106=CARTESIAN_POINT ( 'NONE',  ( 11.99999999999999645, 134.9999999999998863, 187.0000000000000000 ) ) ;
#6107=LINE ( 'NONE', #966, #26174 ) ;
#6108=VERTEX_POINT ( 'NONE', #20653 ) ;
#6112=ORIENTED_EDGE ( 'NONE', *, *, #11608, .F. ) ;
#6113=LINE ( 'NONE', #17013, #26515 ) ;
#6125=AXIS2_PLACEMENT_3D ( 'NONE', #5614, #11512, #16512 ) ;
#6126=EDGE_CURVE ( 'NONE', #35, #34661, #21532, .T. ) ;
#6127=ORIENTED_EDGE ( 'NONE', *, *, #27207, .T. ) ;
#6128=LINE ( 'NONE', #11317, #21171 ) ;
#6129=LINE ( 'NONE', #28034, #19992 ) ;
#6142=ORIENTED_EDGE ( 'NONE', *, *, #6018, .T. ) ;
#6144=PLANE ( 'NONE',  #34423 ) ;
#6148=DIRECTION ( 'NONE',  ( 0.000000000000000000, 0.000000000000000000, -1.000000000000000000 ) ) ;
#6151=DIRECTION ( 'NONE',  ( 0.000000000000000000, -7.888609052210118054E-31, -1.000000000000000000 ) ) ;
#6152=VECTOR ( 'NONE', #16384, 1000.000000000000000 ) ;
#6153=ORIENTED_EDGE ( 'NONE', *, *, #19154, .T. ) ;
#6155=DIRECTION ( 'NONE',  ( -0.000000000000000000, -0.000000000000000000, 1.000000000000000000 ) ) ;
#6157=VECTOR ( 'NONE', #20359, 1000.000000000000000 ) ;
#6160=DIRECTION ( 'NONE',  ( 1.000000000000000000, 3.469446951953834515E-18, 0.000000000000000000 ) ) ;
#6164=ADVANCED_FACE ( 'NONE', ( #29712 ), #13692, .T. ) ;
#6169=PLANE ( 'NONE',  #22266 ) ;
#6170=DIRECTION ( 'NONE',  ( 1.000000000000000000, 3.040835319149746090E-31, 1.232595164407830946E-32 ) ) ;
#6172=ORIENTED_EDGE ( 'NONE', *, *, #18618, .T. ) ;
#6177=VECTOR ( 'NONE', #11170, 1000.000000000000000 ) ;
#6185=ORIENTED_EDGE ( 'NONE', *, *, #19899, .T. ) ;
#6186=LINE ( 'NONE', #17617, #8041 ) ;
#6187=DIRECTION ( 'NONE',  ( 0.000000000000000000, 0.000000000000000000, -1.000000000000000000 ) ) ;
#6188=VECTOR ( 'NONE', #27293, 1000.000000000000000 ) ;
#6193=ORIENTED_EDGE ( 'NONE', *, *, #5711, .F. ) ;
#6194=DIRECTION ( 'NONE',  ( -3.469446951953832974E-18, -1.000000000000000000, -7.888609052210116302E-31 ) ) ;
#6196=EDGE_LOOP ( 'NONE', ( #9973, #31628, #6229, #28424 ) ) ;
#6197=CIRCLE ( 'NONE', #16449, 2.000000000000001776 ) ;
#6207=CARTESIAN_POINT ( 'NONE',  ( -365.0000000000000000, -119.0000000000000000, 110.0000000000000000 ) ) ;
#6209=FACE_OUTER_BOUND ( 'NONE', #17421, .T. ) ;
#6211=( NAMED_UNIT ( * ) PLANE_ANGLE_UNIT ( ) SI_UNIT ( $, .RADIAN. ) );
#6214=EDGE_LOOP ( 'NONE', ( #8870, #26253, #3248, #28580 ) ) ;
#6219=ADVANCED_FACE ( 'NONE', ( #23840 ), #10315, .T. ) ;
#6222=LINE ( 'NONE', #911, #895 ) ;
#6224=VECTOR ( 'NONE', #31383, 1000.000000000000000 ) ;
#6229=ORIENTED_EDGE ( 'NONE', *, *, #3023, .F. ) ;
#6232=LINE ( 'NONE', #921, #2327 ) ;
#6235=DIRECTION ( 'NONE',  ( 0.000000000000000000, 0.000000000000000000, 1.000000000000000000 ) ) ;
#6241=DIRECTION ( 'NONE',  ( -1.000000000000000000, 0.000000000000000000, 1.232595164407831220E-32 ) ) ;
#6242=DIRECTION ( 'NONE',  ( 0.000000000000000000, 0.000000000000000000, -1.000000000000000000 ) ) ;
#6244=LINE ( 'NONE', #3583, #3739 ) ;
#6245=LINE ( 'NONE', #14297, #22421 ) ;
#6246=DIRECTION ( 'NONE',  ( 1.000000000000000000, 0.000000000000000000, 0.000000000000000000 ) ) ;
#6249=CARTESIAN_POINT ( 'NONE',  ( -418.0000000000000000, -124.9999999999999858, -69.99999999999998579 ) ) ;
#6253=ORIENTED_EDGE ( 'NONE', *, *, #8008, .T. ) ;
#6255=EDGE_CURVE ( 'NONE', #25547, #17261, #13354, .T. ) ;
#6258=VECTOR ( 'NONE', #8785, 1000.000000000000000 ) ;
#6261=ORIENTED_EDGE ( 'NONE', *, *, #1841, .F. ) ;
#6263=FACE_OUTER_BOUND ( 'NONE', #26371, .T. ) ;
#6264=EDGE_CURVE ( 'NONE', #4827, #27012, #16793, .T. ) ;
#6266=ORIENTED_EDGE ( 'NONE', *, *, #14682, .T. ) ;
#6267=DIRECTION ( 'NONE',  ( 1.000000000000000000, 0.000000000000000000, 0.000000000000000000 ) ) ;
#6269=ORIENTED_EDGE ( 'NONE', *, *, #17400, .T. ) ;
#6277=VERTEX_POINT ( 'NONE', #8353 ) ;
#6278=AXIS2_PLACEMENT_3D ( 'NONE', #19178, #16152, #5443 ) ;
#6283=VERTEX_POINT ( 'NONE', #16914 ) ;
#6287=DIRECTION ( 'NONE',  ( 2.891205793294675861E-16, 0.000000000000000000, -1.000000000000000000 ) ) ;
#6289=VECTOR ( 'NONE', #18396, 1000.000000000000000 ) ;
#6290=VECTOR ( 'NONE', #6246, 1000.000000000000000 ) ;
#6295=DIRECTION ( 'NONE',  ( 0.000000000000000000, 0.000000000000000000, 1.000000000000000000 ) ) ;
#6298=ADVANCED_FACE ( 'NONE', ( #8873 ), #30068, .T. ) ;
#6301=DIRECTION ( 'NONE',  ( 0.000000000000000000, 3.374343856708137958E-53, -1.000000000000000000 ) ) ;
#6303=EDGE_CURVE ( 'NONE', #1235, #639, #19749, .T. ) ;
#6304=ORIENTED_EDGE ( 'NONE', *, *, #10010, .T. ) ;
#6309=EDGE_LOOP ( 'NONE', ( #5149, #24298, #16187, #26347, #3356, #27566 ) ) ;
#6310=FACE_BOUND ( 'NONE', #6100, .T. ) ;
#6313=CARTESIAN_POINT ( 'NONE',  ( -449.9999999999999432, 104.9999999999999858, -187.0000000000000000 ) ) ;
#6316=VERTEX_POINT ( 'NONE', #14052 ) ;
#6318=VECTOR ( 'NONE', #12498, 1000.000000000000000 ) ;
#6322=CIRCLE ( 'NONE', #28518, 7.999999999999979572 ) ;
#6324=LINE ( 'NONE', #1697, #11322 ) ;
#6325=CYLINDRICAL_SURFACE ( 'NONE', #31365, 4.750000000000004441 ) ;
#6329=PLANE ( 'NONE',  #11343 ) ;
#6331=CARTESIAN_POINT ( 'NONE',  ( 11.99999999999999645, -115.0000000000000142, 162.9999999999999716 ) ) ;
#6332=ADVANCED_FACE ( 'NONE', ( #3706 ), #30764, .F. ) ;
#6333=CARTESIAN_POINT ( 'NONE',  ( -12.00000000000001066, 144.9999999999999716, -190.9999999999999432 ) ) ;
#6335=CARTESIAN_POINT ( 'NONE',  ( -20.00000000000007461, 144.9999999999999716, -162.9999999999999716 ) ) ;
#6336=VERTEX_POINT ( 'NONE', #6014 ) ;
#6337=EDGE_CURVE ( 'NONE', #18108, #26418, #11376, .T. ) ;
#6338=EDGE_CURVE ( 'NONE', #6590, #9496, #28683, .T. ) ;
#6339=CARTESIAN_POINT ( 'NONE',  ( -499.9999999999999432, 140.9999999999999716, -162.9999999999999716 ) ) ;
#6340=ORIENTED_EDGE ( 'NONE', *, *, #23149, .F. ) ;
#6344=VECTOR ( 'NONE', #25559, 1000.000000000000000 ) ;
#6346=AXIS2_PLACEMENT_3D ( 'NONE', #25396, #1028, #11895 ) ;
#6349=DIRECTION ( 'NONE',  ( 0.000000000000000000, 1.310824597558155437E-49, 1.000000000000000000 ) ) ;
#6351=VECTOR ( 'NONE', #11934, 1000.000000000000000 ) ;
#6356=ORIENTED_EDGE ( 'NONE', *, *, #25539, .F. ) ;
#6357=PLANE ( 'NONE',  #22949 ) ;
#6358=CARTESIAN_POINT ( 'NONE',  ( -414.0000000000000568, 104.9999999999999858, -162.9999999999999716 ) ) ;
#6360=DIRECTION ( 'NONE',  ( -0.000000000000000000, 0.000000000000000000, -1.000000000000000000 ) ) ;
#6366=EDGE_CURVE ( 'NONE', #5175, #13611, #5836, .T. ) ;
#6369=EDGE_CURVE ( 'NONE', #1848, #27507, #23290, .T. ) ;
#6370=DIRECTION ( 'NONE',  ( 0.000000000000000000, 1.000000000000000000, 1.224646799147353207E-16 ) ) ;
#6376=AXIS2_PLACEMENT_3D ( 'NONE', #29826, #27316, #24640 ) ;
#6379=DIRECTION ( 'NONE',  ( 0.000000000000000000, 0.000000000000000000, -1.000000000000000000 ) ) ;
#6381=EDGE_LOOP ( 'NONE', ( #3221, #22225, #34631, #10297 ) ) ;
#6383=CARTESIAN_POINT ( 'NONE',  ( -499.9999999999999432, 136.9999999999999432, 194.9999999999999716 ) ) ;
#6384=LINE ( 'NONE', #9763, #19506 ) ;
#6385=ORIENTED_EDGE ( 'NONE', *, *, #3405, .T. ) ;
#6388=FACE_OUTER_BOUND ( 'NONE', #28269, .T. ) ;
#6402=VERTEX_POINT ( 'NONE', #28279 ) ;
#6403=DIRECTION ( 'NONE',  ( 0.000000000000000000, 1.000000000000000000, 2.465190328815662439E-32 ) ) ;
#6404=EDGE_CURVE ( 'NONE', #28665, #20300, #33230, .T. ) ;
#6405=EDGE_CURVE ( 'NONE', #19566, #34661, #21870, .T. ) ;
#6406=CARTESIAN_POINT ( 'NONE',  ( -12.00000000000001066, -124.9999999999999432, -154.9999999999999716 ) ) ;
#6409=VERTEX_POINT ( 'NONE', #31633 ) ;
#6410=DIRECTION ( 'NONE',  ( -0.000000000000000000, 1.000000000000000000, -0.000000000000000000 ) ) ;
#6411=ADVANCED_FACE ( 'NONE', ( #25954 ), #23123, .T. ) ;
#6412=FACE_OUTER_BOUND ( 'NONE', #33615, .T. ) ;
#6424=PLANE ( 'NONE',  #19433 ) ;
#6426=DIRECTION ( 'NONE',  ( -1.000000000000000000, 0.000000000000000000, 0.000000000000000000 ) ) ;
#6427=CARTESIAN_POINT ( 'NONE',  ( 12.00000000000001066, -134.9999999999999716, 187.0000000000000000 ) ) ;
#6428=CARTESIAN_POINT ( 'NONE',  ( -410.0000000000000568, -105.0000000000001279, 132.0000000000000000 ) ) ;
#6435=VERTEX_POINT ( 'NONE', #18147 ) ;
#6439=AXIS2_PLACEMENT_3D ( 'NONE', #16797, #6426, #25475 ) ;
#6442=ORIENTED_EDGE ( 'NONE', *, *, #30901, .F. ) ;
#6444=CARTESIAN_POINT ( 'NONE',  ( -418.0000000000000000, 137.0000000000000000, -155.0000000000000000 ) ) ;
#6447=ORIENTED_EDGE ( 'NONE', *, *, #15359, .F. ) ;
#6448=CARTESIAN_POINT ( 'NONE',  ( 15.99999999999998579, 112.9999999999999574, -155.0000000000000000 ) ) ;
#6449=LINE ( 'NONE', #22495, #1193 ) ;
#6450=EDGE_LOOP ( 'NONE', ( #28105, #26436, #33959, #10670 ) ) ;
#6451=ORIENTED_EDGE ( 'NONE', *, *, #21013, .T. ) ;
#6455=EDGE_CURVE ( 'NONE', #32595, #4812, #1574, .T. ) ;
#6457=LINE ( 'NONE', #21403, #3354 ) ;
#6458=CARTESIAN_POINT ( 'NONE',  ( -20.00000000000004619, -137.0000000000000000, -187.0000000000000000 ) ) ;
#6460=VERTEX_POINT ( 'NONE', #4559 ) ;
#6462=CIRCLE ( 'NONE', #33171, 8.000000000000007105 ) ;
#6463=EDGE_CURVE ( 'NONE', #16235, #33086, #26413, .T. ) ;
#6464=EDGE_CURVE ( 'NONE', #17403, #7548, #9417, .T. ) ;
#6465=FACE_OUTER_BOUND ( 'NONE', #9531, .T. ) ;
#6468=DIRECTION ( 'NONE',  ( 1.000000000000000000, 3.040835319149746528E-31, 1.232595164407830946E-32 ) ) ;
#6475=AXIS2_PLACEMENT_3D ( 'NONE', #23983, #10994, #7787 ) ;
#6479=LINE ( 'NONE', #17378, #27416 ) ;
#6481=AXIS2_PLACEMENT_3D ( 'NONE', #13079, #15571, #26409 ) ;
#6482=ORIENTED_EDGE ( 'NONE', *, *, #23666, .T. ) ;
#6485=ORIENTED_EDGE ( 'NONE', *, *, #3056, .F. ) ;
#6486=AXIS2_PLACEMENT_3D ( 'NONE', #3644, #5603, #19694 ) ;
#6488=DIRECTION ( 'NONE',  ( -1.000000000000000000, 0.000000000000000000, 0.000000000000000000 ) ) ;
#6491=DIRECTION ( 'NONE',  ( 0.000000000000000000, 0.000000000000000000, 1.000000000000000000 ) ) ;
#6492=AXIS2_PLACEMENT_3D ( 'NONE', #25629, #17655, #12477 ) ;
#6495=VECTOR ( 'NONE', #30656, 1000.000000000000000 ) ;
#6497=CARTESIAN_POINT ( 'NONE',  ( -349.0000000000000000, -125.0000000000000284, 130.0000000000000000 ) ) ;
#6498=VERTEX_POINT ( 'NONE', #6892 ) ;
#6502=FACE_OUTER_BOUND ( 'NONE', #5892, .T. ) ;
#6503=DIRECTION ( 'NONE',  ( -1.000000000000000000, 0.000000000000000000, -1.300283923313630633E-47 ) ) ;
#6504=CIRCLE ( 'NONE', #32089, 7.999999999999952038 ) ;
#6507=CARTESIAN_POINT ( 'NONE',  ( -355.0000000000000000, 132.9999999999999716, 126.0000000000000000 ) ) ;
#6508=EDGE_CURVE ( 'NONE', #24429, #33545, #26295, .T. ) ;
#6511=ORIENTED_EDGE ( 'NONE', *, *, #24255, .F. ) ;
#6514=DIRECTION ( 'NONE',  ( 0.000000000000000000, 1.000000000000000000, 0.000000000000000000 ) ) ;
#6515=DIRECTION ( 'NONE',  ( 1.000000000000000000, -0.000000000000000000, -0.000000000000000000 ) ) ;
#6516=VERTEX_POINT ( 'NONE', #1738 ) ;
#6517=VECTOR ( 'NONE', #17914, 1000.000000000000000 ) ;
#6520=CARTESIAN_POINT ( 'NONE',  ( 11.99999999999999645, -141.0000000000000000, 174.9999999999999432 ) ) ;
#6521=VECTOR ( 'NONE', #28447, 1000.000000000000000 ) ;
#6525=AXIS2_PLACEMENT_3D ( 'NONE', #9807, #31518, #14651 ) ;
#6526=ORIENTED_EDGE ( 'NONE', *, *, #3732, .T. ) ;
#6528=CYLINDRICAL_SURFACE ( 'NONE', #1233, 3.999999999999976019 ) ;
#6529=FACE_OUTER_BOUND ( 'NONE', #21562, .T. ) ;
#6530=CARTESIAN_POINT ( 'NONE',  ( -410.0000000000000568, 104.9999999999999858, -187.0000000000000000 ) ) ;
#6531=EDGE_CURVE ( 'NONE', #1296, #10318, #17449, .T. ) ;
#6537=ORIENTED_EDGE ( 'NONE', *, *, #12360, .F. ) ;
#6541=VECTOR ( 'NONE', #27992, 1000.000000000000000 ) ;
#6542=LINE ( 'NONE', #23443, #27694 ) ;
#6544=ORIENTED_EDGE ( 'NONE', *, *, #9052, .T. ) ;
#6545=ORIENTED_EDGE ( 'NONE', *, *, #3165, .F. ) ;
#6549=VECTOR ( 'NONE', #3488, 1000.000000000000000 ) ;
#6556=VECTOR ( 'NONE', #6349, 1000.000000000000000 ) ;
#6557=CARTESIAN_POINT ( 'NONE',  ( 15.99999999999998579, 144.9999999999999716, 162.9999999999999716 ) ) ;
#6558=DIRECTION ( 'NONE',  ( 0.000000000000000000, 1.000000000000000000, 1.224646799147353207E-16 ) ) ;
#6559=VERTEX_POINT ( 'NONE', #34666 ) ;
#6560=AXIS2_PLACEMENT_3D ( 'NONE', #18245, #28739, #20903 ) ;
#6561=FACE_OUTER_BOUND ( 'NONE', #1719, .T. ) ;
#6567=CARTESIAN_POINT ( 'NONE',  ( -15.99999999999998579, -137.0000000000000000, -155.0000000000000284 ) ) ;
#6568=CARTESIAN_POINT ( 'NONE',  ( 11.99999999999999645, -115.0000000000000142, 162.9999999999999716 ) ) ;
#6569=VECTOR ( 'NONE', #12475, 1000.000000000000000 ) ;
#6571=CARTESIAN_POINT ( 'NONE',  ( -442.0000000000000000, 105.0000000000000142, 155.0000000000000000 ) ) ;
#6572=DIRECTION ( 'NONE',  ( 0.000000000000000000, 0.000000000000000000, 1.000000000000000000 ) ) ;
#6573=VECTOR ( 'NONE', #14149, 1000.000000000000000 ) ;
#6575=EDGE_CURVE ( 'NONE', #17921, #24256, #7414, .T. ) ;
#6577=ORIENTED_EDGE ( 'NONE', *, *, #1243, .F. ) ;
#6589=PLANE ( 'NONE',  #5025 ) ;
#6590=VERTEX_POINT ( 'NONE', #21656 ) ;
#6591=ORIENTED_EDGE ( 'NONE', *, *, #11112, .T. ) ;
#6594=DIRECTION ( 'NONE',  ( 1.000000000000000000, 0.000000000000000000, 0.000000000000000000 ) ) ;
#6598=LINE ( 'NONE', #30472, #8990 ) ;
#6599=ORIENTED_EDGE ( 'NONE', *, *, #1120, .T. ) ;
#6601=DIRECTION ( 'NONE',  ( -0.000000000000000000, 1.000000000000000000, -0.000000000000000000 ) ) ;
#6604=CARTESIAN_POINT ( 'NONE',  ( -365.0000000000000000, -119.0000000000000000, 126.0000000000000000 ) ) ;
#6605=CARTESIAN_POINT ( 'NONE',  ( 19.99999999999998934, -115.0000000000000000, 162.9999999999999716 ) ) ;
#6609=DIRECTION ( 'NONE',  ( 0.000000000000000000, -2.309213040847544338E-50, -1.000000000000000000 ) ) ;
#6610=CARTESIAN_POINT ( 'NONE',  ( 15.99999999999998579, -55.00000000000002132, 162.9999999999999716 ) ) ;
#6614=VECTOR ( 'NONE', #19095, 1000.000000000000000 ) ;
#6615=ADVANCED_FACE ( 'NONE', ( #29329 ), #31806, .T. ) ;
#6618=VECTOR ( 'NONE', #18623, 1000.000000000000000 ) ;
#6619=ORIENTED_EDGE ( 'NONE', *, *, #33489, .T. ) ;
#6621=ORIENTED_EDGE ( 'NONE', *, *, #10961, .F. ) ;
#6624=CARTESIAN_POINT ( 'NONE',  ( -19.99999999999998934, 144.9999999999999716, -162.9999999999999432 ) ) ;
#6628=DIRECTION ( 'NONE',  ( 1.000000000000000000, 0.000000000000000000, 0.000000000000000000 ) ) ;
#6629=FACE_BOUND ( 'NONE', #9584, .T. ) ;
#6634=VECTOR ( 'NONE', #22644, 1000.000000000000000 ) ;
#6636=CARTESIAN_POINT ( 'NONE',  ( -500.0000000000000000, -145.0000000000000000, 162.9999999999999716 ) ) ;
#6644=CARTESIAN_POINT ( 'NONE',  ( -355.0000000000000000, 116.9999999999999858, 126.0000000000000000 ) ) ;
#6648=DIRECTION ( 'NONE',  ( 0.000000000000000000, 1.000000000000000000, 5.145227585319922065E-49 ) ) ;
#6649=( NAMED_UNIT ( * ) PLANE_ANGLE_UNIT ( ) SI_UNIT ( $, .RADIAN. ) );
#6653=ORIENTED_EDGE ( 'NONE', *, *, #27300, .T. ) ;
#6654=DIRECTION ( 'NONE',  ( 0.000000000000000000, 1.000000000000000000, 1.131431318426415506E-52 ) ) ;
#6657=ADVANCED_FACE ( 'NONE', ( #2433 ), #26650, .T. ) ;
#6658=ORIENTED_EDGE ( 'NONE', *, *, #9863, .F. ) ;
#6664=CIRCLE ( 'NONE', #29969, 7.999999999999979572 ) ;
#6669=VERTEX_POINT ( 'NONE', #10104 ) ;
#6671=LINE ( 'NONE', #17394, #6517 ) ;
#6674=AXIS2_PLACEMENT_3D ( 'NONE', #26120, #1907, #20442 ) ;
#6676=DIRECTION ( 'NONE',  ( 0.000000000000000000, 0.000000000000000000, -1.000000000000000000 ) ) ;
#6678=ORIENTED_EDGE ( 'NONE', *, *, #34837, .F. ) ;
#6679=ORIENTED_EDGE ( 'NONE', *, *, #4467, .T. ) ;
#6680=DIRECTION ( 'NONE',  ( -1.000000000000000000, 0.000000000000000000, 0.000000000000000000 ) ) ;
#6682=DIRECTION ( 'NONE',  ( 0.000000000000000000, 0.000000000000000000, -1.000000000000000000 ) ) ;
#6683=DIRECTION ( 'NONE',  ( 3.469446951953832974E-18, 1.000000000000000000, 7.888609052210116302E-31 ) ) ;
#6685=DIRECTION ( 'NONE',  ( -0.000000000000000000, -0.000000000000000000, -1.000000000000000000 ) ) ;
#6687=CARTESIAN_POINT ( 'NONE',  ( -499.9999999999998863, -109.0000000000000142, -162.9999999999999716 ) ) ;
#6690=DIRECTION ( 'NONE',  ( -1.000000000000000000, 0.000000000000000000, -1.300283923313630633E-47 ) ) ;
#6691=DIRECTION ( 'NONE',  ( 0.000000000000000000, 0.000000000000000000, -1.000000000000000000 ) ) ;
#6697=CARTESIAN_POINT ( 'NONE',  ( -12.00000000000001066, -124.9999999999999432, -154.9999999999999716 ) ) ;
#6698=LINE ( 'NONE', #15962, #6855 ) ;
#6699=CIRCLE ( 'NONE', #27150, 7.999999999999979572 ) ;
#6704=ADVANCED_FACE ( 'NONE', ( #5269 ), #21134, .T. ) ;
#6705=ORIENTED_EDGE ( 'NONE', *, *, #14218, .T. ) ;
#6706=EDGE_CURVE ( 'NONE', #23628, #16142, #12801, .T. ) ;
#6711=FACE_OUTER_BOUND ( 'NONE', #11643, .T. ) ;
#6713=VECTOR ( 'NONE', #20126, 1000.000000000000000 ) ;
#6714=DIRECTION ( 'NONE',  ( -0.000000000000000000, -0.000000000000000000, -1.000000000000000000 ) ) ;
#6715=DIRECTION ( 'NONE',  ( -0.000000000000000000, 1.000000000000000000, -0.000000000000000000 ) ) ;
#6720=ORIENTED_EDGE ( 'NONE', *, *, #34835, .T. ) ;
#6721=DIRECTION ( 'NONE',  ( 0.000000000000000000, 3.374343856708137958E-53, -1.000000000000000000 ) ) ;
#6723=FACE_BOUND ( 'NONE', #34036, .T. ) ;
#6724=VECTOR ( 'NONE', #32768, 1000.000000000000000 ) ;
#6726=DIRECTION ( 'NONE',  ( 1.000000000000000000, 0.000000000000000000, -1.232595164407831220E-32 ) ) ;
#6727=CARTESIAN_POINT ( 'NONE',  ( -418.0000000000000000, 109.0000000000000142, -175.0000000000000000 ) ) ;
#6728=DIRECTION ( 'NONE',  ( 0.000000000000000000, 1.000000000000000000, 1.224646799147353207E-16 ) ) ;
#6730=EDGE_CURVE ( 'NONE', #28532, #26055, #832, .T. ) ;
#6734=EDGE_CURVE ( 'NONE', #14082, #11787, #19353, .T. ) ;
#6735=PLANE ( 'NONE',  #27115 ) ;
#6738=CARTESIAN_POINT ( 'NONE',  ( -418.0000000000000000, -105.0000000000000142, 132.0000000000000000 ) ) ;
#6741=CARTESIAN_POINT ( 'NONE',  ( -355.0000000000000000, -131.0000000000000000, 130.0000000000000000 ) ) ;
#6746=UNCERTAINTY_MEASURE_WITH_UNIT (LENGTH_MEASURE( 1.000000000000000082E-05 ), #22080, 'distance_accuracy_value', 'NONE');
#6747=DIRECTION ( 'NONE',  ( 1.000000000000000000, 3.469446951953834515E-18, 0.000000000000000000 ) ) ;
#6753=EDGE_CURVE ( 'NONE', #33261, #22350, #4831, .T. ) ;
#6755=ORIENTED_EDGE ( 'NONE', *, *, #21763, .F. ) ;
#6756=DIRECTION ( 'NONE',  ( 0.000000000000000000, 0.000000000000000000, 1.000000000000000000 ) ) ;
#6759=ORIENTED_EDGE ( 'NONE', *, *, #20942, .F. ) ;
#6762=VECTOR ( 'NONE', #8821, 1000.000000000000000 ) ;
#6767=FACE_OUTER_BOUND ( 'NONE', #5491, .T. ) ;
#6768=CARTESIAN_POINT ( 'NONE',  ( -15.99999999999998579, -124.9999999999999432, -186.9999999999999716 ) ) ;
#6769=DIRECTION ( 'NONE',  ( 0.000000000000000000, 2.465190328815661892E-32, 1.000000000000000000 ) ) ;
#6780=DIRECTION ( 'NONE',  ( 0.000000000000000000, 0.000000000000000000, -1.000000000000000000 ) ) ;
#6782=VECTOR ( 'NONE', #26036, 1000.000000000000000 ) ;
#6783=FACE_OUTER_BOUND ( 'NONE', #31838, .T. ) ;
#6784=EDGE_CURVE ( 'NONE', #9096, #8875, #1448, .T. ) ;
#6785=DIRECTION ( 'NONE',  ( 0.000000000000000000, 1.000000000000000000, 5.145227585319922065E-49 ) ) ;
#6787=CARTESIAN_POINT ( 'NONE',  ( 19.99999999999998224, -55.00000000000000711, -158.9999999999999716 ) ) ;
#6788=PLANE ( 'NONE',  #25742 ) ;
#6789=ORIENTED_EDGE ( 'NONE', *, *, #2836, .T. ) ;
#6794=ORIENTED_EDGE ( 'NONE', *, *, #25399, .T. ) ;
#6796=ORIENTED_EDGE ( 'NONE', *, *, #1677, .F. ) ;
#6798=DIRECTION ( 'NONE',  ( 1.000000000000000000, 3.469446951953834515E-18, 0.000000000000000000 ) ) ;
#6801=DIRECTION ( 'NONE',  ( 0.000000000000000000, 0.000000000000000000, -1.000000000000000000 ) ) ;
#6805=DIRECTION ( 'NONE',  ( 2.736911063134582149E-48, -7.888609052210118054E-31, -1.000000000000000000 ) ) ;
#6810=DIRECTION ( 'NONE',  ( -1.848892746611746419E-32, -6.842277657836020854E-49, 1.000000000000000000 ) ) ;
#6811=ORIENTED_EDGE ( 'NONE', *, *, #8034, .F. ) ;
#6812=EDGE_CURVE ( 'NONE', #11236, #2088, #16690, .T. ) ;
#6814=CARTESIAN_POINT ( 'NONE',  ( -365.0000000000000000, 134.9999999999999716, 126.0000000000000000 ) ) ;
#6817=CARTESIAN_POINT ( 'NONE',  ( -430.0000000000000000, -119.0000000000000000, 113.9999999999999858 ) ) ;
#6819=CARTESIAN_POINT ( 'NONE',  ( 19.99999999999998224, 144.9999999999999716, -186.9999999999999716 ) ) ;
#6820=LINE ( 'NONE', #3444, #18342 ) ;
#6824=CARTESIAN_POINT ( 'NONE',  ( -418.0000000000000000, -125.0000000000000000, -101.9999999999999858 ) ) ;
#6826=EDGE_LOOP ( 'NONE', ( #21832, #10796 ) ) ;
#6828=LINE ( 'NONE', #28558, #12096 ) ;
#6832=ORIENTED_EDGE ( 'NONE', *, *, #12805, .F. ) ;
#6833=VERTEX_POINT ( 'NONE', #23414 ) ;
#6835=ORIENTED_EDGE ( 'NONE', *, *, #11062, .F. ) ;
#6837=CIRCLE ( 'NONE', #23342, 3.999999999999948042 ) ;
#6839=FACE_OUTER_BOUND ( 'NONE', #15655, .T. ) ;
#6840=DIRECTION ( 'NONE',  ( 0.000000000000000000, 0.000000000000000000, -1.000000000000000000 ) ) ;
#6841=CARTESIAN_POINT ( 'NONE',  ( -449.9999999999999432, -105.0000000000000142, -101.9999999999999858 ) ) ;
#6842=ORIENTED_EDGE ( 'NONE', *, *, #1334, .F. ) ;
#6843=EDGE_LOOP ( 'NONE', ( #30038, #3681, #30506, #7916 ) ) ;
#6844=ADVANCED_FACE ( 'NONE', ( #12055 ), #23253, .T. ) ;
#6845=LINE ( 'NONE', #26076, #25888 ) ;
#6848=EDGE_CURVE ( 'NONE', #763, #9401, #7201, .T. ) ;
#6849=DIRECTION ( 'NONE',  ( 0.000000000000000000, 1.000000000000000000, 5.145227585319922065E-49 ) ) ;
#6852=ADVANCED_FACE ( 'NONE', ( #20409 ), #25378, .F. ) ;
#6855=VECTOR ( 'NONE', #24287, 1000.000000000000000 ) ;
#6856=EDGE_CURVE ( 'NONE', #17691, #2320, #33926, .T. ) ;
#6859=DIRECTION ( 'NONE',  ( 0.000000000000000000, 0.000000000000000000, -1.000000000000000000 ) ) ;
#6865=CARTESIAN_POINT ( 'NONE',  ( -19.99999999999998934, -141.0000000000000000, 162.9999999999999716 ) ) ;
#6868=VECTOR ( 'NONE', #28045, 1000.000000000000000 ) ;
#6872=VERTEX_POINT ( 'NONE', #17748 ) ;
#6873=AXIS2_PLACEMENT_3D ( 'NONE', #10149, #2300, #26339 ) ;
#6875=AXIS2_PLACEMENT_3D ( 'NONE', #22252, #8719, #14614 ) ;
#6876=VECTOR ( 'NONE', #3287, 1000.000000000000000 ) ;
#6877=DIRECTION ( 'NONE',  ( 1.000000000000000000, 0.000000000000000000, 0.000000000000000000 ) ) ;
#6880=CARTESIAN_POINT ( 'NONE',  ( -500.0000000000000000, -113.0000000000000000, 162.9999999999999716 ) ) ;
#6882=CARTESIAN_POINT ( 'NONE',  ( -442.0000000000000000, -137.0000000000000000, -175.0000000000000000 ) ) ;
#6885=EDGE_LOOP ( 'NONE', ( #5966, #29158, #14846, #24386 ) ) ;
#6889=EDGE_CURVE ( 'NONE', #13897, #14045, #15109, .T. ) ;
#6890=DIRECTION ( 'NONE',  ( -1.000000000000000000, 0.000000000000000000, 0.000000000000000000 ) ) ;
#6891=AXIS2_PLACEMENT_3D ( 'NONE', #17693, #7320, #4642 ) ;
#6892=CARTESIAN_POINT ( 'NONE',  ( -499.9999999999999432, 104.9999999999999858, -187.0000000000000000 ) ) ;
#6894=LINE ( 'NONE', #23125, #6074 ) ;
#6895=CARTESIAN_POINT ( 'NONE',  ( -414.0000000000000568, 105.0000000000000000, -77.99999999999997158 ) ) ;
#6901=ORIENTED_EDGE ( 'NONE', *, *, #31218, .F. ) ;
#6905=VECTOR ( 'NONE', #18847, 1000.000000000000000 ) ;
#6906=DIRECTION ( 'NONE',  ( 0.000000000000000000, 0.000000000000000000, 1.000000000000000000 ) ) ;
#6911=DIRECTION ( 'NONE',  ( 0.000000000000000000, 0.000000000000000000, -1.000000000000000000 ) ) ;
#6913=CARTESIAN_POINT ( 'NONE',  ( 11.99999999999999645, -145.0000000000000000, -190.9999999999999432 ) ) ;
#6916=VECTOR ( 'NONE', #13650, 1000.000000000000000 ) ;
#6921=AXIS2_PLACEMENT_3D ( 'NONE', #18163, #5292, #12814 ) ;
#6923=EDGE_CURVE ( 'NONE', #1214, #13897, #31597, .T. ) ;
#6928=EDGE_LOOP ( 'NONE', ( #17966, #30775, #4998, #10249, #22700, #868, #21703, #20860 ) ) ;
#6930=PLANE ( 'NONE',  #15081 ) ;
#6933=CARTESIAN_POINT ( 'NONE',  ( -361.0000000000000000, -125.0000000000000284, 185.0000000000000000 ) ) ;
#6935=VERTEX_POINT ( 'NONE', #1360 ) ;
#6937=PLANE ( 'NONE',  #25937 ) ;
#6940=VERTEX_POINT ( 'NONE', #12235 ) ;
#6942=EDGE_CURVE ( 'NONE', #13175, #25965, #26603, .T. ) ;
#6943=EDGE_CURVE ( 'NONE', #16123, #5041, #22467, .T. ) ;
#6947=CARTESIAN_POINT ( 'NONE',  ( -430.0000000000000000, -114.9999999999999858, 113.9999999999999858 ) ) ;
#6948=AXIS2_PLACEMENT_3D ( 'NONE', #16892, #2979, #330 ) ;
#6955=CARTESIAN_POINT ( 'NONE',  ( -430.0000000000000000, -119.0000000000000000, 109.9999999999999858 ) ) ;
#6957=( NAMED_UNIT ( * ) SI_UNIT ( $, .STERADIAN. ) SOLID_ANGLE_UNIT ( ) );
#6959=ORIENTED_EDGE ( 'NONE', *, *, #29422, .T. ) ;
#6962=EDGE_CURVE ( 'NONE', #4948, #20279, #15950, .T. ) ;
#6963=ORIENTED_EDGE ( 'NONE', *, *, #23432, .T. ) ;
#6964=EDGE_CURVE ( 'NONE', #7371, #27008, #23766, .T. ) ;
#6968=VERTEX_POINT ( 'NONE', #10065 ) ;
#6969=VERTEX_POINT ( 'NONE', #15589 ) ;
#6970=DIRECTION ( 'NONE',  ( -1.232595164407830946E-32, -7.496237820289040735E-63, 1.000000000000000000 ) ) ;
#6974=VERTEX_POINT ( 'NONE', #26956 ) ;
#6977=DIRECTION ( 'NONE',  ( 0.000000000000000000, -1.000000000000000000, 0.000000000000000000 ) ) ;
#6978=ORIENTED_EDGE ( 'NONE', *, *, #24789, .F. ) ;
#6979=CIRCLE ( 'NONE', #1306, 7.999999999999979572 ) ;
#6981=AXIS2_PLACEMENT_3D ( 'NONE', #12531, #24774, #13934 ) ;
#6982=DIRECTION ( 'NONE',  ( 0.000000000000000000, 0.000000000000000000, -1.000000000000000000 ) ) ;
#6985=DIRECTION ( 'NONE',  ( 0.000000000000000000, 1.131431318426415506E-52, 1.000000000000000000 ) ) ;
#6988=CARTESIAN_POINT ( 'NONE',  ( 19.99999999999998934, -137.0000000000000000, -155.0000000000000284 ) ) ;
#6990=FACE_OUTER_BOUND ( 'NONE', #14129, .T. ) ;
#6996=DIRECTION ( 'NONE',  ( -0.000000000000000000, 0.000000000000000000, 1.000000000000000000 ) ) ;
#6999=DIRECTION ( 'NONE',  ( -0.000000000000000000, 1.000000000000000000, -0.000000000000000000 ) ) ;
#7000=ORIENTED_EDGE ( 'NONE', *, *, #8513, .F. ) ;
#7007=CARTESIAN_POINT ( 'NONE',  ( -15.99999999999998579, 112.9999999999999574, -155.0000000000000000 ) ) ;
#7011=ORIENTED_EDGE ( 'NONE', *, *, #34592, .F. ) ;
#7015=FACE_OUTER_BOUND ( 'NONE', #32100, .T. ) ;
#7016=VECTOR ( 'NONE', #6061, 1000.000000000000000 ) ;
#7017=CARTESIAN_POINT ( 'NONE',  ( 12.00000000000001066, -134.9999999999999716, 155.0000000000000000 ) ) ;
#7018=CARTESIAN_POINT ( 'NONE',  ( -410.0000000000000568, 105.0000000000000000, 132.0000000000000000 ) ) ;
#7019=ORIENTED_EDGE ( 'NONE', *, *, #3159, .T. ) ;
#7020=ORIENTED_EDGE ( 'NONE', *, *, #8826, .T. ) ;
#7023=CYLINDRICAL_SURFACE ( 'NONE', #464, 2.000000000000001776 ) ;
#7024=CARTESIAN_POINT ( 'NONE',  ( -20.00000000000007461, -113.0000000000000000, -155.0000000000000000 ) ) ;
#7025=CARTESIAN_POINT ( 'NONE',  ( -418.0000000000000000, -124.9999999999999716, 135.9999999999999716 ) ) ;
#7026=ORIENTED_EDGE ( 'NONE', *, *, #28804, .F. ) ;
#7030=AXIS2_PLACEMENT_3D ( 'NONE', #33365, #28386, #31228 ) ;
#7040=DIRECTION ( 'NONE',  ( -1.232595164407830946E-32, 0.000000000000000000, -1.000000000000000000 ) ) ;
#7041=CYLINDRICAL_SURFACE ( 'NONE', #34147, 3.999999999999976019 ) ;
#7042=CIRCLE ( 'NONE', #20708, 7.999999999999979572 ) ;
#7047=EDGE_CURVE ( 'NONE', #32367, #10757, #15774, .T. ) ;
#7050=EDGE_CURVE ( 'NONE', #19630, #13520, #19076, .T. ) ;
#7059=CIRCLE ( 'NONE', #13337, 3.999999999999976019 ) ;
#7065=ORIENTED_EDGE ( 'NONE', *, *, #25835, .T. ) ;
#7066=DIRECTION ( 'NONE',  ( -0.000000000000000000, -1.000000000000000000, -0.000000000000000000 ) ) ;
#7068=AXIS2_PLACEMENT_3D ( 'NONE', #21433, #1856, #2034 ) ;
#7069=DIRECTION ( 'NONE',  ( 1.000000000000000000, 0.000000000000000000, 0.000000000000000000 ) ) ;
#7070=FACE_BOUND ( 'NONE', #30489, .T. ) ;
#7076=EDGE_LOOP ( 'NONE', ( #4118, #718, #12932, #31672 ) ) ;
#7080=DIRECTION ( 'NONE',  ( 0.000000000000000000, 0.000000000000000000, -1.000000000000000000 ) ) ;
#7081=VERTEX_POINT ( 'NONE', #34803 ) ;
#7082=DIRECTION ( 'NONE',  ( 0.000000000000000000, 0.000000000000000000, 1.000000000000000000 ) ) ;
#7083=VECTOR ( 'NONE', #19383, 1000.000000000000000 ) ;
#7084=DIRECTION ( 'NONE',  ( 0.000000000000000000, -1.000000000000000000, -2.465190328815662439E-32 ) ) ;
#7087=LINE ( 'NONE', #17807, #25118 ) ;
#7088=EDGE_CURVE ( 'NONE', #33693, #9482, #7550, .T. ) ;
#7090=VECTOR ( 'NONE', #12302, 1000.000000000000000 ) ;
#7091=VERTEX_POINT ( 'NONE', #21271 ) ;
#7094=VERTEX_POINT ( 'NONE', #2392 ) ;
#7095=VECTOR ( 'NONE', #2223, 1000.000000000000000 ) ;
#7098=FACE_OUTER_BOUND ( 'NONE', #33930, .T. ) ;
#7101=AXIS2_PLACEMENT_3D ( 'NONE', #12422, #31616, #12586 ) ;
#7102=ORIENTED_EDGE ( 'NONE', *, *, #4940, .T. ) ;
#7106=EDGE_CURVE ( 'NONE', #4812, #32414, #34986, .T. ) ;
#7109=ORIENTED_EDGE ( 'NONE', *, *, #21557, .T. ) ;
#7110=EDGE_LOOP ( 'NONE', ( #14791, #1818 ) ) ;
#7111=DIRECTION ( 'NONE',  ( 0.000000000000000000, 1.000000000000000000, 1.224646799147353207E-16 ) ) ;
#7112=ORIENTED_EDGE ( 'NONE', *, *, #5379, .T. ) ;
#7117=DIRECTION ( 'NONE',  ( -0.000000000000000000, 1.000000000000000000, -0.000000000000000000 ) ) ;
#7126=CARTESIAN_POINT ( 'NONE',  ( -410.0000000000000568, -105.0000000000000142, -174.9999999999999432 ) ) ;
#7132=EDGE_LOOP ( 'NONE', ( #17614, #9652, #23679, #3538 ) ) ;
#7133=VERTEX_POINT ( 'NONE', #32289 ) ;
#7138=EDGE_CURVE ( 'NONE', #7094, #25411, #4298, .T. ) ;
#7140=VERTEX_POINT ( 'NONE', #785 ) ;
#7142=LINE ( 'NONE', #26896, #23053 ) ;
#7143=ORIENTED_EDGE ( 'NONE', *, *, #26142, .F. ) ;
#7148=DIRECTION ( 'NONE',  ( 0.000000000000000000, 0.000000000000000000, 1.000000000000000000 ) ) ;
#7150=CARTESIAN_POINT ( 'NONE',  ( -12.00000000000001066, -145.0000000000000000, 187.0000000000000000 ) ) ;
#7151=CARTESIAN_POINT ( 'NONE',  ( -363.0000000000000000, -125.0000000000000284, 126.0000000000000000 ) ) ;
#7153=LINE ( 'NONE', #34224, #19417 ) ;
#7154=VERTEX_POINT ( 'NONE', #2743 ) ;
#7157=AXIS2_PLACEMENT_3D ( 'NONE', #14719, #25903, #6676 ) ;
#7159=DIRECTION ( 'NONE',  ( 0.000000000000000000, 0.000000000000000000, 1.000000000000000000 ) ) ;
#7163=CARTESIAN_POINT ( 'NONE',  ( -442.0000000000000000, -105.0000000000000142, 159.0000000000000000 ) ) ;
#7167=EDGE_CURVE ( 'NONE', #29943, #2443, #8841, .T. ) ;
#7168=CIRCLE ( 'NONE', #1521, 4.750000000000004441 ) ;
#7173=CARTESIAN_POINT ( 'NONE',  ( -499.9999999999999432, 112.9999999999999574, 162.9999999999999716 ) ) ;
#7176=ORIENTED_EDGE ( 'NONE', *, *, #22098, .T. ) ;
#7178=STYLED_ITEM('',(#35254),#1117);
#7182=EDGE_LOOP ( 'NONE', ( #33208, #33502, #15644, #7955 ) ) ;
#7185=ORIENTED_EDGE ( 'NONE', *, *, #26292, .F. ) ;
#7186=DIRECTION ( 'NONE',  ( 0.000000000000000000, 1.000000000000000000, 2.465190328815662439E-32 ) ) ;
#7191=FACE_OUTER_BOUND ( 'NONE', #18202, .T. ) ;
#7192=ORIENTED_EDGE ( 'NONE', *, *, #31346, .F. ) ;
#7201=LINE ( 'NONE', #4358, #12269 ) ;
#7204=VECTOR ( 'NONE', #15036, 1000.000000000000000 ) ;
#7208=DIRECTION ( 'NONE',  ( 0.000000000000000000, 0.000000000000000000, -1.000000000000000000 ) ) ;
#7210=EDGE_CURVE ( 'NONE', #15103, #28398, #19314, .T. ) ;
#7211=FACE_OUTER_BOUND ( 'NONE', #11152, .T. ) ;
#7212=ORIENTED_EDGE ( 'NONE', *, *, #18421, .F. ) ;
#7216=AXIS2_PLACEMENT_3D ( 'NONE', #8707, #20109, #33974 ) ;
#7218=AXIS2_PLACEMENT_3D ( 'NONE', #29382, #31850, #23683 ) ;
#7219=ORIENTED_EDGE ( 'NONE', *, *, #2504, .T. ) ;
#7220=CYLINDRICAL_SURFACE ( 'NONE', #13760, 7.999999999999979572 ) ;
#7222=LINE ( 'NONE', #31272, #316 ) ;
#7227=CARTESIAN_POINT ( 'NONE',  ( -500.0000000000000000, -145.0000000000000000, 162.9999999999999716 ) ) ;
#7228=ORIENTED_EDGE ( 'NONE', *, *, #14075, .F. ) ;
#7229=CARTESIAN_POINT ( 'NONE',  ( -499.9999999999999432, 112.9999999999999574, -162.9999999999999716 ) ) ;
#7233=LINE ( 'NONE', #4732, #25032 ) ;
#7236=VERTEX_POINT ( 'NONE', #10941 ) ;
#7245=CARTESIAN_POINT ( 'NONE',  ( 11.99999999999999645, 124.9999999999999716, 187.0000000000000000 ) ) ;
#7246=VERTEX_POINT ( 'NONE', #5577 ) ;
#7247=EDGE_CURVE ( 'NONE', #890, #11445, #8264, .T. ) ;
#7249=DIRECTION ( 'NONE',  ( 0.000000000000000000, -1.131431318426415506E-52, -1.000000000000000000 ) ) ;
#7250=VECTOR ( 'NONE', #961, 1000.000000000000000 ) ;
#7251=EDGE_CURVE ( 'NONE', #1893, #33296, #16473, .T. ) ;
#7252=DIRECTION ( 'NONE',  ( 0.000000000000000000, 7.888609052210118054E-31, 1.000000000000000000 ) ) ;
#7255=DIRECTION ( 'NONE',  ( 0.000000000000000000, 0.000000000000000000, 1.000000000000000000 ) ) ;
#7256=VERTEX_POINT ( 'NONE', #19144 ) ;
#7257=DIRECTION ( 'NONE',  ( 1.000000000000000000, 3.040835319149746090E-31, 1.232595164407830946E-32 ) ) ;
#7259=AXIS2_PLACEMENT_3D ( 'NONE', #32972, #13780, #32805 ) ;
#7263=ORIENTED_EDGE ( 'NONE', *, *, #8238, .F. ) ;
#7264=AXIS2_PLACEMENT_3D ( 'NONE', #26871, #10328, #24372 ) ;
#7270=FACE_OUTER_BOUND ( 'NONE', #17750, .T. ) ;
#7273=ORIENTED_EDGE ( 'NONE', *, *, #20238, .F. ) ;
#7277=AXIS2_PLACEMENT_3D ( 'NONE', #18909, #16247, #27079 ) ;
#7279=ORIENTED_EDGE ( 'NONE', *, *, #426, .F. ) ;
#7282=VERTEX_POINT ( 'NONE', #21974 ) ;
#7283=EDGE_CURVE ( 'NONE', #12207, #32312, #8441, .T. ) ;
#7284=CARTESIAN_POINT ( 'NONE',  ( -355.0000000000000000, 130.9999999999999716, 109.9999999999999858 ) ) ;
#7285=DIRECTION ( 'NONE',  ( 0.000000000000000000, 0.000000000000000000, -1.000000000000000000 ) ) ;
#7287=AXIS2_PLACEMENT_3D ( 'NONE', #3864, #24875, #14406 ) ;
#7288=LINE ( 'NONE', #13015, #17481 ) ;
#7293=LINE ( 'NONE', #7467, #28304 ) ;
#7294=FACE_OUTER_BOUND ( 'NONE', #20368, .T. ) ;
#7295=CARTESIAN_POINT ( 'NONE',  ( 11.99999999999999645, -145.0000000000000000, -186.9999999999999716 ) ) ;
#7302=DIRECTION ( 'NONE',  ( 0.000000000000000000, 3.374343856708137958E-53, -1.000000000000000000 ) ) ;
#7312=VERTEX_POINT ( 'NONE', #23369 ) ;
#7316=CARTESIAN_POINT ( 'NONE',  ( -418.0000000000000000, -141.0000000000000000, -155.0000000000000000 ) ) ;
#7320=DIRECTION ( 'NONE',  ( 0.000000000000000000, 1.310824597558155437E-49, 1.000000000000000000 ) ) ;
#7322=VERTEX_POINT ( 'NONE', #1317 ) ;
#7328=EDGE_LOOP ( 'NONE', ( #27246, #4750, #25702, #12958 ) ) ;
#7330=CARTESIAN_POINT ( 'NONE',  ( -499.9999999999999432, -141.0000000000000000, -162.9999999999999716 ) ) ;
#7331=CIRCLE ( 'NONE', #10199, 3.999999999999976019 ) ;
#7332=VERTEX_POINT ( 'NONE', #6814 ) ;
#7333=EDGE_CURVE ( 'NONE', #25265, #29943, #23209, .T. ) ;
#7338=CARTESIAN_POINT ( 'NONE',  ( -418.0000000000000000, 105.0000000000000000, -77.99999999999997158 ) ) ;
#7341=ADVANCED_FACE ( 'NONE', ( #25335 ), #20366, .T. ) ;
#7342=CARTESIAN_POINT ( 'NONE',  ( -445.9999999999999432, -112.9999999999999858, 155.0000000000000000 ) ) ;
#7348=ORIENTED_EDGE ( 'NONE', *, *, #28057, .F. ) ;
#7349=CARTESIAN_POINT ( 'NONE',  ( -500.0000000000000000, -141.0000000000000000, 187.0000000000000000 ) ) ;
#7351=EDGE_CURVE ( 'NONE', #8689, #22441, #26042, .T. ) ;
#7352=CIRCLE ( 'NONE', #34667, 3.999999999999976019 ) ;
#7354=LINE ( 'NONE', #20556, #317 ) ;
#7356=ORIENTED_EDGE ( 'NONE', *, *, #2612, .F. ) ;
#7359=CARTESIAN_POINT ( 'NONE',  ( 11.99999999999999645, 144.9999999999999147, 187.0000000000000000 ) ) ;
#7362=ORIENTED_EDGE ( 'NONE', *, *, #31569, .F. ) ;
#7365=DIRECTION ( 'NONE',  ( 0.000000000000000000, 0.000000000000000000, -1.000000000000000000 ) ) ;
#7369=DIRECTION ( 'NONE',  ( -0.000000000000000000, 6.123233995736766036E-17, 1.000000000000000000 ) ) ;
#7371=VERTEX_POINT ( 'NONE', #9141 ) ;
#7372=AXIS2_PLACEMENT_3D ( 'NONE', #28999, #26327, #31830 ) ;
#7375=LINE ( 'NONE', #4006, #22129 ) ;
#7376=EDGE_LOOP ( 'NONE', ( #1810, #22306, #18745, #25043, #23903, #8065, #28326, #17589, #14965, #10425, #18910 ) ) ;
#7377=LINE ( 'NONE', #2571, #6618 ) ;
#7378=DIRECTION ( 'NONE',  ( 0.000000000000000000, -1.310824597558155437E-49, -1.000000000000000000 ) ) ;
#7381=LINE ( 'NONE', #21281, #14942 ) ;
#7384=ADVANCED_FACE ( 'NONE', ( #15199 ), #1657, .T. ) ;
#7386=FACE_OUTER_BOUND ( 'NONE', #4502, .T. ) ;
#7388=DIRECTION ( 'NONE',  ( 1.000000000000000000, 3.040835319149746528E-31, 1.232595164407830946E-32 ) ) ;
#7389=CARTESIAN_POINT ( 'NONE',  ( -499.9999999999999432, 136.9999999999999432, -155.0000000000000000 ) ) ;
#7391=ADVANCED_FACE ( 'NONE', ( #14688 ), #1488, .F. ) ;
#7397=ORIENTED_EDGE ( 'NONE', *, *, #23510, .T. ) ;
#7400=CARTESIAN_POINT ( 'NONE',  ( -19.99999999999998934, -137.0000000000000000, 187.0000000000000000 ) ) ;
#7402=DIRECTION ( 'NONE',  ( -0.000000000000000000, -1.000000000000000000, -0.000000000000000000 ) ) ;
#7403=ADVANCED_FACE ( 'NONE', ( #17180 ), #17363, .T. ) ;
#7406=DIRECTION ( 'NONE',  ( -0.000000000000000000, 0.000000000000000000, -1.000000000000000000 ) ) ;
#7409=ORIENTED_EDGE ( 'NONE', *, *, #12105, .T. ) ;
#7410=ORIENTED_EDGE ( 'NONE', *, *, #22989, .T. ) ;
#7411=LINE ( 'NONE', #31462, #16946 ) ;
#7414=LINE ( 'NONE', #10810, #3675 ) ;
#7418=CARTESIAN_POINT ( 'NONE',  ( -365.0000000000000000, -131.0000000000000000, 113.9999999999999858 ) ) ;
#7424=CARTESIAN_POINT ( 'NONE',  ( -349.0000000000000000, -125.0000000000000284, 113.9999999999999858 ) ) ;
#7425=ORIENTED_EDGE ( 'NONE', *, *, #25479, .F. ) ;
#7427=ORIENTED_EDGE ( 'NONE', *, *, #13712, .F. ) ;
#7430=VECTOR ( 'NONE', #17700, 1000.000000000000000 ) ;
#7431=VERTEX_POINT ( 'NONE', #31554 ) ;
#7436=DIRECTION ( 'NONE',  ( 1.000000000000000000, 3.040835319149746090E-31, 1.232595164407830946E-32 ) ) ;
#7449=EDGE_LOOP ( 'NONE', ( #17810, #27063, #6835, #31042 ) ) ;
#7451=DIRECTION ( 'NONE',  ( 0.000000000000000000, 0.000000000000000000, 1.000000000000000000 ) ) ;
#7455=ORIENTED_EDGE ( 'NONE', *, *, #10276, .T. ) ;
#7462=CARTESIAN_POINT ( 'NONE',  ( 19.99999999999998224, 134.9999999999999432, -162.9999999999999432 ) ) ;
#7463=ORIENTED_EDGE ( 'NONE', *, *, #11954, .F. ) ;
#7467=CARTESIAN_POINT ( 'NONE',  ( -19.99999999999998934, 144.9999999999999716, 162.9999999999999716 ) ) ;
#7469=CIRCLE ( 'NONE', #6891, 7.999999999999986677 ) ;
#7474=CARTESIAN_POINT ( 'NONE',  ( 12.00000000000001066, -60.99999999999997158, -175.0000000000000000 ) ) ;
#7476=DIRECTION ( 'NONE',  ( 1.000000000000000000, 0.000000000000000000, 1.300283923313630633E-47 ) ) ;
#7478=VECTOR ( 'NONE', #7436, 1000.000000000000000 ) ;
#7479=ORIENTED_EDGE ( 'NONE', *, *, #20683, .F. ) ;
#7482=CIRCLE ( 'NONE', #9209, 3.999999999999976019 ) ;
#7486=EDGE_CURVE ( 'NONE', #14225, #26110, #34758, .T. ) ;
#7493=ADVANCED_FACE ( 'NONE', ( #32072 ), #34583, .T. ) ;
#7494=LINE ( 'NONE', #7316, #29295 ) ;
#7495=CARTESIAN_POINT ( 'NONE',  ( -500.0000000000000000, -104.9999999999999858, -162.9999999999999716 ) ) ;
#7511=( GEOMETRIC_REPRESENTATION_CONTEXT ( 3 ) GLOBAL_UNCERTAINTY_ASSIGNED_CONTEXT ( ( #22475 ) ) GLOBAL_UNIT_ASSIGNED_CONTEXT ( ( #21468, #29648, #19685 ) ) REPRESENTATION_CONTEXT ( 'NONE', 'WORKASPACE' ) );
#7512=CARTESIAN_POINT ( 'NONE',  ( 15.99999999999998579, -145.0000000000000000, 162.9999999999999716 ) ) ;
#7513=CARTESIAN_POINT ( 'NONE',  ( -12.00000000000001066, 124.9999999999999716, 155.0000000000000000 ) ) ;
#7514=PLANE ( 'NONE',  #25174 ) ;
#7517=DIRECTION ( 'NONE',  ( 1.000000000000000000, 0.000000000000000000, -1.848892746611746966E-32 ) ) ;
#7518=ORIENTED_EDGE ( 'NONE', *, *, #2444, .T. ) ;
#7520=CARTESIAN_POINT ( 'NONE',  ( 15.99999999999998579, -56.99999999999997868, -154.9999999999999716 ) ) ;
#7522=ORIENTED_EDGE ( 'NONE', *, *, #18044, .F. ) ;
#7525=EDGE_CURVE ( 'NONE', #17161, #27507, #4483, .T. ) ;
#7526=VECTOR ( 'NONE', #18674, 1000.000000000000000 ) ;
#7532=ORIENTED_EDGE ( 'NONE', *, *, #5166, .T. ) ;
#7535=EDGE_CURVE ( 'NONE', #28627, #11597, #25920, .T. ) ;
#7537=LINE ( 'NONE', #18251, #29053 ) ;
#7540=EDGE_CURVE ( 'NONE', #13074, #4867, #26564, .T. ) ;
#7541=ORIENTED_EDGE ( 'NONE', *, *, #18034, .F. ) ;
#7547=CARTESIAN_POINT ( 'NONE',  ( -345.0000000000000000, 134.9999999999999716, 113.9999999999999858 ) ) ;
#7548=VERTEX_POINT ( 'NONE', #15545 ) ;
#7550=LINE ( 'NONE', #18442, #10578 ) ;
#7551=AXIS2_PLACEMENT_3D ( 'NONE', #20192, #8449, #22330 ) ;
#7557=VERTEX_POINT ( 'NONE', #23726 ) ;
#7565=PLANE ( 'NONE',  #3453 ) ;
#7566=DIRECTION ( 'NONE',  ( 1.232595164407830946E-32, 3.421138828918010427E-49, -1.000000000000000000 ) ) ;
#7568=CYLINDRICAL_SURFACE ( 'NONE', #22295, 3.999999999999976019 ) ;
#7579=CIRCLE ( 'NONE', #1899, 2.000000000000001776 ) ;
#7582=ADVANCED_FACE ( 'NONE', ( #21408 ), #15914, .T. ) ;
#7584=EDGE_CURVE ( 'NONE', #5838, #27122, #29763, .T. ) ;
#7591=CARTESIAN_POINT ( 'NONE',  ( -418.0000000000000000, -105.0000000000000142, 139.9999999999999716 ) ) ;
#7593=DIRECTION ( 'NONE',  ( 0.000000000000000000, 0.000000000000000000, -1.000000000000000000 ) ) ;
#7602=AXIS2_PLACEMENT_3D ( 'NONE', #22004, #24653, #13817 ) ;
#7603=LINE ( 'NONE', #4937, #7526 ) ;
#7604=ORIENTED_EDGE ( 'NONE', *, *, #3211, .T. ) ;
#7606=EDGE_CURVE ( 'NONE', #4507, #32250, #10003, .T. ) ;
#7607=CARTESIAN_POINT ( 'NONE',  ( -20.00000000000007461, 112.9999999999999574, -159.0000000000000000 ) ) ;
#7608=EDGE_CURVE ( 'NONE', #19198, #30770, #5707, .T. ) ;
#7609=DIRECTION ( 'NONE',  ( -3.040835319149746090E-31, -1.000000000000000000, 0.000000000000000000 ) ) ;
#7613=AXIS2_PLACEMENT_3D ( 'NONE', #32180, #8141, #26840 ) ;
#7621=VERTEX_POINT ( 'NONE', #24768 ) ;
#7625=CARTESIAN_POINT ( 'NONE',  ( -499.9999999999999432, 136.9999999999999432, 162.9999999999999716 ) ) ;
#7634=CARTESIAN_POINT ( 'NONE',  ( -430.0000000000000000, -133.0000000000000000, 126.0000000000000000 ) ) ;
#7635=DIRECTION ( 'NONE',  ( -1.000000000000000000, 0.000000000000000000, 0.000000000000000000 ) ) ;
#7636=DIRECTION ( 'NONE',  ( 0.000000000000000000, 0.000000000000000000, -1.000000000000000000 ) ) ;
#7638=ORIENTED_EDGE ( 'NONE', *, *, #31227, .T. ) ;
#7640=VECTOR ( 'NONE', #13941, 1000.000000000000000 ) ;
#7644=CARTESIAN_POINT ( 'NONE',  ( -449.9999999999999432, 137.0000000000000000, -155.0000000000000000 ) ) ;
#7648=CYLINDRICAL_SURFACE ( 'NONE', #699, 4.000000000000003553 ) ;
#7655=EDGE_CURVE ( 'NONE', #17624, #27112, #21747, .T. ) ;
#7656=VECTOR ( 'NONE', #555, 1000.000000000000000 ) ;
#7664=EDGE_LOOP ( 'NONE', ( #11874, #17392, #23792, #32982 ) ) ;
#7666=VERTEX_POINT ( 'NONE', #30286 ) ;
#7674=AXIS2_PLACEMENT_3D ( 'NONE', #4916, #27166, #32159 ) ;
#7679=LINE ( 'NONE', #2176, #34469 ) ;
#7683=ADVANCED_FACE ( 'NONE', ( #8403 ), #14106, .T. ) ;
#7684=VECTOR ( 'NONE', #28054, 1000.000000000000000 ) ;
#7685=CARTESIAN_POINT ( 'NONE',  ( -345.0000000000000000, -125.0000000000000284, 181.0000000000000000 ) ) ;
#7691=VECTOR ( 'NONE', #16711, 1000.000000000000000 ) ;
#7693=DIRECTION ( 'NONE',  ( -3.040835319149746528E-31, -1.000000000000000000, 0.000000000000000000 ) ) ;
#7694=ADVANCED_FACE ( 'NONE', ( #16435 ), #19278, .T. ) ;
#7695=DIRECTION ( 'NONE',  ( 0.000000000000000000, -1.000000000000000000, -2.465190328815662439E-32 ) ) ;
#7700=AXIS2_PLACEMENT_3D ( 'NONE', #29619, #31585, #31920 ) ;
#7701=EDGE_CURVE ( 'NONE', #6283, #6435, #16259, .T. ) ;
#7707=CARTESIAN_POINT ( 'NONE',  ( -410.0000000000000568, 124.9999999999999432, -162.9999999999999716 ) ) ;
#7709=ORIENTED_EDGE ( 'NONE', *, *, #15476, .T. ) ;
#7710=DIRECTION ( 'NONE',  ( 1.000000000000000000, 0.000000000000000000, 0.000000000000000000 ) ) ;
#7715=VERTEX_POINT ( 'NONE', #13747 ) ;
#7717=DIRECTION ( 'NONE',  ( 0.000000000000000000, 2.465190328815661892E-32, 1.000000000000000000 ) ) ;
#7722=ORIENTED_EDGE ( 'NONE', *, *, #1578, .T. ) ;
#7723=CARTESIAN_POINT ( 'NONE',  ( -345.0000000000000000, 124.9999999999999432, 168.9999999999999716 ) ) ;
#7724=DIRECTION ( 'NONE',  ( 1.000000000000000000, -0.000000000000000000, -0.000000000000000000 ) ) ;
#7727=DIRECTION ( 'NONE',  ( -1.000000000000000000, 0.000000000000000000, 0.000000000000000000 ) ) ;
#7728=ORIENTED_EDGE ( 'NONE', *, *, #4662, .T. ) ;
#7732=EDGE_LOOP ( 'NONE', ( #22287, #16154, #10591, #2077 ) ) ;
#7738=CARTESIAN_POINT ( 'NONE',  ( -12.00000000000001066, 134.9999999999998863, 187.0000000000000000 ) ) ;
#7739=ORIENTED_EDGE ( 'NONE', *, *, #15312, .T. ) ;
#7741=EDGE_LOOP ( 'NONE', ( #21467, #32024, #2663, #11767, #29338, #9409 ) ) ;
#7743=EDGE_LOOP ( 'NONE', ( #30871, #1289, #24851, #34537 ) ) ;
#7745=CARTESIAN_POINT ( 'NONE',  ( -70.00000000000000000, 75.55999999999990280, -177.7400000000000091 ) ) ;
#7747=DIRECTION ( 'NONE',  ( -1.000000000000000000, 0.000000000000000000, 0.000000000000000000 ) ) ;
#7752=EDGE_CURVE ( 'NONE', #27733, #25432, #28758, .T. ) ;
#7753=ORIENTED_EDGE ( 'NONE', *, *, #28290, .T. ) ;
#7757=ORIENTED_EDGE ( 'NONE', *, *, #11062, .T. ) ;
#7763=CARTESIAN_POINT ( 'NONE',  ( -418.0000000000000000, -125.0000000000000000, 159.0000000000000000 ) ) ;
#7770=LINE ( 'NONE', #7949, #19201 ) ;
#7774=DIRECTION ( 'NONE',  ( -0.000000000000000000, -0.000000000000000000, 1.000000000000000000 ) ) ;
#7777=VECTOR ( 'NONE', #30607, 1000.000000000000000 ) ;
#7779=DIRECTION ( 'NONE',  ( -0.000000000000000000, 5.053935297177146739E-49, 1.000000000000000000 ) ) ;
#7781=ORIENTED_EDGE ( 'NONE', *, *, #20959, .F. ) ;
#7783=FACE_OUTER_BOUND ( 'NONE', #32835, .T. ) ;
#7785=CARTESIAN_POINT ( 'NONE',  ( -12.00000000000001243, 134.9999999999999432, -154.9999999999999716 ) ) ;
#7787=DIRECTION ( 'NONE',  ( 0.000000000000000000, 0.000000000000000000, -1.000000000000000000 ) ) ;
#7814=ADVANCED_FACE ( 'NONE', ( #19969 ), #18317, .T. ) ;
#7817=EDGE_CURVE ( 'NONE', #30541, #29056, #14809, .T. ) ;
#7820=DIRECTION ( 'NONE',  ( -1.000000000000000000, 0.000000000000000000, 0.000000000000000000 ) ) ;
#7821=EDGE_LOOP ( 'NONE', ( #162, #13824, #12393, #22072 ) ) ;
#7824=CARTESIAN_POINT ( 'NONE',  ( -430.0000000000000000, 118.9999999999999716, 113.9999999999999858 ) ) ;
#7829=EDGE_LOOP ( 'NONE', ( #26573, #28655, #1430, #1724 ) ) ;
#7832=CARTESIAN_POINT ( 'NONE',  ( -418.0000000000000000, -125.0000000000000000, -109.9999999999999574 ) ) ;
#7835=AXIS2_PLACEMENT_3D ( 'NONE', #34944, #16436, #5187 ) ;
#7837=ADVANCED_FACE ( 'NONE', ( #18152 ), #28978, .F. ) ;
#7838=ADVANCED_FACE ( 'NONE', ( #1914 ), #745, .T. ) ;
#7840=CARTESIAN_POINT ( 'NONE',  ( -349.0000000000000000, -125.0000000000000284, 168.9999999999999716 ) ) ;
#7843=VECTOR ( 'NONE', #15241, 1000.000000000000000 ) ;
#7844=VERTEX_POINT ( 'NONE', #27177 ) ;
#7852=ORIENTED_EDGE ( 'NONE', *, *, #33222, .F. ) ;
#7856=VECTOR ( 'NONE', #2645, 1000.000000000000000 ) ;
#7857=EDGE_CURVE ( 'NONE', #22621, #11445, #2265, .T. ) ;
#7859=ORIENTED_EDGE ( 'NONE', *, *, #25543, .F. ) ;
#7863=DIRECTION ( 'NONE',  ( 1.000000000000000000, 0.000000000000000000, 0.000000000000000000 ) ) ;
#7868=CARTESIAN_POINT ( 'NONE',  ( -365.0000000000000000, -119.0000000000000000, 130.0000000000000000 ) ) ;
#7872=CARTESIAN_POINT ( 'NONE',  ( -70.00000000000000000, 4.559999999999908127, 172.9900000000000091 ) ) ;
#7875=EDGE_CURVE ( 'NONE', #5682, #27718, #34858, .T. ) ;
#7877=PLANE ( 'NONE',  #8613 ) ;
#7885=DIRECTION ( 'NONE',  ( 0.000000000000000000, 0.000000000000000000, 1.000000000000000000 ) ) ;
#7888=VECTOR ( 'NONE', #26284, 1000.000000000000000 ) ;
#7889=ORIENTED_EDGE ( 'NONE', *, *, #33581, .F. ) ;
#7894=AXIS2_PLACEMENT_3D ( 'NONE', #29937, #25957, #9933 ) ;
#7905=CARTESIAN_POINT ( 'NONE',  ( -418.0000000000000000, -124.9999999999999858, -73.99999999999998579 ) ) ;
#7908=CARTESIAN_POINT ( 'NONE',  ( -20.00000000000007461, 112.9999999999999574, 159.0000000000000000 ) ) ;
#7910=DIRECTION ( 'NONE',  ( 0.000000000000000000, 0.000000000000000000, -1.000000000000000000 ) ) ;
#7912=ORIENTED_EDGE ( 'NONE', *, *, #9086, .T. ) ;
#7913=AXIS2_PLACEMENT_3D ( 'NONE', #26723, #33913, #25540 ) ;
#7915=DIRECTION ( 'NONE',  ( 0.000000000000000000, -3.374343856708137958E-53, 1.000000000000000000 ) ) ;
#7916=ORIENTED_EDGE ( 'NONE', *, *, #25648, .T. ) ;
#7917=CARTESIAN_POINT ( 'NONE',  ( -500.0000000000000000, -137.0000000000000000, 155.0000000000000000 ) ) ;
#7921=VECTOR ( 'NONE', #27483, 1000.000000000000000 ) ;
#7922=CARTESIAN_POINT ( 'NONE',  ( -442.0000000000000000, -137.0000000000000000, 154.9999999999999716 ) ) ;
#7925=ORIENTED_EDGE ( 'NONE', *, *, #33501, .T. ) ;
#7928=AXIS2_PLACEMENT_3D ( 'NONE', #32942, #5360, #27085 ) ;
#7934=ORIENTED_EDGE ( 'NONE', *, *, #11535, .F. ) ;
#7947=LINE ( 'NONE', #8120, #16812 ) ;
#7949=CARTESIAN_POINT ( 'NONE',  ( -499.9999999999999432, 104.9999999999999858, 162.9999999999999716 ) ) ;
#7950=LINE ( 'NONE', #5267, #12061 ) ;
#7951=DIRECTION ( 'NONE',  ( -1.000000000000000000, 0.000000000000000000, 0.000000000000000000 ) ) ;
#7955=ORIENTED_EDGE ( 'NONE', *, *, #5611, .T. ) ;
#7957=ADVANCED_FACE ( 'NONE', ( #13486, #10282 ), #21140, .T. ) ;
#7959=CARTESIAN_POINT ( 'NONE',  ( -20.00000000000004619, -137.0000000000000000, -190.9999999999999716 ) ) ;
#7960=ORIENTED_EDGE ( 'NONE', *, *, #11222, .T. ) ;
#7964=LINE ( 'NONE', #21670, #26368 ) ;
#7965=AXIS2_PLACEMENT_3D ( 'NONE', #25804, #12300, #30631 ) ;
#7966=ORIENTED_EDGE ( 'NONE', *, *, #2239, .F. ) ;
#7967=DIRECTION ( 'NONE',  ( -0.000000000000000000, -0.000000000000000000, 1.000000000000000000 ) ) ;
#7969=DIRECTION ( 'NONE',  ( 1.000000000000000000, 0.000000000000000000, 0.000000000000000000 ) ) ;
#7970=VERTEX_POINT ( 'NONE', #29335 ) ;
#7973=DIRECTION ( 'NONE',  ( 0.000000000000000000, 0.000000000000000000, -1.000000000000000000 ) ) ;
#7978=CARTESIAN_POINT ( 'NONE',  ( -20.00000000000004619, -145.0000000000000000, -162.9999999999999432 ) ) ;
#7983=EDGE_CURVE ( 'NONE', #21957, #7154, #4928, .T. ) ;
#7984=DIRECTION ( 'NONE',  ( 1.000000000000000000, 0.000000000000000000, 0.000000000000000000 ) ) ;
#7986=VECTOR ( 'NONE', #19563, 1000.000000000000000 ) ;
#7988=DIRECTION ( 'NONE',  ( 1.232595164407830946E-32, 3.421138828918010427E-49, -1.000000000000000000 ) ) ;
#7990=EDGE_LOOP ( 'NONE', ( #18821, #21984, #19873, #21528, #24648, #23471, #22361, #1913 ) ) ;
#7991=ADVANCED_FACE ( 'NONE', ( #33220, #22372 ), #22557, .T. ) ;
#7996=ADVANCED_FACE ( 'NONE', ( #25381 ), #30563, .F. ) ;
#8000=DIRECTION ( 'NONE',  ( -0.000000000000000000, 1.000000000000000000, -0.000000000000000000 ) ) ;
#8002=( GEOMETRIC_REPRESENTATION_CONTEXT ( 3 ) GLOBAL_UNCERTAINTY_ASSIGNED_CONTEXT ( ( #14296 ) ) GLOBAL_UNIT_ASSIGNED_CONTEXT ( ( #32654, #8279, #18802 ) ) REPRESENTATION_CONTEXT ( 'NONE', 'WORKASPACE' ) );
#8006=CARTESIAN_POINT ( 'NONE',  ( -15.99999999999998579, -32.99999999999997158, -154.9999999999999716 ) ) ;
#8007=CYLINDRICAL_SURFACE ( 'NONE', #29632, 3.999999999999976019 ) ;
#8008=EDGE_CURVE ( 'NONE', #2489, #32312, #30380, .T. ) ;
#8009=DIRECTION ( 'NONE',  ( 1.000000000000000000, 0.000000000000000000, 0.000000000000000000 ) ) ;
#8010=LINE ( 'NONE', #18720, #4307 ) ;
#8019=ORIENTED_EDGE ( 'NONE', *, *, #1570, .F. ) ;
#8020=VECTOR ( 'NONE', #16216, 1000.000000000000000 ) ;
#8024=ORIENTED_EDGE ( 'NONE', *, *, #4096, .T. ) ;
#8025=AXIS2_PLACEMENT_3D ( 'NONE', #16850, #27675, #11677 ) ;
#8028=CARTESIAN_POINT ( 'NONE',  ( -12.00000000000001066, 134.9999999999998863, 162.9999999999999716 ) ) ;
#8031=ORIENTED_EDGE ( 'NONE', *, *, #24497, .F. ) ;
#8034=EDGE_CURVE ( 'NONE', #29789, #20441, #1016, .T. ) ;
#8038=DIRECTION ( 'NONE',  ( -1.000000000000000000, 0.000000000000000000, 0.000000000000000000 ) ) ;
#8041=VECTOR ( 'NONE', #9415, 1000.000000000000000 ) ;
#8043=CARTESIAN_POINT ( 'NONE',  ( 11.99999999999999645, 136.9999999999999716, 155.0000000000000000 ) ) ;
#8045=CARTESIAN_POINT ( 'NONE',  ( -20.00000000000007461, 136.9999999999999432, 162.9999999999999716 ) ) ;
#8047=DIRECTION ( 'NONE',  ( 1.000000000000000000, 3.040835319149746528E-31, 1.232595164407830946E-32 ) ) ;
#8050=DIRECTION ( 'NONE',  ( 0.000000000000000000, 0.000000000000000000, -1.000000000000000000 ) ) ;
#8052=AXIS2_PLACEMENT_3D ( 'NONE', #4538, #29122, #12942 ) ;
#8053=DIRECTION ( 'NONE',  ( -0.000000000000000000, 1.000000000000000000, -0.000000000000000000 ) ) ;
#8054=AXIS2_PLACEMENT_3D ( 'NONE', #15112, #6726, #1575 ) ;
#8056=LINE ( 'NONE', #2542, #25843 ) ;
#8059=EDGE_CURVE ( 'NONE', #31695, #27282, #17053, .T. ) ;
#8060=EDGE_CURVE ( 'NONE', #4867, #10934, #945, .T. ) ;
#8063=( LENGTH_UNIT ( ) NAMED_UNIT ( * ) SI_UNIT ( .MILLI., .METRE. ) );
#8065=ORIENTED_EDGE ( 'NONE', *, *, #11305, .T. ) ;
#8068=VERTEX_POINT ( 'NONE', #30731 ) ;
#8071=ORIENTED_EDGE ( 'NONE', *, *, #21380, .T. ) ;
#8072=DIRECTION ( 'NONE',  ( 0.000000000000000000, 0.000000000000000000, 1.000000000000000000 ) ) ;
#8073=( GEOMETRIC_REPRESENTATION_CONTEXT ( 3 ) GLOBAL_UNCERTAINTY_ASSIGNED_CONTEXT ( ( #14954 ) ) GLOBAL_UNIT_ASSIGNED_CONTEXT ( ( #11939, #17989, #14616 ) ) REPRESENTATION_CONTEXT ( 'NONE', 'WORKASPACE' ) );
#8077=DIRECTION ( 'NONE',  ( 0.000000000000000000, 0.000000000000000000, 1.000000000000000000 ) ) ;
#8080=VECTOR ( 'NONE', #26833, 1000.000000000000000 ) ;
#8082=DIRECTION ( 'NONE',  ( 0.000000000000000000, 0.000000000000000000, 1.000000000000000000 ) ) ;
#8085=ORIENTED_EDGE ( 'NONE', *, *, #26759, .F. ) ;
#8086=DIRECTION ( 'NONE',  ( 1.000000000000000000, 0.000000000000000000, 0.000000000000000000 ) ) ;
#8087=CARTESIAN_POINT ( 'NONE',  ( -500.0000000000000000, -113.0000000000000000, 194.9999999999999716 ) ) ;
#8091=DIRECTION ( 'NONE',  ( 0.000000000000000000, 1.224646799147353207E-16, -1.000000000000000000 ) ) ;
#8097=CARTESIAN_POINT ( 'NONE',  ( -442.0000000000000000, -109.0000000000000142, 155.0000000000000000 ) ) ;
#8099=EDGE_CURVE ( 'NONE', #726, #27282, #23601, .T. ) ;
#8102=VECTOR ( 'NONE', #33620, 1000.000000000000000 ) ;
#8103=EDGE_LOOP ( 'NONE', ( #23984, #18516, #16069, #24046, #5580, #1763 ) ) ;
#8105=AXIS2_PLACEMENT_3D ( 'NONE', #8316, #24326, #19017 ) ;
#8109=ORIENTED_EDGE ( 'NONE', *, *, #2367, .F. ) ;
#8117=CARTESIAN_POINT ( 'NONE',  ( 11.99999999999999645, -145.0000000000000000, -154.9999999999999716 ) ) ;
#8118=ORIENTED_EDGE ( 'NONE', *, *, #27834, .T. ) ;
#8120=CARTESIAN_POINT ( 'NONE',  ( 11.99999999999999645, 140.9999999999999716, 155.0000000000000000 ) ) ;
#8121=DIRECTION ( 'NONE',  ( 1.000000000000000000, 0.000000000000000000, 0.000000000000000000 ) ) ;
#8122=DIRECTION ( 'NONE',  ( -1.000000000000000000, 0.000000000000000000, -5.546364386991661285E-52 ) ) ;
#8125=DIRECTION ( 'NONE',  ( -0.000000000000000000, 0.000000000000000000, -1.000000000000000000 ) ) ;
#8127=AXIS2_PLACEMENT_3D ( 'NONE', #4013, #28597, #12245 ) ;
#8128=MECHANICAL_DESIGN_GEOMETRIC_PRESENTATION_REPRESENTATION('',(#23398),#17812);
#8129=FACE_OUTER_BOUND ( 'NONE', #19152, .T. ) ;
#8130=CIRCLE ( 'NONE', #29733, 7.999999999999979572 ) ;
#8133=CARTESIAN_POINT ( 'NONE',  ( -12.00000000000001066, -109.0000000000000142, 155.0000000000000000 ) ) ;
#8134=CARTESIAN_POINT ( 'NONE',  ( -418.0000000000000000, -112.9999999999999858, -155.0000000000000000 ) ) ;
#8137=DIRECTION ( 'NONE',  ( 0.000000000000000000, 5.145227585319922065E-49, 1.000000000000000000 ) ) ;
#8140=EDGE_CURVE ( 'NONE', #6590, #12207, #8489, .T. ) ;
#8141=DIRECTION ( 'NONE',  ( 0.000000000000000000, -1.000000000000000000, -1.224646799147353207E-16 ) ) ;
#8143=ORIENTED_EDGE ( 'NONE', *, *, #3119, .F. ) ;
#8145=CARTESIAN_POINT ( 'NONE',  ( -410.0000000000000568, 105.0000000000000142, 162.9999999999999716 ) ) ;
#8153=AXIS2_PLACEMENT_3D ( 'NONE', #17467, #33452, #27756 ) ;
#8155=ORIENTED_EDGE ( 'NONE', *, *, #32256, .F. ) ;
#8156=LINE ( 'NONE', #11012, #33402 ) ;
#8157=CARTESIAN_POINT ( 'NONE',  ( -15.99999999999998579, 75.55999999999990280, -172.9900000000000091 ) ) ;
#8161=CARTESIAN_POINT ( 'NONE',  ( 11.99999999999995559, -145.0000000000000000, -162.9999999999999432 ) ) ;
#8165=ORIENTED_EDGE ( 'NONE', *, *, #5681, .F. ) ;
#8166=VERTEX_POINT ( 'NONE', #3837 ) ;
#8170=CARTESIAN_POINT ( 'NONE',  ( -499.9999999999999432, 136.9999999999999432, 162.9999999999999716 ) ) ;
#8174=CYLINDRICAL_SURFACE ( 'NONE', #16404, 3.999999999999989786 ) ;
#8178=FACE_OUTER_BOUND ( 'NONE', #31226, .T. ) ;
#8179=VERTEX_POINT ( 'NONE', #17751 ) ;
#8180=CYLINDRICAL_SURFACE ( 'NONE', #19774, 3.999999999999976019 ) ;
#8181=CARTESIAN_POINT ( 'NONE',  ( -20.00000000000004619, 112.9999999999999574, -154.9999999999999716 ) ) ;
#8190=ORIENTED_EDGE ( 'NONE', *, *, #25260, .T. ) ;
#8192=CARTESIAN_POINT ( 'NONE',  ( -20.00000000000004619, -105.0000000000000000, -187.0000000000000000 ) ) ;
#8195=VECTOR ( 'NONE', #17307, 1000.000000000000000 ) ;
#8196=ORIENTED_EDGE ( 'NONE', *, *, #887, .T. ) ;
#8199=VECTOR ( 'NONE', #12716, 1000.000000000000000 ) ;
#8203=DIRECTION ( 'NONE',  ( 0.000000000000000000, 2.309213040847544338E-50, 1.000000000000000000 ) ) ;
#8205=VECTOR ( 'NONE', #61, 1000.000000000000000 ) ;
#8211=CARTESIAN_POINT ( 'NONE',  ( 18.92820323027550344, -115.0000000000000000, -158.9999999999999716 ) ) ;
#8216=DIRECTION ( 'NONE',  ( -1.000000000000000000, 0.000000000000000000, 0.000000000000000000 ) ) ;
#8217=DIRECTION ( 'NONE',  ( -2.154935995002245207E-17, -0.000000000000000000, -1.000000000000000000 ) ) ;
#8218=VECTOR ( 'NONE', #25137, 1000.000000000000000 ) ;
#8221=DIRECTION ( 'NONE',  ( 0.000000000000000000, 0.000000000000000000, 1.000000000000000000 ) ) ;
#8222=CARTESIAN_POINT ( 'NONE',  ( 11.99999999999999645, -55.00000000000000711, 162.9999999999999716 ) ) ;
#8224=CARTESIAN_POINT ( 'NONE',  ( -12.00000000000001066, 144.9999999999999716, 159.0000000000000000 ) ) ;
#8230=EDGE_LOOP ( 'NONE', ( #17213, #14529, #14877, #18329 ) ) ;
#8233=DIRECTION ( 'NONE',  ( -0.000000000000000000, -0.000000000000000000, 1.000000000000000000 ) ) ;
#8234=AXIS2_PLACEMENT_3D ( 'NONE', #22398, #8340, #11729 ) ;
#8238=EDGE_CURVE ( 'NONE', #1340, #7081, #22547, .T. ) ;
#8241=VECTOR ( 'NONE', #12172, 1000.000000000000000 ) ;
#8243=CARTESIAN_POINT ( 'NONE',  ( -20.00000000000007461, 136.9999999999999432, -155.0000000000000000 ) ) ;
#8245=ORIENTED_EDGE ( 'NONE', *, *, #10275, .T. ) ;
#8246=CARTESIAN_POINT ( 'NONE',  ( -499.9999999999999432, 112.9999999999999574, -194.9999999999999716 ) ) ;
#8249=ADVANCED_FACE ( 'NONE', ( #24077 ), #26934, .T. ) ;
#8250=DIRECTION ( 'NONE',  ( 0.000000000000000000, 0.000000000000000000, 1.000000000000000000 ) ) ;
#8252=ORIENTED_EDGE ( 'NONE', *, *, #19984, .T. ) ;
#8253=ORIENTED_EDGE ( 'NONE', *, *, #2365, .F. ) ;
#8259=EDGE_CURVE ( 'NONE', #7715, #33356, #27076, .T. ) ;
#8263=EDGE_CURVE ( 'NONE', #4626, #24189, #20755, .T. ) ;
#8264=LINE ( 'NONE', #30148, #6573 ) ;
#8266=CARTESIAN_POINT ( 'NONE',  ( -410.0000000000000568, -125.0000000000000000, 187.0000000000000000 ) ) ;
#8269=ADVANCED_FACE ( 'NONE', ( #28242 ), #20243, .T. ) ;
#8274=AXIS2_PLACEMENT_3D ( 'NONE', #20650, #31493, #32680 ) ;
#8275=DIRECTION ( 'NONE',  ( 0.000000000000000000, 1.000000000000000000, 2.465190328815662439E-32 ) ) ;
#8276=ORIENTED_EDGE ( 'NONE', *, *, #21307, .F. ) ;
#8279=( NAMED_UNIT ( * ) PLANE_ANGLE_UNIT ( ) SI_UNIT ( $, .RADIAN. ) );
#8286=AXIS2_PLACEMENT_3D ( 'NONE', #8755, #19637, #31004 ) ;
#8287=ORIENTED_EDGE ( 'NONE', *, *, #7875, .F. ) ;
#8292=VERTEX_POINT ( 'NONE', #21450 ) ;
#8294=CARTESIAN_POINT ( 'NONE',  ( 19.99999999999998224, -55.00000000000000711, -154.9999999999999716 ) ) ;
#8295=LINE ( 'NONE', #21479, #9622 ) ;
#8297=DIRECTION ( 'NONE',  ( 0.000000000000000000, 0.000000000000000000, -1.000000000000000000 ) ) ;
#8300=EDGE_LOOP ( 'NONE', ( #8620, #32439, #30606, #15427 ) ) ;
#8301=CARTESIAN_POINT ( 'NONE',  ( -20.00000000000001776, -113.0000000000000000, 190.9999999999999716 ) ) ;
#8305=AXIS2_PLACEMENT_3D ( 'NONE', #11614, #13655, #2790 ) ;
#8307=ADVANCED_FACE ( 'NONE', ( #26783 ), #13616, .T. ) ;
#8308=EDGE_CURVE ( 'NONE', #3718, #32967, #7377, .T. ) ;
#8316=CARTESIAN_POINT ( 'NONE',  ( 11.99999999999999645, -115.0000000000000000, 162.9999999999999716 ) ) ;
#8318=ADVANCED_FACE ( 'NONE', ( #29811 ), #15778, .T. ) ;
#8319=DIRECTION ( 'NONE',  ( 1.000000000000000000, -0.000000000000000000, -0.000000000000000000 ) ) ;
#8325=DIRECTION ( 'NONE',  ( 1.000000000000000000, -0.000000000000000000, -0.000000000000000000 ) ) ;
#8327=LINE ( 'NONE', #16712, #5214 ) ;
#8329=ORIENTED_EDGE ( 'NONE', *, *, #8387, .T. ) ;
#8333=CARTESIAN_POINT ( 'NONE',  ( -499.9999999999999432, 104.9999999999999858, 187.0000000000000000 ) ) ;
#8334=EDGE_CURVE ( 'NONE', #4421, #3207, #5412, .T. ) ;
#8340=DIRECTION ( 'NONE',  ( -1.000000000000000000, 0.000000000000000000, 1.232595164407831220E-32 ) ) ;
#8345=ORIENTED_EDGE ( 'NONE', *, *, #15652, .T. ) ;
#8346=DIRECTION ( 'NONE',  ( -3.469446951953832974E-18, -1.000000000000000000, -7.888609052210116302E-31 ) ) ;
#8348=EDGE_CURVE ( 'NONE', #15373, #32238, #27133, .T. ) ;
#8353=CARTESIAN_POINT ( 'NONE',  ( -347.0000000000000000, 134.9999999999999716, 126.0000000000000000 ) ) ;
#8355=VERTEX_POINT ( 'NONE', #21622 ) ;
#8360=ORIENTED_EDGE ( 'NONE', *, *, #16093, .F. ) ;
#8362=DIRECTION ( 'NONE',  ( 0.000000000000000000, 0.000000000000000000, -1.000000000000000000 ) ) ;
#8363=DIRECTION ( 'NONE',  ( 0.000000000000000000, 0.000000000000000000, 1.000000000000000000 ) ) ;
#8364=ORIENTED_EDGE ( 'NONE', *, *, #12404, .F. ) ;
#8366=DIRECTION ( 'NONE',  ( 1.000000000000000000, 0.000000000000000000, 0.000000000000000000 ) ) ;
#8370=CARTESIAN_POINT ( 'NONE',  ( -12.00000000000001066, 140.9999999999999716, -175.0000000000000284 ) ) ;
#8372=AXIS2_PLACEMENT_3D ( 'NONE', #30429, #22069, #3539 ) ;
#8373=AXIS2_PLACEMENT_3D ( 'NONE', #31380, #1826, #12187 ) ;
#8379=ORIENTED_EDGE ( 'NONE', *, *, #19499, .F. ) ;
#8380=CIRCLE ( 'NONE', #25984, 4.000000000000003553 ) ;
#8385=CARTESIAN_POINT ( 'NONE',  ( -499.9999999999999432, -145.0000000000000000, -187.0000000000000000 ) ) ;
#8387=EDGE_CURVE ( 'NONE', #16257, #5027, #24731, .T. ) ;
#8388=FACE_OUTER_BOUND ( 'NONE', #8759, .T. ) ;
#8394=CARTESIAN_POINT ( 'NONE',  ( -12.00000000000001066, 144.9999999999999716, -186.9999999999999716 ) ) ;
#8395=ADVANCED_FACE ( 'NONE', ( #13097 ), #29465, .T. ) ;
#8401=DIRECTION ( 'NONE',  ( 0.000000000000000000, 0.000000000000000000, -1.000000000000000000 ) ) ;
#8402=CIRCLE ( 'NONE', #9559, 4.000000000000003553 ) ;
#8403=FACE_OUTER_BOUND ( 'NONE', #33163, .T. ) ;
#8404=LINE ( 'NONE', #26737, #3290 ) ;
#8406=( NAMED_UNIT ( * ) SI_UNIT ( $, .STERADIAN. ) SOLID_ANGLE_UNIT ( ) );
#8408=DIRECTION ( 'NONE',  ( -1.000000000000000000, 0.000000000000000000, 1.848892746611746966E-32 ) ) ;
#8409=MECHANICAL_DESIGN_GEOMETRIC_PRESENTATION_REPRESENTATION('',(#20364),#2710);
#8417=VECTOR ( 'NONE', #18213, 1000.000000000000000 ) ;
#8422=ORIENTED_EDGE ( 'NONE', *, *, #22091, .T. ) ;
#8426=CARTESIAN_POINT ( 'NONE',  ( 11.99999999999999645, 134.9999999999998863, 155.0000000000000000 ) ) ;
#8431=VERTEX_POINT ( 'NONE', #26433 ) ;
#8435=EDGE_CURVE ( 'NONE', #27344, #32731, #17463, .T. ) ;
#8441=LINE ( 'NONE', #5745, #29882 ) ;
#8448=CYLINDRICAL_SURFACE ( 'NONE', #13781, 3.999999999999976019 ) ;
#8449=DIRECTION ( 'NONE',  ( 1.000000000000000000, 3.040835319149746528E-31, 1.232595164407830946E-32 ) ) ;
#8451=ORIENTED_EDGE ( 'NONE', *, *, #32887, .F. ) ;
#8464=EDGE_CURVE ( 'NONE', #25101, #12748, #33357, .T. ) ;
#8468=CARTESIAN_POINT ( 'NONE',  ( -430.0000000000000000, -117.0000000000000000, 113.9999999999999858 ) ) ;
#8469=VERTEX_POINT ( 'NONE', #266 ) ;
#8470=ORIENTED_EDGE ( 'NONE', *, *, #9383, .T. ) ;
#8471=CARTESIAN_POINT ( 'NONE',  ( -365.0000000000000000, 116.9999999999999858, 113.9999999999999858 ) ) ;
#8476=EDGE_LOOP ( 'NONE', ( #19930, #4070, #8031, #10541 ) ) ;
#8478=DIRECTION ( 'NONE',  ( 5.546364386991661285E-52, 0.000000000000000000, 1.000000000000000000 ) ) ;
#8481=DIRECTION ( 'NONE',  ( 1.000000000000000000, 0.000000000000000000, 0.000000000000000000 ) ) ;
#8483=CARTESIAN_POINT ( 'NONE',  ( 12.00000000000001066, -64.99999999999997158, -175.0000000000000000 ) ) ;
#8486=CARTESIAN_POINT ( 'NONE',  ( -414.0000000000000568, -124.9999999999999858, -77.99999999999997158 ) ) ;
#8489=LINE ( 'NONE', #30198, #29296 ) ;
#8491=LINE ( 'NONE', #19539, #11528 ) ;
#8496=ORIENTED_EDGE ( 'NONE', *, *, #25634, .T. ) ;
#8497=DIRECTION ( 'NONE',  ( 0.000000000000000000, 0.000000000000000000, 1.000000000000000000 ) ) ;
#8499=AXIS2_PLACEMENT_3D ( 'NONE', #15321, #28657, #29001 ) ;
#8500=ORIENTED_EDGE ( 'NONE', *, *, #3903, .F. ) ;
#8503=FACE_OUTER_BOUND ( 'NONE', #16906, .T. ) ;
#8506=AXIS2_PLACEMENT_3D ( 'NONE', #31965, #4725, #2076 ) ;
#8511=ORIENTED_EDGE ( 'NONE', *, *, #4936, .T. ) ;
#8513=EDGE_CURVE ( 'NONE', #5041, #14854, #6113, .T. ) ;
#8517=ORIENTED_EDGE ( 'NONE', *, *, #34012, .T. ) ;
#8519=ORIENTED_EDGE ( 'NONE', *, *, #8906, .T. ) ;
#8525=LINE ( 'NONE', #5493, #17483 ) ;
#8529=ORIENTED_EDGE ( 'NONE', *, *, #20887, .F. ) ;
#8530=AXIS2_PLACEMENT_3D ( 'NONE', #27245, #19086, #32757 ) ;
#8531=VERTEX_POINT ( 'NONE', #27837 ) ;
#8532=CARTESIAN_POINT ( 'NONE',  ( -499.9999999999999432, 136.9999999999999432, -159.0000000000000000 ) ) ;
#8534=ORIENTED_EDGE ( 'NONE', *, *, #25230, .F. ) ;
#8535=PLANE ( 'NONE',  #20351 ) ;
#8536=DIRECTION ( 'NONE',  ( 0.000000000000000000, -1.000000000000000000, 6.123233995736766036E-17 ) ) ;
#8537=CARTESIAN_POINT ( 'NONE',  ( -418.0000000000000000, -104.9999999999999716, -187.0000000000000000 ) ) ;
#8541=LINE ( 'NONE', #21719, #25251 ) ;
#8542=CARTESIAN_POINT ( 'NONE',  ( 15.99999999999998579, 124.9999999999999716, 187.0000000000000000 ) ) ;
#8548=ORIENTED_EDGE ( 'NONE', *, *, #5609, .T. ) ;
#8554=DIRECTION ( 'NONE',  ( 0.000000000000000000, 0.000000000000000000, 1.000000000000000000 ) ) ;
#8558=CIRCLE ( 'NONE', #1202, 4.000000000000003553 ) ;
#8567=DIRECTION ( 'NONE',  ( 1.000000000000000000, 3.040835319149746528E-31, 1.232595164407830946E-32 ) ) ;
#8571=AXIS2_PLACEMENT_3D ( 'NONE', #13789, #27294, #10770 ) ;
#8575=LINE ( 'NONE', #8224, #17814 ) ;
#8578=DIRECTION ( 'NONE',  ( 0.000000000000000000, 1.000000000000000000, -6.842277657836020854E-49 ) ) ;
#8585=VECTOR ( 'NONE', #15501, 1000.000000000000000 ) ;
#8586=VECTOR ( 'NONE', #27760, 1000.000000000000000 ) ;
#8592=VERTEX_POINT ( 'NONE', #9327 ) ;
#8596=VECTOR ( 'NONE', #4222, 1000.000000000000000 ) ;
#8599=FACE_OUTER_BOUND ( 'NONE', #16959, .T. ) ;
#8600=CARTESIAN_POINT ( 'NONE',  ( -347.0000000000000000, 134.9999999999999716, 114.0000000000000000 ) ) ;
#8601=VERTEX_POINT ( 'NONE', #6819 ) ;
#8604=DIRECTION ( 'NONE',  ( 0.000000000000000000, -1.000000000000000000, -2.465190328815662439E-32 ) ) ;
#8606=CARTESIAN_POINT ( 'NONE',  ( -442.0000000000000000, 124.9999999999999432, -155.0000000000000000 ) ) ;
#8613=AXIS2_PLACEMENT_3D ( 'NONE', #13409, #24242, #12147 ) ;
#8615=DIRECTION ( 'NONE',  ( 0.000000000000000000, -2.465190328815661892E-32, -1.000000000000000000 ) ) ;
#8616=FACE_OUTER_BOUND ( 'NONE', #12595, .T. ) ;
#8618=ORIENTED_EDGE ( 'NONE', *, *, #5078, .F. ) ;
#8619=DIRECTION ( 'NONE',  ( 0.000000000000000000, -5.145227585319922065E-49, -1.000000000000000000 ) ) ;
#8620=ORIENTED_EDGE ( 'NONE', *, *, #18281, .T. ) ;
#8622=FACE_OUTER_BOUND ( 'NONE', #9036, .T. ) ;
#8626=CARTESIAN_POINT ( 'NONE',  ( -430.0000000000000000, -131.0000000000000000, 126.0000000000000000 ) ) ;
#8630=ADVANCED_FACE ( 'NONE', ( #28888 ), #25338, .T. ) ;
#8633=VECTOR ( 'NONE', #34057, 1000.000000000000000 ) ;
#8634=EDGE_CURVE ( 'NONE', #2214, #16123, #20023, .T. ) ;
#8636=ORIENTED_EDGE ( 'NONE', *, *, #22989, .F. ) ;
#8638=CARTESIAN_POINT ( 'NONE',  ( 12.00000000000001066, -32.99999999999997158, -154.9999999999999716 ) ) ;
#8640=EDGE_LOOP ( 'NONE', ( #7757, #28443, #30687, #19475 ) ) ;
#8641=AXIS2_PLACEMENT_3D ( 'NONE', #2491, #18885, #8366 ) ;
#8644=CARTESIAN_POINT ( 'NONE',  ( -414.0000000000000568, -137.0000000000000000, -155.0000000000000000 ) ) ;
#8646=CARTESIAN_POINT ( 'NONE',  ( -430.0000000000000000, 130.9999999999999716, 111.9999999999999858 ) ) ;
#8647=ORIENTED_EDGE ( 'NONE', *, *, #29737, .T. ) ;
#8648=EDGE_LOOP ( 'NONE', ( #623, #33785, #8529, #13242 ) ) ;
#8652=DIRECTION ( 'NONE',  ( 0.000000000000000000, -1.000000000000000000, 3.374343856708137958E-53 ) ) ;
#8654=LINE ( 'NONE', #27174, #2120 ) ;
#8657=CLOSED_SHELL ( 'NONE', ( #21004, #24410, #19616, #27914, #22164, #33945, #5857, #9540, #21077, #25711, #3534, #28709, #5521, #14832, #3612, #13063, #34674, #3473, #25599, #8758, #28836, #208, #26922, #18145, #7341, #17096, #3003 ) ) ;
#8660=AXIS2_PLACEMENT_3D ( 'NONE', #29260, #15749, #22572 ) ;
#8662=DIRECTION ( 'NONE',  ( 0.000000000000000000, -1.000000000000000000, -5.053935297177146739E-49 ) ) ;
#8663=VERTEX_POINT ( 'NONE', #1320 ) ;
#8664=AXIS2_PLACEMENT_3D ( 'NONE', #15250, #13274, #17934 ) ;
#8666=AXIS2_PLACEMENT_3D ( 'NONE', #22559, #837, #11705 ) ;
#8667=LINE ( 'NONE', #2795, #28614 ) ;
#8668=ORIENTED_EDGE ( 'NONE', *, *, #32045, .F. ) ;
#8669=CARTESIAN_POINT ( 'NONE',  ( -349.0000000000000000, 124.9999999999999432, 168.9999999999999716 ) ) ;
#8671=ORIENTED_EDGE ( 'NONE', *, *, #24789, .T. ) ;
#8674=DIRECTION ( 'NONE',  ( -0.000000000000000000, 0.000000000000000000, -1.000000000000000000 ) ) ;
#8676=ADVANCED_FACE ( 'NONE', ( #17370 ), #4488, .T. ) ;
#8677=VERTEX_POINT ( 'NONE', #20534 ) ;
#8682=ORIENTED_EDGE ( 'NONE', *, *, #15815, .F. ) ;
#8683=FACE_OUTER_BOUND ( 'NONE', #30492, .T. ) ;
#8686=LINE ( 'NONE', #19218, #7986 ) ;
#8689=VERTEX_POINT ( 'NONE', #25695 ) ;
#8695=DIRECTION ( 'NONE',  ( 1.848892746611746419E-32, 6.842277657836020854E-49, -1.000000000000000000 ) ) ;
#8696=ORIENTED_EDGE ( 'NONE', *, *, #29160, .T. ) ;
#8701=CARTESIAN_POINT ( 'NONE',  ( -499.9999999999999432, 144.9999999999999716, 187.0000000000000000 ) ) ;
#8702=LINE ( 'NONE', #3361, #25067 ) ;
#8705=ORIENTED_EDGE ( 'NONE', *, *, #8747, .T. ) ;
#8706=EDGE_CURVE ( 'NONE', #3104, #23064, #28196, .T. ) ;
#8707=CARTESIAN_POINT ( 'NONE',  ( -361.0000000000000000, -125.0000000000000284, 181.0000000000000000 ) ) ;
#8708=AXIS2_PLACEMENT_3D ( 'NONE', #2185, #18587, #10374 ) ;
#8714=DIRECTION ( 'NONE',  ( -1.000000000000000000, 0.000000000000000000, 0.000000000000000000 ) ) ;
#8716=DIRECTION ( 'NONE',  ( 1.000000000000000000, 3.469446951953834515E-18, 0.000000000000000000 ) ) ;
#8718=AXIS2_PLACEMENT_3D ( 'NONE', #6568, #33275, #3890 ) ;
#8719=DIRECTION ( 'NONE',  ( 1.000000000000000000, 0.000000000000000000, 0.000000000000000000 ) ) ;
#8721=ORIENTED_EDGE ( 'NONE', *, *, #33222, .T. ) ;
#8726=DIRECTION ( 'NONE',  ( 0.000000000000000000, -1.000000000000000000, 6.123233995736766036E-17 ) ) ;
#8730=LINE ( 'NONE', #16595, #304 ) ;
#8733=CYLINDRICAL_SURFACE ( 'NONE', #25244, 7.999999999999979572 ) ;
#8736=ORIENTED_EDGE ( 'NONE', *, *, #18783, .T. ) ;
#8738=VECTOR ( 'NONE', #1842, 1000.000000000000000 ) ;
#8741=DIRECTION ( 'NONE',  ( 0.000000000000000000, 0.000000000000000000, -1.000000000000000000 ) ) ;
#8746=CARTESIAN_POINT ( 'NONE',  ( -355.0000000000000000, 130.9999999999999716, 128.0000000000000000 ) ) ;
#8747=EDGE_CURVE ( 'NONE', #8677, #33838, #10200, .T. ) ;
#8755=CARTESIAN_POINT ( 'NONE',  ( -363.0000000000000000, -125.0000000000000284, 114.0000000000000000 ) ) ;
#8756=VECTOR ( 'NONE', #1685, 1000.000000000000000 ) ;
#8758=ADVANCED_FACE ( 'NONE', ( #10024 ), #34412, .T. ) ;
#8759=EDGE_LOOP ( 'NONE', ( #3295, #19128, #4474, #9139 ) ) ;
#8760=CARTESIAN_POINT ( 'NONE',  ( -499.9999999999999432, 104.9999999999999858, -187.0000000000000000 ) ) ;
#8761=AXIS2_PLACEMENT_3D ( 'NONE', #12920, #23762, #34619 ) ;
#8762=ORIENTED_EDGE ( 'NONE', *, *, #13140, .T. ) ;
#8763=AXIS2_PLACEMENT_3D ( 'NONE', #2882, #30484, #27981 ) ;
#8769=DIRECTION ( 'NONE',  ( 0.000000000000000000, 0.000000000000000000, -1.000000000000000000 ) ) ;
#8775=VERTEX_POINT ( 'NONE', #16084 ) ;
#8776=FACE_OUTER_BOUND ( 'NONE', #5477, .T. ) ;
#8777=CARTESIAN_POINT ( 'NONE',  ( -445.9999999999999432, -137.0000000000000000, -155.0000000000000000 ) ) ;
#8778=ORIENTED_EDGE ( 'NONE', *, *, #7752, .T. ) ;
#8780=DIRECTION ( 'NONE',  ( -3.040835319149746090E-31, -1.000000000000000000, 0.000000000000000000 ) ) ;
#8785=DIRECTION ( 'NONE',  ( -1.000000000000000000, 0.000000000000000000, -1.300283923313630633E-47 ) ) ;
#8786=CARTESIAN_POINT ( 'NONE',  ( 0.000000000000000000, 144.9999999999999716, 194.9999999999999716 ) ) ;
#8790=DIRECTION ( 'NONE',  ( 0.000000000000000000, 1.310824597558155437E-49, 1.000000000000000000 ) ) ;
#8794=DIRECTION ( 'NONE',  ( -1.000000000000000000, 0.000000000000000000, -1.300283923313630633E-47 ) ) ;
#8796=AXIS2_PLACEMENT_3D ( 'NONE', #17075, #690, #16545 ) ;
#8798=CARTESIAN_POINT ( 'NONE',  ( -349.0000000000000000, 124.9999999999999432, 164.9999999999999716 ) ) ;
#8800=CARTESIAN_POINT ( 'NONE',  ( -418.0000000000000000, 105.0000000000000000, 132.0000000000000000 ) ) ;
#8806=AXIS2_PLACEMENT_3D ( 'NONE', #32239, #2167, #15528 ) ;
#8811=EDGE_LOOP ( 'NONE', ( #6112, #22318, #32658, #29442 ) ) ;
#8817=VERTEX_POINT ( 'NONE', #4657 ) ;
#8821=DIRECTION ( 'NONE',  ( 0.000000000000000000, -1.000000000000000000, -2.309213040847544338E-50 ) ) ;
#8823=DIRECTION ( 'NONE',  ( -0.000000000000000000, 1.000000000000000000, -0.000000000000000000 ) ) ;
#8824=ORIENTED_EDGE ( 'NONE', *, *, #27472, .T. ) ;
#8825=ORIENTED_EDGE ( 'NONE', *, *, #11727, .F. ) ;
#8826=EDGE_CURVE ( 'NONE', #6559, #29137, #5511, .T. ) ;
#8827=DIRECTION ( 'NONE',  ( 0.000000000000000000, 1.000000000000000000, -3.374343856708137958E-53 ) ) ;
#8833=VECTOR ( 'NONE', #22893, 1000.000000000000000 ) ;
#8837=DIRECTION ( 'NONE',  ( -3.469446951953832974E-18, -1.000000000000000000, 7.888609052210118054E-31 ) ) ;
#8840=EDGE_CURVE ( 'NONE', #18883, #1235, #6664, .T. ) ;
#8841=CIRCLE ( 'NONE', #32715, 4.000000000000003553 ) ;
#8842=CARTESIAN_POINT ( 'NONE',  ( -430.0000000000000000, 118.9999999999999716, 126.0000000000000000 ) ) ;
#8843=CYLINDRICAL_SURFACE ( 'NONE', #5195, 4.750000000000004441 ) ;
#8844=DIRECTION ( 'NONE',  ( -0.000000000000000000, 1.000000000000000000, -0.000000000000000000 ) ) ;
#8847=VERTEX_POINT ( 'NONE', #7512 ) ;
#8848=LINE ( 'NONE', #6520, #16800 ) ;
#8849=CARTESIAN_POINT ( 'NONE',  ( -449.9999999999999432, -112.9999999999999858, -174.9999999999999716 ) ) ;
#8855=DIRECTION ( 'NONE',  ( 1.000000000000000000, 0.000000000000000000, 0.000000000000000000 ) ) ;
#8860=DIRECTION ( 'NONE',  ( 0.000000000000000000, 1.310824597558155437E-49, 1.000000000000000000 ) ) ;
#8868=ORIENTED_EDGE ( 'NONE', *, *, #29287, .T. ) ;
#8870=ORIENTED_EDGE ( 'NONE', *, *, #24062, .F. ) ;
#8873=FACE_OUTER_BOUND ( 'NONE', #20609, .T. ) ;
#8875=VERTEX_POINT ( 'NONE', #22288 ) ;
#8876=ORIENTED_EDGE ( 'NONE', *, *, #4086, .T. ) ;
#8877=DIRECTION ( 'NONE',  ( 0.000000000000000000, 1.000000000000000000, 1.224646799147353207E-16 ) ) ;
#8878=ORIENTED_EDGE ( 'NONE', *, *, #23991, .T. ) ;
#8880=DIRECTION ( 'NONE',  ( 1.000000000000000000, 0.000000000000000000, -1.848892746611746966E-32 ) ) ;
#8885=CIRCLE ( 'NONE', #15741, 7.999999999999979572 ) ;
#8886=( LENGTH_UNIT ( ) NAMED_UNIT ( * ) SI_UNIT ( .MILLI., .METRE. ) );
#8887=EDGE_CURVE ( 'NONE', #13361, #35039, #22115, .T. ) ;
#8894=DIRECTION ( 'NONE',  ( 3.040835319149746090E-31, 1.000000000000000000, 0.000000000000000000 ) ) ;
#8895=FACE_OUTER_BOUND ( 'NONE', #3760, .T. ) ;
#8897=CARTESIAN_POINT ( 'NONE',  ( -12.00000000000001066, 108.9999999999999858, -175.0000000000000284 ) ) ;
#8898=EDGE_LOOP ( 'NONE', ( #2420, #7889, #13126, #2853 ) ) ;
#8899=EDGE_CURVE ( 'NONE', #6409, #32490, #574, .T. ) ;
#8903=EDGE_LOOP ( 'NONE', ( #33153, #31403, #27468, #31746 ) ) ;
#8904=AXIS2_PLACEMENT_3D ( 'NONE', #26162, #31676, #23680 ) ;
#8906=EDGE_CURVE ( 'NONE', #12986, #5991, #20330, .T. ) ;
#8908=EDGE_CURVE ( 'NONE', #34042, #23786, #3816, .T. ) ;
#8909=CYLINDRICAL_SURFACE ( 'NONE', #13665, 7.999999999999952038 ) ;
#8911=ORIENTED_EDGE ( 'NONE', *, *, #18421, .T. ) ;
#8912=LINE ( 'NONE', #28136, #7090 ) ;
#8919=CARTESIAN_POINT ( 'NONE',  ( -410.0000000000000568, -112.9999999999999858, 154.9999999999999716 ) ) ;
#8921=DIRECTION ( 'NONE',  ( 0.000000000000000000, 1.000000000000000000, 0.000000000000000000 ) ) ;
#8924=ORIENTED_EDGE ( 'NONE', *, *, #576, .F. ) ;
#8925=CARTESIAN_POINT ( 'NONE',  ( -499.9999999999999432, 136.9999999999999432, -162.9999999999999716 ) ) ;
#8930=ORIENTED_EDGE ( 'NONE', *, *, #23202, .F. ) ;
#8932=AXIS2_PLACEMENT_3D ( 'NONE', #23133, #18625, #12931 ) ;
#8934=EDGE_CURVE ( 'NONE', #25561, #25012, #14109, .T. ) ;
#8936=CARTESIAN_POINT ( 'NONE',  ( 11.99999999999999645, -115.0000000000000000, -162.9999999999999432 ) ) ;
#8940=UNCERTAINTY_MEASURE_WITH_UNIT (LENGTH_MEASURE( 1.000000000000000082E-05 ), #8886, 'distance_accuracy_value', 'NONE');
#8943=CARTESIAN_POINT ( 'NONE',  ( -418.0000000000000000, -137.0000000000000000, -155.0000000000000000 ) ) ;
#8950=AXIS2_PLACEMENT_3D ( 'NONE', #1694, #20568, #31247 ) ;
#8951=VERTEX_POINT ( 'NONE', #24413 ) ;
#8956=DIRECTION ( 'NONE',  ( 0.000000000000000000, -2.309213040847544338E-50, -1.000000000000000000 ) ) ;
#8958=AXIS2_PLACEMENT_3D ( 'NONE', #5535, #5706, #8401 ) ;
#8959=VECTOR ( 'NONE', #19764, 1000.000000000000000 ) ;
#8961=ORIENTED_EDGE ( 'NONE', *, *, #20528, .T. ) ;
#8962=CARTESIAN_POINT ( 'NONE',  ( -445.9999999999999432, 113.0000000000000000, 154.9999999999999716 ) ) ;
#8964=ORIENTED_EDGE ( 'NONE', *, *, #12070, .T. ) ;
#8967=CARTESIAN_POINT ( 'NONE',  ( 19.99999999999998224, 134.9999999999998863, 187.0000000000000000 ) ) ;
#8969=FACE_OUTER_BOUND ( 'NONE', #21598, .T. ) ;
#8971=DIRECTION ( 'NONE',  ( 0.000000000000000000, 0.000000000000000000, 1.000000000000000000 ) ) ;
#8973=ORIENTED_EDGE ( 'NONE', *, *, #1463, .F. ) ;
#8977=VERTEX_POINT ( 'NONE', #30117 ) ;
#8983=AXIS2_PLACEMENT_3D ( 'NONE', #19834, #6628, #20179 ) ;
#8989=DIRECTION ( 'NONE',  ( 0.000000000000000000, 0.000000000000000000, 1.000000000000000000 ) ) ;
#8990=VECTOR ( 'NONE', #14810, 1000.000000000000000 ) ;
#8991=CIRCLE ( 'NONE', #16986, 3.999999999999976019 ) ;
#8997=ORIENTED_EDGE ( 'NONE', *, *, #19932, .T. ) ;
#9001=ORIENTED_EDGE ( 'NONE', *, *, #20522, .F. ) ;
#9002=DIRECTION ( 'NONE',  ( 0.000000000000000000, 1.131431318426415506E-52, 1.000000000000000000 ) ) ;
#9003=EDGE_LOOP ( 'NONE', ( #25021, #22402, #12918, #7532 ) ) ;
#9004=ORIENTED_EDGE ( 'NONE', *, *, #6942, .T. ) ;
#9005=DIRECTION ( 'NONE',  ( 1.000000000000000000, 0.000000000000000000, -5.546364386991661285E-52 ) ) ;
#9010=DIRECTION ( 'NONE',  ( -1.000000000000000000, 0.000000000000000000, 1.848892746611746966E-32 ) ) ;
#9011=ORIENTED_EDGE ( 'NONE', *, *, #17660, .T. ) ;
#9016=CARTESIAN_POINT ( 'NONE',  ( 11.99999999999999645, 144.9999999999999716, -186.9999999999999716 ) ) ;
#9020=LINE ( 'NONE', #3835, #13023 ) ;
#9022=CARTESIAN_POINT ( 'NONE',  ( -500.0000000000000000, -137.0000000000000000, 155.0000000000000000 ) ) ;
#9024=CYLINDRICAL_SURFACE ( 'NONE', #2413, 4.750000000000004441 ) ;
#9025=ORIENTED_EDGE ( 'NONE', *, *, #21585, .T. ) ;
#9026=FACE_OUTER_BOUND ( 'NONE', #1019, .T. ) ;
#9027=ORIENTED_EDGE ( 'NONE', *, *, #18044, .T. ) ;
#9029=DIRECTION ( 'NONE',  ( 0.000000000000000000, 1.224646799147353207E-16, -1.000000000000000000 ) ) ;
#9034=CARTESIAN_POINT ( 'NONE',  ( -449.9999999999999432, 105.0000000000000142, -77.99999999999997158 ) ) ;
#9036=EDGE_LOOP ( 'NONE', ( #23182, #101, #10298, #32927 ) ) ;
#9044=VECTOR ( 'NONE', #25918, 1000.000000000000000 ) ;
#9051=( NAMED_UNIT ( * ) PLANE_ANGLE_UNIT ( ) SI_UNIT ( $, .RADIAN. ) );
#9052=EDGE_CURVE ( 'NONE', #31799, #32157, #22649, .T. ) ;
#9057=VERTEX_POINT ( 'NONE', #1618 ) ;
#9060=DIRECTION ( 'NONE',  ( 0.000000000000000000, 0.000000000000000000, 1.000000000000000000 ) ) ;
#9061=ORIENTED_EDGE ( 'NONE', *, *, #31648, .T. ) ;
#9065=AXIS2_PLACEMENT_3D ( 'NONE', #15626, #26459, #23796 ) ;
#9066=VERTEX_POINT ( 'NONE', #31176 ) ;
#9067=DIRECTION ( 'NONE',  ( -1.000000000000000000, 0.000000000000000000, 0.000000000000000000 ) ) ;
#9068=DIRECTION ( 'NONE',  ( 1.000000000000000000, 0.000000000000000000, 0.000000000000000000 ) ) ;
#9069=ORIENTED_EDGE ( 'NONE', *, *, #17948, .F. ) ;
#9073=CIRCLE ( 'NONE', #8506, 2.000000000000001776 ) ;
#9075=CARTESIAN_POINT ( 'NONE',  ( -361.0000000000000000, -125.0000000000000284, 181.0000000000000000 ) ) ;
#9084=ADVANCED_FACE ( 'NONE', ( #34185 ), #20491, .T. ) ;
#9085=LINE ( 'NONE', #33293, #6713 ) ;
#9086=EDGE_CURVE ( 'NONE', #34350, #31695, #29419, .T. ) ;
#9088=ADVANCED_FACE ( 'NONE', ( #1449 ), #11799, .T. ) ;
#9089=EDGE_LOOP ( 'NONE', ( #3233, #23049, #12736, #34475, #4519, #4512, #1182, #10642 ) ) ;
#9090=CARTESIAN_POINT ( 'NONE',  ( -442.0000000000000000, 104.9999999999999858, -187.0000000000000000 ) ) ;
#9094=CARTESIAN_POINT ( 'NONE',  ( 19.99999999999998934, -145.0000000000000000, 162.9999999999999716 ) ) ;
#9096=VERTEX_POINT ( 'NONE', #9634 ) ;
#9098=DIRECTION ( 'NONE',  ( -0.000000000000000000, -1.000000000000000000, -0.000000000000000000 ) ) ;
#9101=DIRECTION ( 'NONE',  ( 0.000000000000000000, 1.131431318426415506E-52, 1.000000000000000000 ) ) ;
#9108=CARTESIAN_POINT ( 'NONE',  ( 19.99999999999998934, -115.0000000000000000, -155.0000000000000284 ) ) ;
#9109=FACE_OUTER_BOUND ( 'NONE', #31764, .T. ) ;
#9111=DIRECTION ( 'NONE',  ( -1.000000000000000000, 0.000000000000000000, 0.000000000000000000 ) ) ;
#9113=EDGE_LOOP ( 'NONE', ( #7463, #9681, #19053, #14479 ) ) ;
#9116=VECTOR ( 'NONE', #33112, 1000.000000000000000 ) ;
#9119=VECTOR ( 'NONE', #20275, 1000.000000000000000 ) ;
#9122=ORIENTED_EDGE ( 'NONE', *, *, #33628, .T. ) ;
#9123=CARTESIAN_POINT ( 'NONE',  ( 19.99999999999998934, -145.0000000000000000, 187.0000000000000000 ) ) ;
#9126=CARTESIAN_POINT ( 'NONE',  ( -12.00000000000001066, 134.9999999999998863, 155.0000000000000000 ) ) ;
#9127=ORIENTED_EDGE ( 'NONE', *, *, #22428, .T. ) ;
#9128=DIRECTION ( 'NONE',  ( -0.000000000000000000, -0.000000000000000000, -1.000000000000000000 ) ) ;
#9129=FACE_OUTER_BOUND ( 'NONE', #25219, .T. ) ;
#9135=CARTESIAN_POINT ( 'NONE',  ( -500.0000000000000000, 112.9999999999999574, 155.0000000000000000 ) ) ;
#9139=ORIENTED_EDGE ( 'NONE', *, *, #9673, .T. ) ;
#9141=CARTESIAN_POINT ( 'NONE',  ( 19.99999999999998934, -32.99999999999997158, -154.9999999999999716 ) ) ;
#9157=VERTEX_POINT ( 'NONE', #18548 ) ;
#9161=EDGE_CURVE ( 'NONE', #19763, #32511, #22588, .T. ) ;
#9169=ORIENTED_EDGE ( 'NONE', *, *, #33540, .T. ) ;
#9170=CARTESIAN_POINT ( 'NONE',  ( -410.0000000000000568, -124.9999999999999716, 132.0000000000000000 ) ) ;
#9177=CIRCLE ( 'NONE', #6873, 7.999999999999979572 ) ;
#9178=DIRECTION ( 'NONE',  ( -0.000000000000000000, 0.000000000000000000, -1.000000000000000000 ) ) ;
#9179=ORIENTED_EDGE ( 'NONE', *, *, #17332, .T. ) ;
#9182=CARTESIAN_POINT ( 'NONE',  ( -410.0000000000000568, -125.0000000000000000, 187.0000000000000000 ) ) ;
#9186=DIRECTION ( 'NONE',  ( -0.000000000000000000, 1.000000000000000000, -0.000000000000000000 ) ) ;
#9188=DIRECTION ( 'NONE',  ( 0.000000000000000000, -1.000000000000000000, 3.374343856708137958E-53 ) ) ;
#9194=CARTESIAN_POINT ( 'NONE',  ( -70.00000000000000000, 75.55999999999990280, 172.9900000000000091 ) ) ;
#9195=VECTOR ( 'NONE', #10007, 1000.000000000000000 ) ;
#9196=EDGE_CURVE ( 'NONE', #25155, #23608, #8402, .T. ) ;
#9197=PLANE ( 'NONE',  #13231 ) ;
#9198=ORIENTED_EDGE ( 'NONE', *, *, #13058, .T. ) ;
#9200=DIRECTION ( 'NONE',  ( 1.000000000000000000, 0.000000000000000000, 1.300283923313630633E-47 ) ) ;
#9203=DIRECTION ( 'NONE',  ( 0.000000000000000000, -0.000000000000000000, -1.000000000000000000 ) ) ;
#9204=VECTOR ( 'NONE', #3200, 1000.000000000000000 ) ;
#9206=ORIENTED_EDGE ( 'NONE', *, *, #20665, .F. ) ;
#9208=CARTESIAN_POINT ( 'NONE',  ( -445.9999999999999432, -125.0000000000000000, 107.9999999999999858 ) ) ;
#9209=AXIS2_PLACEMENT_3D ( 'NONE', #33793, #3875, #19750 ) ;
#9211=CARTESIAN_POINT ( 'NONE',  ( -445.9999999999999432, 105.0000000000000142, -101.9999999999999858 ) ) ;
#9212=VECTOR ( 'NONE', #30435, 1000.000000000000000 ) ;
#9213=ORIENTED_EDGE ( 'NONE', *, *, #2461, .T. ) ;
#9215=CARTESIAN_POINT ( 'NONE',  ( -15.99999999999998579, 75.55999999999990280, 177.7400000000000091 ) ) ;
#9216=VERTEX_POINT ( 'NONE', #4610 ) ;
#9220=DIRECTION ( 'NONE',  ( -1.000000000000000000, 0.000000000000000000, 0.000000000000000000 ) ) ;
#9226=CARTESIAN_POINT ( 'NONE',  ( -19.99999999999998934, -134.9999999999999716, 187.0000000000000000 ) ) ;
#9227=FACE_OUTER_BOUND ( 'NONE', #28123, .T. ) ;
#9229=DIRECTION ( 'NONE',  ( 0.000000000000000000, 0.000000000000000000, 1.000000000000000000 ) ) ;
#9232=ORIENTED_EDGE ( 'NONE', *, *, #3023, .T. ) ;
#9233=PLANE ( 'NONE',  #24246 ) ;
#9236=ORIENTED_EDGE ( 'NONE', *, *, #7817, .F. ) ;
#9238=DIRECTION ( 'NONE',  ( 0.000000000000000000, 1.000000000000000000, 5.145227585319922065E-49 ) ) ;
#9241=EDGE_CURVE ( 'NONE', #4681, #27224, #24018, .T. ) ;
#9243=LINE ( 'NONE', #32911, #7777 ) ;
#9246=VERTEX_POINT ( 'NONE', #21374 ) ;
#9248=DIRECTION ( 'NONE',  ( 1.000000000000000000, 0.000000000000000000, 0.000000000000000000 ) ) ;
#9252=CARTESIAN_POINT ( 'NONE',  ( 11.99999999999999645, 144.9999999999999716, -158.9999999999999716 ) ) ;
#9254=ORIENTED_EDGE ( 'NONE', *, *, #19106, .T. ) ;
#9255=VERTEX_POINT ( 'NONE', #28845 ) ;
#9256=AXIS2_PLACEMENT_3D ( 'NONE', #27752, #11220, #16398 ) ;
#9257=AXIS2_PLACEMENT_3D ( 'NONE', #33498, #13942, #24952 ) ;
#9261=CARTESIAN_POINT ( 'NONE',  ( -365.0000000000000000, -131.0000000000000000, 126.0000000000000000 ) ) ;
#9262=DIRECTION ( 'NONE',  ( 0.000000000000000000, 1.000000000000000000, 1.310824597558155437E-49 ) ) ;
#9264=VERTEX_POINT ( 'NONE', #1787 ) ;
#9271=ORIENTED_EDGE ( 'NONE', *, *, #11727, .T. ) ;
#9273=CARTESIAN_POINT ( 'NONE',  ( -12.00000000000001066, -145.0000000000000000, 194.9999999999999716 ) ) ;
#9275=EDGE_CURVE ( 'NONE', #14377, #25358, #7293, .T. ) ;
#9277=FACE_BOUND ( 'NONE', #26803, .T. ) ;
#9282=AXIS2_PLACEMENT_3D ( 'NONE', #33573, #9200, #30915 ) ;
#9283=AXIS2_PLACEMENT_3D ( 'NONE', #32602, #8408, #19281 ) ;
#9284=VERTEX_POINT ( 'NONE', #12844 ) ;
#9294=LINE ( 'NONE', #11142, #14835 ) ;
#9296=CARTESIAN_POINT ( 'NONE',  ( 11.99999999999999645, -145.0000000000000000, -190.9999999999999432 ) ) ;
#9300=VECTOR ( 'NONE', #922, 1000.000000000000000 ) ;
#9302=ORIENTED_EDGE ( 'NONE', *, *, #11924, .F. ) ;
#9305=VECTOR ( 'NONE', #25609, 1000.000000000000000 ) ;
#9315=ORIENTED_EDGE ( 'NONE', *, *, #23237, .F. ) ;
#9318=LINE ( 'NONE', #17699, #29534 ) ;
#9323=DIRECTION ( 'NONE',  ( -3.040835319149746528E-31, -1.000000000000000000, 0.000000000000000000 ) ) ;
#9324=CIRCLE ( 'NONE', #34887, 7.999999999999979572 ) ;
#9327=CARTESIAN_POINT ( 'NONE',  ( 11.99999999999999645, 140.9999999999999716, -155.0000000000000000 ) ) ;
#9329=CARTESIAN_POINT ( 'NONE',  ( -12.00000000000001066, 144.9999999999999716, 187.0000000000000000 ) ) ;
#9330=EDGE_CURVE ( 'NONE', #20393, #34350, #5502, .T. ) ;
#9335=AXIS2_PLACEMENT_3D ( 'NONE', #1109, #30832, #17327 ) ;
#9338=AXIS2_PLACEMENT_3D ( 'NONE', #3631, #25703, #28557 ) ;
#9339=CARTESIAN_POINT ( 'NONE',  ( 11.99999999999999645, -145.0000000000000000, 194.9999999999999716 ) ) ;
#9340=ORIENTED_EDGE ( 'NONE', *, *, #11464, .F. ) ;
#9341=FACE_OUTER_BOUND ( 'NONE', #22628, .T. ) ;
#9344=AXIS2_PLACEMENT_3D ( 'NONE', #770, #11637, #22487 ) ;
#9351=FACE_OUTER_BOUND ( 'NONE', #24890, .T. ) ;
#9355=CARTESIAN_POINT ( 'NONE',  ( -365.0000000000000000, 132.9999999999999716, 126.0000000000000000 ) ) ;
#9358=DIRECTION ( 'NONE',  ( 1.000000000000000000, 0.000000000000000000, -1.848892746611746966E-32 ) ) ;
#9363=ADVANCED_FACE ( 'NONE', ( #5672 ), #8180, .F. ) ;
#9368=DIRECTION ( 'NONE',  ( -1.000000000000000000, 0.000000000000000000, 0.000000000000000000 ) ) ;
#9369=DIRECTION ( 'NONE',  ( 1.000000000000000000, 0.000000000000000000, -1.848892746611746966E-32 ) ) ;
#9370=DIRECTION ( 'NONE',  ( -0.000000000000000000, -0.000000000000000000, 1.000000000000000000 ) ) ;
#9372=ADVANCED_FACE ( 'NONE', ( #16573 ), #8535, .F. ) ;
#9373=DIRECTION ( 'NONE',  ( 1.232595164407830946E-32, 0.000000000000000000, 1.000000000000000000 ) ) ;
#9374=DIRECTION ( 'NONE',  ( 0.000000000000000000, 0.000000000000000000, -1.000000000000000000 ) ) ;
#9378=DIRECTION ( 'NONE',  ( 0.000000000000000000, 0.000000000000000000, 1.000000000000000000 ) ) ;
#9379=CARTESIAN_POINT ( 'NONE',  ( -365.0000000000000000, -119.0000000000000000, 109.9999999999999858 ) ) ;
#9380=FACE_BOUND ( 'NONE', #24612, .T. ) ;
#9382=VECTOR ( 'NONE', #10222, 1000.000000000000000 ) ;
#9383=EDGE_CURVE ( 'NONE', #11080, #13888, #23748, .T. ) ;
#9385=DIRECTION ( 'NONE',  ( 1.000000000000000000, 0.000000000000000000, 0.000000000000000000 ) ) ;
#9387=LINE ( 'NONE', #25030, #287 ) ;
#9391=AXIS2_PLACEMENT_3D ( 'NONE', #8669, #19897, #25389 ) ;
#9392=ORIENTED_EDGE ( 'NONE', *, *, #3056, .T. ) ;
#9396=DIRECTION ( 'NONE',  ( 0.000000000000000000, -2.309213040847544338E-50, -1.000000000000000000 ) ) ;
#9400=CARTESIAN_POINT ( 'NONE',  ( -449.9999999999999432, -105.0000000000000142, -77.99999999999997158 ) ) ;
#9401=VERTEX_POINT ( 'NONE', #32386 ) ;
#9404=DIRECTION ( 'NONE',  ( 0.000000000000000000, 0.000000000000000000, 1.000000000000000000 ) ) ;
#9406=CIRCLE ( 'NONE', #8806, 4.750000000000004441 ) ;
#9407=DIRECTION ( 'NONE',  ( 0.000000000000000000, 2.309213040847544338E-50, 1.000000000000000000 ) ) ;
#9408=DIRECTION ( 'NONE',  ( -1.000000000000000000, 0.000000000000000000, 0.000000000000000000 ) ) ;
#9409=ORIENTED_EDGE ( 'NONE', *, *, #18470, .T. ) ;
#9412=AXIS2_PLACEMENT_3D ( 'NONE', #17582, #28419, #25738 ) ;
#9414=EDGE_CURVE ( 'NONE', #12936, #980, #21548, .T. ) ;
#9415=DIRECTION ( 'NONE',  ( -0.000000000000000000, 1.000000000000000000, -0.000000000000000000 ) ) ;
#9417=LINE ( 'NONE', #12445, #25272 ) ;
#9418=CARTESIAN_POINT ( 'NONE',  ( -500.0000000000000000, -113.0000000000000000, 155.0000000000000000 ) ) ;
#9419=AXIS2_PLACEMENT_3D ( 'NONE', #2070, #15092, #34466 ) ;
#9420=CARTESIAN_POINT ( 'NONE',  ( -430.0000000000000000, 118.9999999999999716, 109.9999999999999858 ) ) ;
#9423=EDGE_CURVE ( 'NONE', #8068, #14037, #12963, .T. ) ;
#9428=FACE_OUTER_BOUND ( 'NONE', #20626, .T. ) ;
#9429=CARTESIAN_POINT ( 'NONE',  ( -12.00000000000001066, 144.9999999999999716, -194.9999999999999432 ) ) ;
#9431=LINE ( 'NONE', #31139, #4397 ) ;
#9432=( LENGTH_UNIT ( ) NAMED_UNIT ( * ) SI_UNIT ( .MILLI., .METRE. ) );
#9436=DIRECTION ( 'NONE',  ( -1.232595164407830946E-32, -3.421138828918010427E-49, 1.000000000000000000 ) ) ;
#9437=EDGE_CURVE ( 'NONE', #15497, #5208, #9431, .T. ) ;
#9438=DIRECTION ( 'NONE',  ( 0.000000000000000000, 1.000000000000000000, 1.224646799147353207E-16 ) ) ;
#9444=VERTEX_POINT ( 'NONE', #3722 ) ;
#9449=CIRCLE ( 'NONE', #7157, 7.999999999999979572 ) ;
#9452=VERTEX_POINT ( 'NONE', #25607 ) ;
#9453=DIRECTION ( 'NONE',  ( 0.000000000000000000, -7.888609052210118054E-31, -1.000000000000000000 ) ) ;
#9455=VECTOR ( 'NONE', #2559, 1000.000000000000000 ) ;
#9456=CARTESIAN_POINT ( 'NONE',  ( -499.9999999999999432, 108.9999999999999858, -187.0000000000000000 ) ) ;
#9457=DIRECTION ( 'NONE',  ( 0.000000000000000000, 1.000000000000000000, 0.000000000000000000 ) ) ;
#9459=ORIENTED_EDGE ( 'NONE', *, *, #426, .T. ) ;
#9465=DIRECTION ( 'NONE',  ( 0.000000000000000000, 0.000000000000000000, 1.000000000000000000 ) ) ;
#9466=VERTEX_POINT ( 'NONE', #11933 ) ;
#9468=CARTESIAN_POINT ( 'NONE',  ( -499.9999999999999432, 136.9999999999999432, -162.9999999999999716 ) ) ;
#9471=DIRECTION ( 'NONE',  ( 0.000000000000000000, 0.000000000000000000, -1.000000000000000000 ) ) ;
#9473=DIRECTION ( 'NONE',  ( 0.000000000000000000, 1.000000000000000000, -2.309213040847544338E-50 ) ) ;
#9475=ORIENTED_EDGE ( 'NONE', *, *, #21255, .F. ) ;
#9482=VERTEX_POINT ( 'NONE', #28462 ) ;
#9485=DIRECTION ( 'NONE',  ( 0.000000000000000000, 2.309213040847544338E-50, 1.000000000000000000 ) ) ;
#9486=ORIENTED_EDGE ( 'NONE', *, *, #23530, .T. ) ;
#9487=ORIENTED_EDGE ( 'NONE', *, *, #33279, .F. ) ;
#9490=DIRECTION ( 'NONE',  ( 0.000000000000000000, 0.000000000000000000, 1.000000000000000000 ) ) ;
#9491=VECTOR ( 'NONE', #10034, 1000.000000000000000 ) ;
#9493=DIRECTION ( 'NONE',  ( 0.000000000000000000, -1.000000000000000000, 0.000000000000000000 ) ) ;
#9494=FACE_OUTER_BOUND ( 'NONE', #11208, .T. ) ;
#9496=VERTEX_POINT ( 'NONE', #30611 ) ;
#9497=CARTESIAN_POINT ( 'NONE',  ( -19.99999999999998934, 112.9999999999999574, 155.0000000000000000 ) ) ;
#9498=DIRECTION ( 'NONE',  ( -1.000000000000000000, 0.000000000000000000, 0.000000000000000000 ) ) ;
#9501=DIRECTION ( 'NONE',  ( 1.000000000000000000, 0.000000000000000000, 0.000000000000000000 ) ) ;
#9503=DIRECTION ( 'NONE',  ( 0.000000000000000000, 0.000000000000000000, 1.000000000000000000 ) ) ;
#9510=DIRECTION ( 'NONE',  ( 1.000000000000000000, 0.000000000000000000, 0.000000000000000000 ) ) ;
#9517=EDGE_LOOP ( 'NONE', ( #468, #8345, #25002, #17879 ) ) ;
#9521=VECTOR ( 'NONE', #9369, 1000.000000000000000 ) ;
#9522=EDGE_LOOP ( 'NONE', ( #15414, #11002, #5444, #34777 ) ) ;
#9524=LINE ( 'NONE', #17721, #19432 ) ;
#9526=EDGE_CURVE ( 'NONE', #25899, #20834, #11574, .T. ) ;
#9528=AXIS2_PLACEMENT_3D ( 'NONE', #2876, #19806, #32601 ) ;
#9531=EDGE_LOOP ( 'NONE', ( #21872, #11708, #13263, #20041 ) ) ;
#9532=EDGE_LOOP ( 'NONE', ( #31156, #9392, #27208, #1319 ) ) ;
#9536=( GEOMETRIC_REPRESENTATION_CONTEXT ( 3 ) GLOBAL_UNCERTAINTY_ASSIGNED_CONTEXT ( ( #12745 ) ) GLOBAL_UNIT_ASSIGNED_CONTEXT ( ( #33072, #9051, #30761 ) ) REPRESENTATION_CONTEXT ( 'NONE', 'WORKASPACE' ) );
#9538=DIRECTION ( 'NONE',  ( 0.000000000000000000, 0.000000000000000000, 1.000000000000000000 ) ) ;
#9539=CARTESIAN_POINT ( 'NONE',  ( -418.0000000000000000, 105.0000000000000000, -73.99999999999998579 ) ) ;
#9540=ADVANCED_FACE ( 'NONE', ( #33624 ), #20113, .F. ) ;
#9541=ORIENTED_EDGE ( 'NONE', *, *, #19499, .T. ) ;
#9543=ORIENTED_EDGE ( 'NONE', *, *, #34846, .T. ) ;
#9545=DIRECTION ( 'NONE',  ( 0.000000000000000000, -6.123233995736766036E-17, -1.000000000000000000 ) ) ;
#9546=CARTESIAN_POINT ( 'NONE',  ( -365.0000000000000000, 134.9999999999999716, 126.0000000000000000 ) ) ;
#9549=CARTESIAN_POINT ( 'NONE',  ( -418.0000000000000000, 137.0000000000000000, -175.0000000000000000 ) ) ;
#9550=CIRCLE ( 'NONE', #26982, 4.000000000000003553 ) ;
#9558=AXIS2_PLACEMENT_3D ( 'NONE', #23993, #32196, #23833 ) ;
#9559=AXIS2_PLACEMENT_3D ( 'NONE', #26876, #24202, #26166 ) ;
#9560=CARTESIAN_POINT ( 'NONE',  ( -349.0000000000000000, -125.0000000000000284, 183.0000000000000000 ) ) ;
#9562=CARTESIAN_POINT ( 'NONE',  ( 11.99999999999999645, -124.9999999999999432, -154.9999999999999716 ) ) ;
#9564=VECTOR ( 'NONE', #8604, 1000.000000000000000 ) ;
#9568=CARTESIAN_POINT ( 'NONE',  ( 11.99999999999999645, 134.9999999999999432, -186.9999999999999716 ) ) ;
#9570=ORIENTED_EDGE ( 'NONE', *, *, #29949, .T. ) ;
#9577=VECTOR ( 'NONE', #26502, 1000.000000000000000 ) ;
#9582=ORIENTED_EDGE ( 'NONE', *, *, #1751, .T. ) ;
#9583=EDGE_CURVE ( 'NONE', #10395, #7236, #10674, .T. ) ;
#9584=EDGE_LOOP ( 'NONE', ( #813, #33558 ) ) ;
#9585=AXIS2_PLACEMENT_3D ( 'NONE', #10844, #2822, #24186 ) ;
#9586=VERTEX_POINT ( 'NONE', #16336 ) ;
#9588=CARTESIAN_POINT ( 'NONE',  ( -355.0000000000000000, -131.0000000000000000, 128.0000000000000000 ) ) ;
#9590=CARTESIAN_POINT ( 'NONE',  ( -12.00000000000001066, -56.99999999999997868, 154.9999999999999716 ) ) ;
#9598=CARTESIAN_POINT ( 'NONE',  ( -19.99999999999996092, -141.0000000000000000, 162.9999999999999716 ) ) ;
#9600=DIRECTION ( 'NONE',  ( 0.000000000000000000, 1.000000000000000000, 5.053935297177146739E-49 ) ) ;
#9601=ORIENTED_EDGE ( 'NONE', *, *, #130, .F. ) ;
#9602=DIRECTION ( 'NONE',  ( 0.000000000000000000, -3.374343856708137958E-53, 1.000000000000000000 ) ) ;
#9603=EDGE_CURVE ( 'NONE', #31232, #27516, #16376, .T. ) ;
#9611=EDGE_CURVE ( 'NONE', #25692, #10763, #19704, .T. ) ;
#9612=ORIENTED_EDGE ( 'NONE', *, *, #30090, .T. ) ;
#9616=DIRECTION ( 'NONE',  ( 0.000000000000000000, 0.000000000000000000, 1.000000000000000000 ) ) ;
#9617=AXIS2_PLACEMENT_3D ( 'NONE', #29542, #22549, #32204 ) ;
#9618=CARTESIAN_POINT ( 'NONE',  ( -418.0000000000000568, -105.0000000000000142, 159.0000000000000000 ) ) ;
#9620=CARTESIAN_POINT ( 'NONE',  ( -20.00000000000001776, -124.9999999999999432, -162.9999999999999432 ) ) ;
#9622=VECTOR ( 'NONE', #32319, 1000.000000000000000 ) ;
#9623=DIRECTION ( 'NONE',  ( 0.000000000000000000, 1.000000000000000000, 5.053935297177146739E-49 ) ) ;
#9624=FACE_OUTER_BOUND ( 'NONE', #33796, .T. ) ;
#9625=ORIENTED_EDGE ( 'NONE', *, *, #12360, .T. ) ;
#9630=ORIENTED_EDGE ( 'NONE', *, *, #33754, .F. ) ;
#9633=ORIENTED_EDGE ( 'NONE', *, *, #34600, .F. ) ;
#9634=CARTESIAN_POINT ( 'NONE',  ( -414.0000000000000000, -105.0000000000000142, 132.0000000000000000 ) ) ;
#9636=FACE_OUTER_BOUND ( 'NONE', #8476, .T. ) ;
#9645=DIRECTION ( 'NONE',  ( 0.000000000000000000, -1.224646799147353207E-16, 1.000000000000000000 ) ) ;
#9646=FACE_OUTER_BOUND ( 'NONE', #21186, .T. ) ;
#9647=ORIENTED_EDGE ( 'NONE', *, *, #10587, .T. ) ;
#9649=VERTEX_POINT ( 'NONE', #24663 ) ;
#9650=AXIS2_PLACEMENT_3D ( 'NONE', #20709, #33704, #7159 ) ;
#9652=ORIENTED_EDGE ( 'NONE', *, *, #31968, .T. ) ;
#9654=ORIENTED_EDGE ( 'NONE', *, *, #18230, .T. ) ;
#9655=FACE_OUTER_BOUND ( 'NONE', #34843, .T. ) ;
#9657=DIRECTION ( 'NONE',  ( 0.000000000000000000, -1.000000000000000000, 6.123233995736766036E-17 ) ) ;
#9658=CARTESIAN_POINT ( 'NONE',  ( 0.000000000000000000, -115.0000000000000000, 0.000000000000000000 ) ) ;
#9659=ORIENTED_EDGE ( 'NONE', *, *, #34677, .F. ) ;
#9660=ORIENTED_EDGE ( 'NONE', *, *, #26542, .F. ) ;
#9661=PLANE ( 'NONE',  #32181 ) ;
#9662=DIRECTION ( 'NONE',  ( 0.000000000000000000, -2.309213040847544338E-50, -1.000000000000000000 ) ) ;
#9664=LINE ( 'NONE', #7151, #15977 ) ;
#9666=ORIENTED_EDGE ( 'NONE', *, *, #34712, .F. ) ;
#9668=DIRECTION ( 'NONE',  ( -2.530127506375325574E-80, 1.000000000000000000, 6.842277657836020854E-49 ) ) ;
#9669=FACE_OUTER_BOUND ( 'NONE', #11735, .T. ) ;
#9670=ORIENTED_EDGE ( 'NONE', *, *, #12341, .T. ) ;
#9673=EDGE_CURVE ( 'NONE', #26771, #33889, #20930, .T. ) ;
#9676=DIRECTION ( 'NONE',  ( 0.000000000000000000, 0.000000000000000000, -1.000000000000000000 ) ) ;
#9678=CARTESIAN_POINT ( 'NONE',  ( -12.00000000000001066, 134.9999999999998863, 162.9999999999999716 ) ) ;
#9679=ADVANCED_FACE ( 'NONE', ( #13827 ), #2782, .T. ) ;
#9681=ORIENTED_EDGE ( 'NONE', *, *, #18034, .T. ) ;
#9684=CYLINDRICAL_SURFACE ( 'NONE', #20618, 4.750000000000004441 ) ;
#9688=LINE ( 'NONE', #20550, #14305 ) ;
#9690=ORIENTED_EDGE ( 'NONE', *, *, #27157, .T. ) ;
#9691=CARTESIAN_POINT ( 'NONE',  ( -414.0000000000000568, -137.0000000000000000, 154.9999999999999716 ) ) ;
#9692=ORIENTED_EDGE ( 'NONE', *, *, #27854, .F. ) ;
#9693=ORIENTED_EDGE ( 'NONE', *, *, #234, .F. ) ;
#9698=DIRECTION ( 'NONE',  ( 0.000000000000000000, 5.145227585319922065E-49, 1.000000000000000000 ) ) ;
#9699=ORIENTED_EDGE ( 'NONE', *, *, #18980, .F. ) ;
#9700=ORIENTED_EDGE ( 'NONE', *, *, #22833, .F. ) ;
#9705=DIRECTION ( 'NONE',  ( 0.000000000000000000, -2.309213040847544338E-50, -1.000000000000000000 ) ) ;
#9709=ORIENTED_EDGE ( 'NONE', *, *, #10622, .F. ) ;
#9713=CARTESIAN_POINT ( 'NONE',  ( -15.99999999999998579, 75.55999999999990280, 172.9900000000000091 ) ) ;
#9714=EDGE_CURVE ( 'NONE', #24468, #26932, #5788, .T. ) ;
#9717=DIRECTION ( 'NONE',  ( 0.000000000000000000, 1.000000000000000000, 1.224646799147353207E-16 ) ) ;
#9718=ORIENTED_EDGE ( 'NONE', *, *, #12979, .T. ) ;
#9722=CARTESIAN_POINT ( 'NONE',  ( -442.0000000000000000, -125.0000000000000000, 104.0000000000000142 ) ) ;
#9723=FACE_OUTER_BOUND ( 'NONE', #16217, .T. ) ;
#9724=EDGE_CURVE ( 'NONE', #7256, #23038, #27520, .T. ) ;
#9725=AXIS2_PLACEMENT_3D ( 'NONE', #26417, #20562, #23580 ) ;
#9726=ORIENTED_EDGE ( 'NONE', *, *, #11608, .T. ) ;
#9729=CARTESIAN_POINT ( 'NONE',  ( -418.0000000000000000, -105.0000000000000142, -73.99999999999998579 ) ) ;
#9730=DIRECTION ( 'NONE',  ( 0.000000000000000000, 1.000000000000000000, 2.309213040847544338E-50 ) ) ;
#9731=EDGE_CURVE ( 'NONE', #196, #27359, #34007, .T. ) ;
#9733=VECTOR ( 'NONE', #8741, 1000.000000000000000 ) ;
#9737=VERTEX_POINT ( 'NONE', #3904 ) ;
#9739=ORIENTED_EDGE ( 'NONE', *, *, #1120, .F. ) ;
#9742=LINE ( 'NONE', #12599, #32320 ) ;
#9743=DIRECTION ( 'NONE',  ( -0.000000000000000000, -0.000000000000000000, -1.000000000000000000 ) ) ;
#9748=AXIS2_PLACEMENT_3D ( 'NONE', #14503, #25333, #9503 ) ;
#9750=DIRECTION ( 'NONE',  ( 0.000000000000000000, 0.000000000000000000, -1.000000000000000000 ) ) ;
#9754=DIRECTION ( 'NONE',  ( -3.469446951953832974E-18, -1.000000000000000000, -7.888609052210116302E-31 ) ) ;
#9755=CARTESIAN_POINT ( 'NONE',  ( -445.9999999999999432, 124.9999999999999574, -187.0000000000000000 ) ) ;
#9759=AXIS2_PLACEMENT_3D ( 'NONE', #19288, #27630, #30487 ) ;
#9763=CARTESIAN_POINT ( 'NONE',  ( -445.9999999999999432, -124.9999999999999716, 132.0000000000000000 ) ) ;
#9766=VECTOR ( 'NONE', #22777, 1000.000000000000000 ) ;
#9771=EDGE_CURVE ( 'NONE', #15713, #13338, #14626, .T. ) ;
#9773=CARTESIAN_POINT ( 'NONE',  ( 12.00000000000001066, 144.9999999999999716, -154.9999999999999716 ) ) ;
#9780=EDGE_CURVE ( 'NONE', #23416, #5771, #22791, .T. ) ;
#9784=VECTOR ( 'NONE', #18154, 1000.000000000000000 ) ;
#9785=ORIENTED_EDGE ( 'NONE', *, *, #2767, .T. ) ;
#9787=DIRECTION ( 'NONE',  ( -0.000000000000000000, -1.000000000000000000, -0.000000000000000000 ) ) ;
#9788=CARTESIAN_POINT ( 'NONE',  ( -418.0000000000000568, 141.0000000000000000, -155.0000000000000000 ) ) ;
#9790=EDGE_CURVE ( 'NONE', #26110, #2088, #12126, .T. ) ;
#9795=CARTESIAN_POINT ( 'NONE',  ( -12.00000000000001066, 124.9999999999999716, 162.9999999999999716 ) ) ;
#9797=EDGE_CURVE ( 'NONE', #24623, #24780, #9085, .T. ) ;
#9801=DIRECTION ( 'NONE',  ( 0.000000000000000000, 1.131431318426415506E-52, 1.000000000000000000 ) ) ;
#9803=VERTEX_POINT ( 'NONE', #30628 ) ;
#9807=CARTESIAN_POINT ( 'NONE',  ( -365.0000000000000000, -125.0000000000000000, 113.9999999999999858 ) ) ;
#9808=CARTESIAN_POINT ( 'NONE',  ( -449.9999999999999432, -125.0000000000000000, 107.9999999999999858 ) ) ;
#9812=DIRECTION ( 'NONE',  ( -1.000000000000000000, 0.000000000000000000, 0.000000000000000000 ) ) ;
#9814=CARTESIAN_POINT ( 'NONE',  ( -20.00000000000001776, -141.0000000000000000, -186.9999999999999716 ) ) ;
#9817=ORIENTED_EDGE ( 'NONE', *, *, #721, .T. ) ;
#9818=ORIENTED_EDGE ( 'NONE', *, *, #31569, .T. ) ;
#9820=ORIENTED_EDGE ( 'NONE', *, *, #22567, .F. ) ;
#9823=CARTESIAN_POINT ( 'NONE',  ( -19.99999999999998934, -137.0000000000000000, 187.0000000000000000 ) ) ;
#9828=DIRECTION ( 'NONE',  ( 0.000000000000000000, 0.000000000000000000, 1.000000000000000000 ) ) ;
#9829=AXIS2_PLACEMENT_3D ( 'NONE', #21284, #18797, #12577 ) ;
#9832=STYLED_ITEM('',(#35254),#34584);
#9843=CYLINDRICAL_SURFACE ( 'NONE', #9650, 3.999999999999976019 ) ;
#9844=ORIENTED_EDGE ( 'NONE', *, *, #19064, .T. ) ;
#9847=LINE ( 'NONE', #7513, #21205 ) ;
#9849=DIRECTION ( 'NONE',  ( 0.000000000000000000, 0.000000000000000000, 1.000000000000000000 ) ) ;
#9858=CIRCLE ( 'NONE', #17858, 7.999999999999979572 ) ;
#9863=EDGE_CURVE ( 'NONE', #35069, #25265, #12435, .T. ) ;
#9864=ORIENTED_EDGE ( 'NONE', *, *, #12591, .F. ) ;
#9866=DIRECTION ( 'NONE',  ( 0.000000000000000000, 1.000000000000000000, -6.842277657836020854E-49 ) ) ;
#9867=ORIENTED_EDGE ( 'NONE', *, *, #801, .F. ) ;
#9869=DIRECTION ( 'NONE',  ( -0.000000000000000000, 1.000000000000000000, -0.000000000000000000 ) ) ;
#9870=EDGE_CURVE ( 'NONE', #22350, #14078, #10134, .T. ) ;
#9876=ORIENTED_EDGE ( 'NONE', *, *, #11333, .F. ) ;
#9880=CARTESIAN_POINT ( 'NONE',  ( -355.0000000000000000, -117.0000000000000000, 113.9999999999999858 ) ) ;
#9882=CARTESIAN_POINT ( 'NONE',  ( 15.99999999999998579, -32.99999999999997158, -154.9999999999999716 ) ) ;
#9883=EDGE_LOOP ( 'NONE', ( #3072, #28088, #19507, #32124 ) ) ;
#9885=ORIENTED_EDGE ( 'NONE', *, *, #21699, .T. ) ;
#9891=DIRECTION ( 'NONE',  ( 0.000000000000000000, 0.000000000000000000, 1.000000000000000000 ) ) ;
#9896=DIRECTION ( 'NONE',  ( -1.000000000000000000, 0.000000000000000000, 0.000000000000000000 ) ) ;
#9900=DIRECTION ( 'NONE',  ( 1.000000000000000000, 0.000000000000000000, -0.000000000000000000 ) ) ;
#9904=CARTESIAN_POINT ( 'NONE',  ( -445.9999999999999432, -112.9999999999999858, -174.9999999999999716 ) ) ;
#9905=CIRCLE ( 'NONE', #29799, 2.000000000000001776 ) ;
#9907=DIRECTION ( 'NONE',  ( 0.000000000000000000, 0.000000000000000000, -1.000000000000000000 ) ) ;
#9910=AXIS2_PLACEMENT_3D ( 'NONE', #3246, #13764, #7885 ) ;
#9911=EDGE_CURVE ( 'NONE', #32668, #15683, #26146, .T. ) ;
#9912=ORIENTED_EDGE ( 'NONE', *, *, #5681, .T. ) ;
#9915=FACE_OUTER_BOUND ( 'NONE', #30134, .T. ) ;
#9918=CARTESIAN_POINT ( 'NONE',  ( -361.0000000000000000, -125.0000000000000284, 168.9999999999999716 ) ) ;
#9921=FACE_OUTER_BOUND ( 'NONE', #27649, .T. ) ;
#9924=ORIENTED_EDGE ( 'NONE', *, *, #2365, .T. ) ;
#9925=VERTEX_POINT ( 'NONE', #34161 ) ;
#9930=DIRECTION ( 'NONE',  ( -1.000000000000000000, 0.000000000000000000, 0.000000000000000000 ) ) ;
#9931=DIRECTION ( 'NONE',  ( -1.000000000000000000, -3.040835319149746090E-31, -1.232595164407830946E-32 ) ) ;
#9932=CARTESIAN_POINT ( 'NONE',  ( -365.0000000000000000, -133.0000000000000000, 113.9999999999999858 ) ) ;
#9933=DIRECTION ( 'NONE',  ( 0.000000000000000000, 0.000000000000000000, -1.000000000000000000 ) ) ;
#9934=EDGE_LOOP ( 'NONE', ( #4304, #33120, #33762, #2372, #2993, #19662 ) ) ;
#9937=EDGE_CURVE ( 'NONE', #2161, #11922, #25838, .T. ) ;
#9942=VECTOR ( 'NONE', #24909, 1000.000000000000000 ) ;
#9944=ORIENTED_EDGE ( 'NONE', *, *, #1601, .T. ) ;
#9945=DIRECTION ( 'NONE',  ( -3.469446951953832974E-18, -1.000000000000000000, -7.888609052210116302E-31 ) ) ;
#9947=DIRECTION ( 'NONE',  ( -1.300283923313630633E-47, 0.000000000000000000, -1.000000000000000000 ) ) ;
#9951=ORIENTED_EDGE ( 'NONE', *, *, #27804, .T. ) ;
#9952=VECTOR ( 'NONE', #27424, 1000.000000000000000 ) ;
#9955=AXIS2_PLACEMENT_3D ( 'NONE', #7917, #15953, #2057 ) ;
#9956=ORIENTED_EDGE ( 'NONE', *, *, #25260, .F. ) ;
#9957=AXIS2_PLACEMENT_3D ( 'NONE', #9549, #17579, #17410 ) ;
#9959=LINE ( 'NONE', #9123, #21827 ) ;
#9962=EDGE_CURVE ( 'NONE', #9066, #7094, #18169, .T. ) ;
#9964=( GEOMETRIC_REPRESENTATION_CONTEXT ( 3 ) GLOBAL_UNCERTAINTY_ASSIGNED_CONTEXT ( ( #10234 ) ) GLOBAL_UNIT_ASSIGNED_CONTEXT ( ( #3448, #6649, #14342 ) ) REPRESENTATION_CONTEXT ( 'NONE', 'WORKASPACE' ) );
#9967=CARTESIAN_POINT ( 'NONE',  ( -12.00000000000001066, -124.9999999999999432, -162.9999999999999432 ) ) ;
#9968=ORIENTED_EDGE ( 'NONE', *, *, #7606, .T. ) ;
#9973=ORIENTED_EDGE ( 'NONE', *, *, #15306, .F. ) ;
#9978=CARTESIAN_POINT ( 'NONE',  ( -442.0000000000000000, -105.0000000000000142, 132.0000000000000000 ) ) ;
#9984=DIRECTION ( 'NONE',  ( -1.000000000000000000, 0.000000000000000000, 0.000000000000000000 ) ) ;
#9988=CARTESIAN_POINT ( 'NONE',  ( -355.0000000000000000, -119.0000000000000000, 130.0000000000000000 ) ) ;
#9990=VECTOR ( 'NONE', #14470, 1000.000000000000000 ) ;
#9993=EDGE_CURVE ( 'NONE', #7844, #25655, #8991, .T. ) ;
#9995=ORIENTED_EDGE ( 'NONE', *, *, #12636, .F. ) ;
#9997=CARTESIAN_POINT ( 'NONE',  ( -449.9999999999999432, 105.0000000000000142, -101.9999999999999858 ) ) ;
#9999=ORIENTED_EDGE ( 'NONE', *, *, #28452, .T. ) ;
#10000=VERTEX_POINT ( 'NONE', #20304 ) ;
#10001=ORIENTED_EDGE ( 'NONE', *, *, #27373, .F. ) ;
#10003=CIRCLE ( 'NONE', #25941, 3.999999999999982681 ) ;
#10007=DIRECTION ( 'NONE',  ( 0.000000000000000000, 1.000000000000000000, -3.374343856708137958E-53 ) ) ;
#10009=ORIENTED_EDGE ( 'NONE', *, *, #23785, .T. ) ;
#10010=EDGE_CURVE ( 'NONE', #2254, #14577, #22642, .T. ) ;
#10011=EDGE_CURVE ( 'NONE', #31407, #23007, #31316, .T. ) ;
#10019=EDGE_LOOP ( 'NONE', ( #1200, #29014, #18652, #6599 ) ) ;
#10020=DIRECTION ( 'NONE',  ( -0.000000000000000000, 5.145227585319922065E-49, 1.000000000000000000 ) ) ;
#10021=CARTESIAN_POINT ( 'NONE',  ( -12.00000000000001066, 144.9999999999999716, -158.9999999999999716 ) ) ;
#10022=AXIS2_PLACEMENT_3D ( 'NONE', #14888, #11688, #33555 ) ;
#10023=VERTEX_POINT ( 'NONE', #5126 ) ;
#10024=FACE_OUTER_BOUND ( 'NONE', #5946, .T. ) ;
#10025=PLANE ( 'NONE',  #24035 ) ;
#10028=CARTESIAN_POINT ( 'NONE',  ( -430.0000000000000000, -131.0000000000000000, 109.9999999999999858 ) ) ;
#10030=CARTESIAN_POINT ( 'NONE',  ( -361.0000000000000000, -135.0000000000000000, 130.0000000000000000 ) ) ;
#10031=ORIENTED_EDGE ( 'NONE', *, *, #2275, .T. ) ;
#10034=DIRECTION ( 'NONE',  ( -0.000000000000000000, 1.000000000000000000, -0.000000000000000000 ) ) ;
#10037=EDGE_CURVE ( 'NONE', #9496, #21957, #26851, .T. ) ;
#10040=AXIS2_PLACEMENT_3D ( 'NONE', #19504, #18977, #21988 ) ;
#10041=ADVANCED_FACE ( 'NONE', ( #21861 ), #13861, .F. ) ;
#10042=ORIENTED_EDGE ( 'NONE', *, *, #882, .T. ) ;
#10043=ADVANCED_FACE ( 'NONE', ( #27375 ), #32362, .F. ) ;
#10044=EDGE_CURVE ( 'NONE', #32813, #27322, #10127, .T. ) ;
#10047=VERTEX_POINT ( 'NONE', #32717 ) ;
#10048=ORIENTED_EDGE ( 'NONE', *, *, #16649, .T. ) ;
#10051=AXIS2_PLACEMENT_3D ( 'NONE', #13533, #19063, #8362 ) ;
#10052=AXIS2_PLACEMENT_3D ( 'NONE', #4226, #33609, #879 ) ;
#10053=CARTESIAN_POINT ( 'NONE',  ( 19.99999999999998934, 75.55999999999990280, -172.9900000000000091 ) ) ;
#10054=CARTESIAN_POINT ( 'NONE',  ( 12.00000000000001066, -145.0000000000000000, 155.0000000000000000 ) ) ;
#10057=PLANE ( 'NONE',  #19648 ) ;
#10061=CARTESIAN_POINT ( 'NONE',  ( -19.99999999999998934, -32.99999999999997158, 154.9999999999999716 ) ) ;
#10062=PLANE ( 'NONE',  #23361 ) ;
#10063=ORIENTED_EDGE ( 'NONE', *, *, #2125, .T. ) ;
#10065=CARTESIAN_POINT ( 'NONE',  ( -12.00000000000001243, 144.9999999999999716, -154.9999999999999716 ) ) ;
#10066=CYLINDRICAL_SURFACE ( 'NONE', #541, 3.999999999999948042 ) ;
#10067=ORIENTED_EDGE ( 'NONE', *, *, #16761, .F. ) ;
#10068=CARTESIAN_POINT ( 'NONE',  ( -12.00000000000001066, -145.0000000000000000, -186.9999999999999716 ) ) ;
#10069=CARTESIAN_POINT ( 'NONE',  ( 11.99999999999999645, 140.9999999999999716, -175.0000000000000284 ) ) ;
#10071=CARTESIAN_POINT ( 'NONE',  ( -361.0000000000000000, -135.0000000000000000, 110.0000000000000000 ) ) ;
#10072=ORIENTED_EDGE ( 'NONE', *, *, #22901, .T. ) ;
#10073=CARTESIAN_POINT ( 'NONE',  ( -19.99999999999998934, -134.9999999999999716, 187.0000000000000000 ) ) ;
#10074=ORIENTED_EDGE ( 'NONE', *, *, #6784, .F. ) ;
#10075=CARTESIAN_POINT ( 'NONE',  ( 11.99999999999999645, -145.0000000000000000, 162.9999999999999716 ) ) ;
#10077=CARTESIAN_POINT ( 'NONE',  ( -499.9999999999998863, -109.0000000000000142, -187.0000000000000000 ) ) ;
#10079=ADVANCED_FACE ( 'NONE', ( #16374 ), #27204, .F. ) ;
#10083=CARTESIAN_POINT ( 'NONE',  ( -12.00000000000001066, -109.0000000000000142, -155.0000000000000284 ) ) ;
#10084=CARTESIAN_POINT ( 'NONE',  ( -442.0000000000000000, -125.0000000000000000, 194.9999999999999716 ) ) ;
#10095=CARTESIAN_POINT ( 'NONE',  ( -449.9999999999999432, 137.0000000000000000, -175.0000000000000000 ) ) ;
#10099=ORIENTED_EDGE ( 'NONE', *, *, #5359, .F. ) ;
#10104=CARTESIAN_POINT ( 'NONE',  ( -499.9999999999999432, 112.9999999999999574, -194.9999999999999716 ) ) ;
#10105=DIRECTION ( 'NONE',  ( 0.000000000000000000, 0.000000000000000000, -1.000000000000000000 ) ) ;
#10114=LINE ( 'NONE', #2106, #16664 ) ;
#10120=VECTOR ( 'NONE', #17692, 1000.000000000000000 ) ;
#10121=VERTEX_POINT ( 'NONE', #19912 ) ;
#10122=CYLINDRICAL_SURFACE ( 'NONE', #5726, 3.999999999999976019 ) ;
#10126=ORIENTED_EDGE ( 'NONE', *, *, #8259, .F. ) ;
#10127=CIRCLE ( 'NONE', #30023, 4.750000000000004441 ) ;
#10128=ORIENTED_EDGE ( 'NONE', *, *, #20900, .T. ) ;
#10131=ORIENTED_EDGE ( 'NONE', *, *, #9603, .T. ) ;
#10134=LINE ( 'NONE', #12642, #32301 ) ;
#10140=CIRCLE ( 'NONE', #10787, 3.999999999999948042 ) ;
#10143=AXIS2_PLACEMENT_3D ( 'NONE', #15902, #26724, #9828 ) ;
#10149=CARTESIAN_POINT ( 'NONE',  ( -418.0000000000000000, 104.9999999999999858, -162.9999999999999716 ) ) ;
#10156=CARTESIAN_POINT ( 'NONE',  ( -499.9999999999999432, 104.9999999999999858, 162.9999999999999716 ) ) ;
#10159=AXIS2_PLACEMENT_3D ( 'NONE', #7245, #12277, #31291 ) ;
#10162=LINE ( 'NONE', #34019, #25812 ) ;
#10172=MANIFOLD_SOLID_BREP ( 'Boss-Extrude4[2]', #8657 ) ;
#10174=ORIENTED_EDGE ( 'NONE', *, *, #2834, .T. ) ;
#10175=EDGE_CURVE ( 'NONE', #25102, #23404, #20408, .T. ) ;
#10179=VERTEX_POINT ( 'NONE', #25227 ) ;
#10180=ORIENTED_EDGE ( 'NONE', *, *, #15929, .T. ) ;
#10184=VECTOR ( 'NONE', #10942, 1000.000000000000000 ) ;
#10190=EDGE_LOOP ( 'NONE', ( #18358, #7019, #30378, #14147 ) ) ;
#10196=ORIENTED_EDGE ( 'NONE', *, *, #29369, .F. ) ;
#10197=LINE ( 'NONE', #26386, #18058 ) ;
#10199=AXIS2_PLACEMENT_3D ( 'NONE', #22502, #3959, #17358 ) ;
#10200=LINE ( 'NONE', #29765, #27585 ) ;
#10201=FACE_OUTER_BOUND ( 'NONE', #17098, .T. ) ;
#10206=FACE_OUTER_BOUND ( 'NONE', #19535, .T. ) ;
#10207=ORIENTED_EDGE ( 'NONE', *, *, #29532, .F. ) ;
#10211=VECTOR ( 'NONE', #31792, 1000.000000000000000 ) ;
#10212=ORIENTED_EDGE ( 'NONE', *, *, #26086, .T. ) ;
#10213=EDGE_CURVE ( 'NONE', #6336, #24518, #5031, .T. ) ;
#10214=EDGE_CURVE ( 'NONE', #1917, #6409, #512, .T. ) ;
#10216=VERTEX_POINT ( 'NONE', #6358 ) ;
#10217=VECTOR ( 'NONE', #1960, 1000.000000000000000 ) ;
#10221=ORIENTED_EDGE ( 'NONE', *, *, #13190, .T. ) ;
#10222=DIRECTION ( 'NONE',  ( 0.000000000000000000, -2.465190328815661892E-32, -1.000000000000000000 ) ) ;
#10223=ADVANCED_FACE ( 'NONE', ( #1036 ), #20436, .F. ) ;
#10225=PLANE ( 'NONE',  #32448 ) ;
#10231=ADVANCED_FACE ( 'NONE', ( #12781 ), #31796, .T. ) ;
#10234=UNCERTAINTY_MEASURE_WITH_UNIT (LENGTH_MEASURE( 1.000000000000000082E-05 ), #3448, 'distance_accuracy_value', 'NONE');
#10238=ADVANCED_FACE ( 'NONE', ( #12259 ), #17773, .F. ) ;
#10240=ORIENTED_EDGE ( 'NONE', *, *, #10487, .F. ) ;
#10247=ORIENTED_EDGE ( 'NONE', *, *, #7251, .F. ) ;
#10249=ORIENTED_EDGE ( 'NONE', *, *, #6405, .T. ) ;
#10250=DIRECTION ( 'NONE',  ( 0.000000000000000000, -1.000000000000000000, 0.000000000000000000 ) ) ;
#10252=ORIENTED_EDGE ( 'NONE', *, *, #15815, .T. ) ;
#10254=CARTESIAN_POINT ( 'NONE',  ( -430.0000000000000000, 118.9999999999999716, 130.0000000000000000 ) ) ;
#10260=CARTESIAN_POINT ( 'NONE',  ( -410.0000000000000568, 113.0000000000000000, 154.9999999999999716 ) ) ;
#10262=DIRECTION ( 'NONE',  ( 1.000000000000000000, -0.000000000000000000, -0.000000000000000000 ) ) ;
#10264=DIRECTION ( 'NONE',  ( -1.000000000000000000, 0.000000000000000000, 0.000000000000000000 ) ) ;
#10267=EDGE_LOOP ( 'NONE', ( #33817, #23943, #14335, #24138, #13010, #17686 ) ) ;
#10269=VECTOR ( 'NONE', #18458, 1000.000000000000000 ) ;
#10275=EDGE_CURVE ( 'NONE', #11988, #11647, #28613, .T. ) ;
#10276=EDGE_CURVE ( 'NONE', #29324, #19338, #1070, .T. ) ;
#10277=CARTESIAN_POINT ( 'NONE',  ( -430.0000000000000000, -119.0000000000000000, 126.0000000000000000 ) ) ;
#10278=CARTESIAN_POINT ( 'NONE',  ( -418.0000000000000000, 124.9999999999999574, -194.9999999999999716 ) ) ;
#10279=DIRECTION ( 'NONE',  ( 1.000000000000000000, 0.000000000000000000, 5.546364386991661285E-52 ) ) ;
#10280=VERTEX_POINT ( 'NONE', #20951 ) ;
#10282=FACE_OUTER_BOUND ( 'NONE', #30498, .T. ) ;
#10284=CIRCLE ( 'NONE', #23367, 4.000000000000003553 ) ;
#10286=EDGE_LOOP ( 'NONE', ( #12652, #21109, #13555, #534 ) ) ;
#10290=FACE_OUTER_BOUND ( 'NONE', #6928, .T. ) ;
#10294=VECTOR ( 'NONE', #2406, 1000.000000000000000 ) ;
#10295=CARTESIAN_POINT ( 'NONE',  ( -410.0000000000000568, 105.0000000000000142, -175.0000000000000000 ) ) ;
#10297=ORIENTED_EDGE ( 'NONE', *, *, #13498, .T. ) ;
#10298=ORIENTED_EDGE ( 'NONE', *, *, #34751, .F. ) ;
#10300=VECTOR ( 'NONE', #4310, 1000.000000000000000 ) ;
#10301=EDGE_CURVE ( 'NONE', #30602, #18391, #27779, .T. ) ;
#10306=DIRECTION ( 'NONE',  ( 0.000000000000000000, 0.000000000000000000, -1.000000000000000000 ) ) ;
#10307=FACE_BOUND ( 'NONE', #7110, .T. ) ;
#10313=EDGE_CURVE ( 'NONE', #11417, #32678, #33780, .T. ) ;
#10314=EDGE_CURVE ( 'NONE', #18883, #31191, #9742, .T. ) ;
#10315=PLANE ( 'NONE',  #26979 ) ;
#10316=CARTESIAN_POINT ( 'NONE',  ( -499.9999999999999432, 108.9999999999999858, 162.9999999999999716 ) ) ;
#10318=VERTEX_POINT ( 'NONE', #29130 ) ;
#10319=VERTEX_POINT ( 'NONE', #14756 ) ;
#10324=MECHANICAL_DESIGN_GEOMETRIC_PRESENTATION_REPRESENTATION('',(#33623),#10885);
#10327=ORIENTED_EDGE ( 'NONE', *, *, #22490, .F. ) ;
#10328=DIRECTION ( 'NONE',  ( -0.000000000000000000, 0.000000000000000000, 1.000000000000000000 ) ) ;
#10330=VERTEX_POINT ( 'NONE', #22925 ) ;
#10332=( NAMED_UNIT ( * ) PLANE_ANGLE_UNIT ( ) SI_UNIT ( $, .RADIAN. ) );
#10333=CARTESIAN_POINT ( 'NONE',  ( -442.0000000000000000, -104.9999999999999858, -194.9999999999999716 ) ) ;
#10335=LINE ( 'NONE', #13371, #23067 ) ;
#10338=CARTESIAN_POINT ( 'NONE',  ( -12.00000000000001066, -145.0000000000000000, 187.0000000000000000 ) ) ;
#10339=AXIS2_PLACEMENT_3D ( 'NONE', #20806, #15838, #21342 ) ;
#10343=AXIS2_PLACEMENT_3D ( 'NONE', #14951, #9602, #1750 ) ;
#10344=MANIFOLD_SOLID_BREP ( 'Square tube 20 X 20 X 2(1)[4]', #22482 ) ;
#10345=ORIENTED_EDGE ( 'NONE', *, *, #18471, .F. ) ;
#10346=ORIENTED_EDGE ( 'NONE', *, *, #26150, .F. ) ;
#10347=CARTESIAN_POINT ( 'NONE',  ( -12.00000000000001066, -112.9999999999999858, 155.0000000000000000 ) ) ;
#10348=EDGE_CURVE ( 'NONE', #5234, #13672, #4031, .T. ) ;
#10356=CARTESIAN_POINT ( 'NONE',  ( -19.99999999999998934, 136.9999999999999716, 155.0000000000000000 ) ) ;
#10360=DIRECTION ( 'NONE',  ( -1.000000000000000000, 0.000000000000000000, 0.000000000000000000 ) ) ;
#10363=EDGE_CURVE ( 'NONE', #14361, #108, #6197, .T. ) ;
#10366=DIRECTION ( 'NONE',  ( -0.000000000000000000, -1.000000000000000000, -0.000000000000000000 ) ) ;
#10370=VECTOR ( 'NONE', #5413, 1000.000000000000000 ) ;
#10374=DIRECTION ( 'NONE',  ( 0.000000000000000000, 0.000000000000000000, 1.000000000000000000 ) ) ;
#10376=EDGE_CURVE ( 'NONE', #10121, #10892, #5088, .T. ) ;
#10380=CARTESIAN_POINT ( 'NONE',  ( -20.00000000000007461, 136.9999999999999432, -187.0000000000000000 ) ) ;
#10381=EDGE_LOOP ( 'NONE', ( #20423, #24808, #15057, #30265 ) ) ;
#10383=DIRECTION ( 'NONE',  ( 0.000000000000000000, 0.000000000000000000, 1.000000000000000000 ) ) ;
#10384=DIRECTION ( 'NONE',  ( 1.300283923313630633E-47, 0.000000000000000000, 1.000000000000000000 ) ) ;
#10385=ORIENTED_EDGE ( 'NONE', *, *, #29287, .F. ) ;
#10386=( NAMED_UNIT ( * ) SI_UNIT ( $, .STERADIAN. ) SOLID_ANGLE_UNIT ( ) );
#10387=ORIENTED_EDGE ( 'NONE', *, *, #31227, .F. ) ;
#10390=AXIS2_PLACEMENT_3D ( 'NONE', #27579, #24540, #8363 ) ;
#10392=AXIS2_PLACEMENT_3D ( 'NONE', #8800, #19676, #22696 ) ;
#10395=VERTEX_POINT ( 'NONE', #16330 ) ;
#10397=DIRECTION ( 'NONE',  ( 1.000000000000000000, 0.000000000000000000, 0.000000000000000000 ) ) ;
#10399=DIRECTION ( 'NONE',  ( 0.000000000000000000, -1.000000000000000000, -1.224646799147353207E-16 ) ) ;
#10403=CARTESIAN_POINT ( 'NONE',  ( -418.0000000000000000, -105.0000000000000142, 187.0000000000000000 ) ) ;
#10411=EDGE_CURVE ( 'NONE', #8166, #3093, #24470, .T. ) ;
#10416=DIRECTION ( 'NONE',  ( -1.000000000000000000, 0.000000000000000000, 0.000000000000000000 ) ) ;
#10417=DIRECTION ( 'NONE',  ( 0.000000000000000000, -0.000000000000000000, 1.000000000000000000 ) ) ;
#10421=ORIENTED_EDGE ( 'NONE', *, *, #12637, .F. ) ;
#10422=CIRCLE ( 'NONE', #14986, 3.999999999999989786 ) ;
#10425=ORIENTED_EDGE ( 'NONE', *, *, #21600, .T. ) ;
#10428=CARTESIAN_POINT ( 'NONE',  ( -19.99999999999998934, -137.0000000000000000, 155.0000000000000000 ) ) ;
#10429=EDGE_CURVE ( 'NONE', #995, #32238, #8295, .T. ) ;
#10430=VERTEX_POINT ( 'NONE', #19175 ) ;
#10434=EDGE_CURVE ( 'NONE', #2726, #4948, #21304, .T. ) ;
#10438=EDGE_CURVE ( 'NONE', #10763, #24914, #14750, .T. ) ;
#10442=ORIENTED_EDGE ( 'NONE', *, *, #2763, .T. ) ;
#10446=DIRECTION ( 'NONE',  ( -0.000000000000000000, 1.000000000000000000, -0.000000000000000000 ) ) ;
#10451=ORIENTED_EDGE ( 'NONE', *, *, #2612, .T. ) ;
#10455=LINE ( 'NONE', #2781, #17409 ) ;
#10460=FACE_OUTER_BOUND ( 'NONE', #32174, .T. ) ;
#10464=CARTESIAN_POINT ( 'NONE',  ( -430.0000000000000000, -131.0000000000000000, 111.9999999999999858 ) ) ;
#10465=VERTEX_POINT ( 'NONE', #30547 ) ;
#10470=VERTEX_POINT ( 'NONE', #22180 ) ;
#10474=VECTOR ( 'NONE', #33998, 1000.000000000000000 ) ;
#10475=LINE ( 'NONE', #29868, #27395 ) ;
#10477=VERTEX_POINT ( 'NONE', #16097 ) ;
#10480=AXIS2_PLACEMENT_3D ( 'NONE', #4240, #34326, #9947 ) ;
#10483=PLANE ( 'NONE',  #6921 ) ;
#10487=EDGE_CURVE ( 'NONE', #11116, #26377, #30013, .T. ) ;
#10490=ORIENTED_EDGE ( 'NONE', *, *, #8887, .T. ) ;
#10492=EDGE_CURVE ( 'NONE', #26511, #27718, #819, .T. ) ;
#10495=CARTESIAN_POINT ( 'NONE',  ( -20.00000000000004619, -105.0000000000000000, -162.9999999999999716 ) ) ;
#10498=LINE ( 'NONE', #32201, #5557 ) ;
#10499=VECTOR ( 'NONE', #33303, 1000.000000000000000 ) ;
#10503=AXIS2_PLACEMENT_3D ( 'NONE', #3060, #16440, #33138 ) ;
#10505=VERTEX_POINT ( 'NONE', #295 ) ;
#10506=VECTOR ( 'NONE', #12499, 1000.000000000000000 ) ;
#10509=AXIS2_PLACEMENT_3D ( 'NONE', #20090, #30755, #1563 ) ;
#10510=CARTESIAN_POINT ( 'NONE',  ( -355.0000000000000000, 118.9999999999999858, 128.0000000000000000 ) ) ;
#10512=EDGE_LOOP ( 'NONE', ( #13701, #2903, #2173, #6832 ) ) ;
#10515=ORIENTED_EDGE ( 'NONE', *, *, #31143, .F. ) ;
#10516=EDGE_CURVE ( 'NONE', #30837, #31738, #14181, .T. ) ;
#10518=DIRECTION ( 'NONE',  ( 1.000000000000000000, 0.000000000000000000, -1.232595164407831220E-32 ) ) ;
#10519=LINE ( 'NONE', #24379, #20118 ) ;
#10522=VECTOR ( 'NONE', #6049, 1000.000000000000000 ) ;
#10523=LINE ( 'NONE', #1796, #26780 ) ;
#10535=AXIS2_PLACEMENT_3D ( 'NONE', #5679, #27060, #30255 ) ;
#10541=ORIENTED_EDGE ( 'NONE', *, *, #6753, .T. ) ;
#10542=DIRECTION ( 'NONE',  ( 0.000000000000000000, -5.145227585319922065E-49, -1.000000000000000000 ) ) ;
#10548=ORIENTED_EDGE ( 'NONE', *, *, #23072, .T. ) ;
#10549=LINE ( 'NONE', #15907, #12332 ) ;
#10554=DIRECTION ( 'NONE',  ( -1.000000000000000000, 0.000000000000000000, 0.000000000000000000 ) ) ;
#10558=DIRECTION ( 'NONE',  ( -1.000000000000000000, 0.000000000000000000, -1.300283923313630633E-47 ) ) ;
#10562=DIRECTION ( 'NONE',  ( -1.000000000000000000, 0.000000000000000000, -1.300283923313630633E-47 ) ) ;
#10565=CARTESIAN_POINT ( 'NONE',  ( -12.00000000000001066, -56.99999999999997868, 154.9999999999999716 ) ) ;
#10566=EDGE_CURVE ( 'NONE', #20271, #1001, #25366, .T. ) ;
#10567=CARTESIAN_POINT ( 'NONE',  ( 11.99999999999999645, -124.9999999999999432, -154.9999999999999716 ) ) ;
#10571=FACE_OUTER_BOUND ( 'NONE', #13045, .T. ) ;
#10573=CIRCLE ( 'NONE', #13442, 7.999999999999979572 ) ;
#10574=EDGE_CURVE ( 'NONE', #28861, #11080, #24655, .T. ) ;
#10577=EDGE_CURVE ( 'NONE', #31670, #17427, #11331, .T. ) ;
#10578=VECTOR ( 'NONE', #2566, 1000.000000000000000 ) ;
#10582=DIRECTION ( 'NONE',  ( 0.000000000000000000, -1.000000000000000000, 2.309213040847544338E-50 ) ) ;
#10583=ORIENTED_EDGE ( 'NONE', *, *, #4996, .F. ) ;
#10587=EDGE_CURVE ( 'NONE', #26714, #28665, #30359, .T. ) ;
#10588=CIRCLE ( 'NONE', #23098, 7.999999999999979572 ) ;
#10589=LINE ( 'NONE', #18430, #30562 ) ;
#10591=ORIENTED_EDGE ( 'NONE', *, *, #12397, .T. ) ;
#10592=ORIENTED_EDGE ( 'NONE', *, *, #7525, .T. ) ;
#10593=LINE ( 'NONE', #26772, #5441 ) ;
#10598=VECTOR ( 'NONE', #18912, 1000.000000000000000 ) ;
#10599=CARTESIAN_POINT ( 'NONE',  ( -15.99999999999998579, -145.0000000000000000, 162.9999999999999716 ) ) ;
#10600=LINE ( 'NONE', #11127, #10184 ) ;
#10602=VECTOR ( 'NONE', #26655, 1000.000000000000000 ) ;
#10604=CARTESIAN_POINT ( 'NONE',  ( -365.0000000000000000, -131.0000000000000000, 111.9999999999999858 ) ) ;
#10605=DIRECTION ( 'NONE',  ( 0.000000000000000000, -1.000000000000000000, 1.310824597558155437E-49 ) ) ;
#10609=DIRECTION ( 'NONE',  ( 0.000000000000000000, 0.000000000000000000, -1.000000000000000000 ) ) ;
#10615=ORIENTED_EDGE ( 'NONE', *, *, #20893, .F. ) ;
#10621=CIRCLE ( 'NONE', #26536, 7.999999999999979572 ) ;
#10622=EDGE_CURVE ( 'NONE', #5027, #7621, #34929, .T. ) ;
#10625=ORIENTED_EDGE ( 'NONE', *, *, #22105, .F. ) ;
#10631=ORIENTED_EDGE ( 'NONE', *, *, #33632, .T. ) ;
#10633=EDGE_LOOP ( 'NONE', ( #7263, #28083, #29714, #12485 ) ) ;
#10641=DIRECTION ( 'NONE',  ( 0.000000000000000000, 0.000000000000000000, 1.000000000000000000 ) ) ;
#10642=ORIENTED_EDGE ( 'NONE', *, *, #19538, .F. ) ;
#10645=CARTESIAN_POINT ( 'NONE',  ( -442.0000000000000000, 145.0000000000000000, -175.0000000000000000 ) ) ;
#10650=EDGE_CURVE ( 'NONE', #980, #7256, #32909, .T. ) ;
#10654=DIRECTION ( 'NONE',  ( 1.000000000000000000, 0.000000000000000000, 0.000000000000000000 ) ) ;
#10655=VECTOR ( 'NONE', #24845, 1000.000000000000000 ) ;
#10657=CARTESIAN_POINT ( 'NONE',  ( -418.0000000000000000, 105.0000000000000000, 135.9999999999999716 ) ) ;
#10658=CIRCLE ( 'NONE', #30554, 7.999999999999979572 ) ;
#10666=ADVANCED_FACE ( 'NONE', ( #12041, #6839 ), #22888, .T. ) ;
#10670=ORIENTED_EDGE ( 'NONE', *, *, #26217, .T. ) ;
#10673=AXIS2_PLACEMENT_3D ( 'NONE', #8486, #13652, #33030 ) ;
#10674=CIRCLE ( 'NONE', #27144, 4.750000000000004441 ) ;
#10675=CARTESIAN_POINT ( 'NONE',  ( 19.99999999999998224, 144.9999999999999147, 187.0000000000000000 ) ) ;
#10680=AXIS2_PLACEMENT_3D ( 'NONE', #12181, #9498, #25506 ) ;
#10683=ORIENTED_EDGE ( 'NONE', *, *, #9414, .T. ) ;
#10684=ORIENTED_EDGE ( 'NONE', *, *, #25499, .F. ) ;
#10692=ORIENTED_EDGE ( 'NONE', *, *, #13140, .F. ) ;
#10695=CIRCLE ( 'NONE', #8983, 4.750000000000004441 ) ;
#10696=DIRECTION ( 'NONE',  ( 0.000000000000000000, -0.000000000000000000, -1.000000000000000000 ) ) ;
#10699=DIRECTION ( 'NONE',  ( 0.000000000000000000, 0.000000000000000000, -1.000000000000000000 ) ) ;
#10703=AXIS2_PLACEMENT_3D ( 'NONE', #19103, #32596, #12885 ) ;
#10705=LINE ( 'NONE', #27235, #13726 ) ;
#10707=LINE ( 'NONE', #18557, #19508 ) ;
#10719=DIRECTION ( 'NONE',  ( 0.000000000000000000, 1.000000000000000000, -3.374343856708137958E-53 ) ) ;
#10720=DIRECTION ( 'NONE',  ( 1.000000000000000000, 3.469446951953834515E-18, 0.000000000000000000 ) ) ;
#10721=VECTOR ( 'NONE', #728, 1000.000000000000000 ) ;
#10726=FACE_OUTER_BOUND ( 'NONE', #31814, .T. ) ;
#10730=CARTESIAN_POINT ( 'NONE',  ( -19.99999999999998934, 134.9999999999998863, 162.9999999999999716 ) ) ;
#10732=ORIENTED_EDGE ( 'NONE', *, *, #13663, .F. ) ;
#10733=CIRCLE ( 'NONE', #1047, 7.999999999999979572 ) ;
#10734=EDGE_CURVE ( 'NONE', #8663, #28119, #28576, .T. ) ;
#10737=EDGE_CURVE ( 'NONE', #10179, #23824, #31223, .T. ) ;
#10738=LINE ( 'NONE', #219, #31686 ) ;
#10742=DIRECTION ( 'NONE',  ( 1.000000000000000000, 0.000000000000000000, 0.000000000000000000 ) ) ;
#10747=DIRECTION ( 'NONE',  ( 0.000000000000000000, 0.000000000000000000, -1.000000000000000000 ) ) ;
#10753=VERTEX_POINT ( 'NONE', #388 ) ;
#10757=VERTEX_POINT ( 'NONE', #32582 ) ;
#10760=AXIS2_PLACEMENT_3D ( 'NONE', #7150, #4478, #15370 ) ;
#10762=FACE_OUTER_BOUND ( 'NONE', #30248, .T. ) ;
#10763=VERTEX_POINT ( 'NONE', #16243 ) ;
#10767=MANIFOLD_SOLID_BREP ( 'Square tube 40 X 40 X 4(1)[13]', #18508 ) ;
#10768=EDGE_CURVE ( 'NONE', #34323, #27344, #29930, .T. ) ;
#10769=CARTESIAN_POINT ( 'NONE',  ( 11.99999999999995559, -145.0000000000000000, -186.9999999999999716 ) ) ;
#10770=DIRECTION ( 'NONE',  ( 0.000000000000000000, 0.000000000000000000, 1.000000000000000000 ) ) ;
#10772=VECTOR ( 'NONE', #35014, 1000.000000000000000 ) ;
#10776=VERTEX_POINT ( 'NONE', #5871 ) ;
#10777=CARTESIAN_POINT ( 'NONE',  ( -499.9999999999999432, 140.9999999999999716, 187.0000000000000000 ) ) ;
#10779=DIRECTION ( 'NONE',  ( 0.000000000000000000, -2.465190328815661892E-32, -1.000000000000000000 ) ) ;
#10784=DIRECTION ( 'NONE',  ( 1.232595164407831220E-32, -3.421138828918010427E-49, 1.000000000000000000 ) ) ;
#10786=CARTESIAN_POINT ( 'NONE',  ( -12.00000000000001066, 112.9999999999999574, -175.0000000000000284 ) ) ;
#10787=AXIS2_PLACEMENT_3D ( 'NONE', #27964, #28494, #1092 ) ;
#10792=EDGE_LOOP ( 'NONE', ( #29215, #838, #13837, #20229 ) ) ;
#10796=ORIENTED_EDGE ( 'NONE', *, *, #2836, .F. ) ;
#10797=EDGE_LOOP ( 'NONE', ( #5626, #14014, #22770, #21941 ) ) ;
#10799=AXIS2_PLACEMENT_3D ( 'NONE', #15200, #26044, #22857 ) ;
#10800=DIRECTION ( 'NONE',  ( 1.000000000000000000, 0.000000000000000000, 1.300283923313630633E-47 ) ) ;
#10804=ORIENTED_EDGE ( 'NONE', *, *, #3696, .T. ) ;
#10810=CARTESIAN_POINT ( 'NONE',  ( -442.0000000000000000, -105.0000000000000142, -174.9999999999999716 ) ) ;
#10811=CARTESIAN_POINT ( 'NONE',  ( -11.99999999999998224, -134.9999999999999716, 155.0000000000000000 ) ) ;
#10817=DIRECTION ( 'NONE',  ( -1.000000000000000000, 0.000000000000000000, 0.000000000000000000 ) ) ;
#10819=ORIENTED_EDGE ( 'NONE', *, *, #6018, .F. ) ;
#10820=ADVANCED_FACE ( 'NONE', ( #3037 ), #24753, .T. ) ;
#10821=DIRECTION ( 'NONE',  ( 0.000000000000000000, 0.000000000000000000, -1.000000000000000000 ) ) ;
#10828=VERTEX_POINT ( 'NONE', #17650 ) ;
#10829=DIRECTION ( 'NONE',  ( 0.000000000000000000, 1.000000000000000000, 1.224646799147353207E-16 ) ) ;
#10836=LINE ( 'NONE', #8333, #31473 ) ;
#10839=CARTESIAN_POINT ( 'NONE',  ( -19.99999999999998934, 4.559999999999908127, -172.9900000000000091 ) ) ;
#10842=ORIENTED_EDGE ( 'NONE', *, *, #34927, .T. ) ;
#10844=CARTESIAN_POINT ( 'NONE',  ( -20.00000000000004619, -137.0000000000000000, -162.9999999999999716 ) ) ;
#10851=VERTEX_POINT ( 'NONE', #17121 ) ;
#10852=DIRECTION ( 'NONE',  ( 1.000000000000000000, 0.000000000000000000, 5.546364386991661285E-52 ) ) ;
#10856=ORIENTED_EDGE ( 'NONE', *, *, #14589, .T. ) ;
#10857=CYLINDRICAL_SURFACE ( 'NONE', #28869, 4.000000000000003553 ) ;
#10858=VECTOR ( 'NONE', #21743, 1000.000000000000000 ) ;
#10860=ADVANCED_FACE ( 'NONE', ( #17821 ), #23839, .T. ) ;
#10863=ORIENTED_EDGE ( 'NONE', *, *, #11618, .T. ) ;
#10864=DIRECTION ( 'NONE',  ( 0.000000000000000000, 1.000000000000000000, -3.374343856708137958E-53 ) ) ;
#10869=CARTESIAN_POINT ( 'NONE',  ( -20.00000000000007461, 112.9999999999999574, 162.9999999999999716 ) ) ;
#10870=AXIS2_PLACEMENT_3D ( 'NONE', #4834, #29051, #31551 ) ;
#10872=AXIS2_PLACEMENT_3D ( 'NONE', #11289, #3607, #957 ) ;
#10874=CARTESIAN_POINT ( 'NONE',  ( -345.0000000000000000, 124.9999999999999432, 181.0000000000000000 ) ) ;
#10875=ORIENTED_EDGE ( 'NONE', *, *, #28074, .T. ) ;
#10885=( GEOMETRIC_REPRESENTATION_CONTEXT ( 3 ) GLOBAL_UNCERTAINTY_ASSIGNED_CONTEXT ( ( #25307 ) ) GLOBAL_UNIT_ASSIGNED_CONTEXT ( ( #22116, #221, #8406 ) ) REPRESENTATION_CONTEXT ( 'NONE', 'WORKASPACE' ) );
#10886=CARTESIAN_POINT ( 'NONE',  ( -499.9999999999999432, 144.9999999999999716, 162.9999999999999716 ) ) ;
#10892=VERTEX_POINT ( 'NONE', #23665 ) ;
#10894=CARTESIAN_POINT ( 'NONE',  ( -442.0000000000000000, -105.0000000000000142, -155.0000000000000000 ) ) ;
#10896=FACE_OUTER_BOUND ( 'NONE', #5930, .T. ) ;
#10898=ORIENTED_EDGE ( 'NONE', *, *, #27509, .T. ) ;
#10900=LINE ( 'NONE', #5015, #15197 ) ;
#10902=CARTESIAN_POINT ( 'NONE',  ( -365.0000000000000000, -131.0000000000000000, 128.0000000000000000 ) ) ;
#10916=CIRCLE ( 'NONE', #28548, 7.999999999999979572 ) ;
#10917=DIRECTION ( 'NONE',  ( 0.000000000000000000, 0.000000000000000000, -1.000000000000000000 ) ) ;
#10919=ORIENTED_EDGE ( 'NONE', *, *, #17828, .F. ) ;
#10920=LINE ( 'NONE', #32270, #4651 ) ;
#10925=DIRECTION ( 'NONE',  ( 0.000000000000000000, 0.000000000000000000, -1.000000000000000000 ) ) ;
#10927=ORIENTED_EDGE ( 'NONE', *, *, #4080, .F. ) ;
#10932=DIRECTION ( 'NONE',  ( -0.000000000000000000, 1.000000000000000000, -0.000000000000000000 ) ) ;
#10934=VERTEX_POINT ( 'NONE', #23484 ) ;
#10940=ORIENTED_EDGE ( 'NONE', *, *, #7525, .F. ) ;
#10941=CARTESIAN_POINT ( 'NONE',  ( 15.99999999999998579, 75.55999999999990280, 168.2400000000000091 ) ) ;
#10942=DIRECTION ( 'NONE',  ( 0.000000000000000000, 1.224646799147353207E-16, -1.000000000000000000 ) ) ;
#10948=CARTESIAN_POINT ( 'NONE',  ( -418.0000000000000000, 113.0000000000000000, -155.0000000000000000 ) ) ;
#10949=DIRECTION ( 'NONE',  ( 1.000000000000000000, 0.000000000000000000, 0.000000000000000000 ) ) ;
#10950=VERTEX_POINT ( 'NONE', #9788 ) ;
#10956=ORIENTED_EDGE ( 'NONE', *, *, #34880, .T. ) ;
#10958=VECTOR ( 'NONE', #2621, 1000.000000000000000 ) ;
#10961=EDGE_CURVE ( 'NONE', #1683, #19066, #20651, .T. ) ;
#10965=VERTEX_POINT ( 'NONE', #31665 ) ;
#10966=CARTESIAN_POINT ( 'NONE',  ( -365.0000000000000000, -131.0000000000000000, 126.0000000000000000 ) ) ;
#10973=ORIENTED_EDGE ( 'NONE', *, *, #26225, .F. ) ;
#10976=DIRECTION ( 'NONE',  ( -1.000000000000000000, 0.000000000000000000, 0.000000000000000000 ) ) ;
#10980=DIRECTION ( 'NONE',  ( 1.000000000000000000, 0.000000000000000000, 0.000000000000000000 ) ) ;
#10981=VECTOR ( 'NONE', #25386, 1000.000000000000000 ) ;
#10983=PLANE ( 'NONE',  #10673 ) ;
#10984=VECTOR ( 'NONE', #407, 1000.000000000000000 ) ;
#10988=DIRECTION ( 'NONE',  ( 0.000000000000000000, 0.000000000000000000, 1.000000000000000000 ) ) ;
#10989=FACE_OUTER_BOUND ( 'NONE', #1189, .T. ) ;
#10990=EDGE_LOOP ( 'NONE', ( #33255, #32663, #14198, #11508 ) ) ;
#10992=ORIENTED_EDGE ( 'NONE', *, *, #6102, .F. ) ;
#10994=DIRECTION ( 'NONE',  ( 1.000000000000000000, 3.469446951953834515E-18, 0.000000000000000000 ) ) ;
#10995=VECTOR ( 'NONE', #42, 1000.000000000000000 ) ;
#10996=ORIENTED_EDGE ( 'NONE', *, *, #1707, .F. ) ;
#10998=DIRECTION ( 'NONE',  ( -0.000000000000000000, 1.000000000000000000, -0.000000000000000000 ) ) ;
#11000=CARTESIAN_POINT ( 'NONE',  ( -355.0000000000000000, -133.0000000000000000, 113.9999999999999858 ) ) ;
#11001=EDGE_CURVE ( 'NONE', #28629, #10047, #2126, .T. ) ;
#11002=ORIENTED_EDGE ( 'NONE', *, *, #7283, .T. ) ;
#11004=EDGE_CURVE ( 'NONE', #28476, #2088, #3869, .T. ) ;
#11006=VECTOR ( 'NONE', #3452, 1000.000000000000000 ) ;
#11012=CARTESIAN_POINT ( 'NONE',  ( -414.0000000000000568, -105.0000000000000142, 132.0000000000000000 ) ) ;
#11014=CARTESIAN_POINT ( 'NONE',  ( -20.00000000000001776, -113.0000000000000000, 190.9999999999999716 ) ) ;
#11020=CARTESIAN_POINT ( 'NONE',  ( -20.00000000000007461, 136.9999999999999432, -155.0000000000000000 ) ) ;
#11021=ADVANCED_FACE ( 'NONE', ( #21691 ), #16023, .T. ) ;
#11022=CARTESIAN_POINT ( 'NONE',  ( -499.9999999999999432, 136.9999999999999432, -159.0000000000000000 ) ) ;
#11026=DIRECTION ( 'NONE',  ( 1.000000000000000000, 0.000000000000000000, 0.000000000000000000 ) ) ;
#11029=DIRECTION ( 'NONE',  ( 0.000000000000000000, 0.000000000000000000, 1.000000000000000000 ) ) ;
#11031=ORIENTED_EDGE ( 'NONE', *, *, #34846, .F. ) ;
#11033=ORIENTED_EDGE ( 'NONE', *, *, #6126, .T. ) ;
#11037=CARTESIAN_POINT ( 'NONE',  ( -430.0000000000000000, -135.0000000000000000, 126.0000000000000000 ) ) ;
#11038=ORIENTED_EDGE ( 'NONE', *, *, #30180, .T. ) ;
#11047=CARTESIAN_POINT ( 'NONE',  ( 15.99999999999997868, -137.0000000000000000, -155.0000000000000284 ) ) ;
#11052=DIRECTION ( 'NONE',  ( 0.000000000000000000, -1.000000000000000000, -5.145227585319922065E-49 ) ) ;
#11055=EDGE_CURVE ( 'NONE', #143, #28422, #11282, .T. ) ;
#11059=EDGE_CURVE ( 'NONE', #9649, #29470, #13170, .T. ) ;
#11060=DIRECTION ( 'NONE',  ( 1.000000000000000000, -2.530127506375325948E-80, 1.848892746611746419E-32 ) ) ;
#11061=VECTOR ( 'NONE', #18022, 1000.000000000000000 ) ;
#11062=EDGE_CURVE ( 'NONE', #1917, #1130, #13688, .T. ) ;
#11065=PRODUCT_CONTEXT ( 'NONE', #27351, 'mechanical' ) ;
#11066=VERTEX_POINT ( 'NONE', #29711 ) ;
#11067=LINE ( 'NONE', #32407, #7656 ) ;
#11069=VECTOR ( 'NONE', #14757, 1000.000000000000000 ) ;
#11072=ORIENTED_EDGE ( 'NONE', *, *, #9911, .T. ) ;
#11075=LINE ( 'NONE', #25596, #6724 ) ;
#11080=VERTEX_POINT ( 'NONE', #30228 ) ;
#11085=VECTOR ( 'NONE', #7069, 1000.000000000000000 ) ;
#11087=ORIENTED_EDGE ( 'NONE', *, *, #16761, .T. ) ;
#11094=CARTESIAN_POINT ( 'NONE',  ( -449.9999999999999432, 105.0000000000000142, -175.0000000000000000 ) ) ;
#11097=CARTESIAN_POINT ( 'NONE',  ( -499.9999999999999432, 112.9999999999999574, 187.0000000000000000 ) ) ;
#11098=CARTESIAN_POINT ( 'NONE',  ( -499.9999999999999432, 104.9999999999999858, -162.9999999999999716 ) ) ;
#11103=ADVANCED_FACE ( 'NONE', ( #24707 ), #16551, .T. ) ;
#11104=EDGE_CURVE ( 'NONE', #11445, #24518, #10498, .T. ) ;
#11109=ORIENTED_EDGE ( 'NONE', *, *, #19560, .T. ) ;
#11112=EDGE_CURVE ( 'NONE', #1812, #22871, #19223, .T. ) ;
#11114=DIRECTION ( 'NONE',  ( 1.000000000000000000, 0.000000000000000000, 0.000000000000000000 ) ) ;
#11115=DIRECTION ( 'NONE',  ( -0.000000000000000000, -5.145227585319922065E-49, -1.000000000000000000 ) ) ;
#11116=VERTEX_POINT ( 'NONE', #30066 ) ;
#11118=VECTOR ( 'NONE', #29123, 1000.000000000000000 ) ;
#11119=CARTESIAN_POINT ( 'NONE',  ( -418.0000000000000000, 105.0000000000000142, -175.0000000000000000 ) ) ;
#11124=CARTESIAN_POINT ( 'NONE',  ( -414.0000000000000568, -125.0000000000000000, -101.9999999999999858 ) ) ;
#11125=ORIENTED_EDGE ( 'NONE', *, *, #34428, .T. ) ;
#11127=CARTESIAN_POINT ( 'NONE',  ( 15.99999999999998579, 144.9999999999999716, -186.9999999999999432 ) ) ;
#11130=LINE ( 'NONE', #21981, #10370 ) ;
#11133=ADVANCED_FACE ( 'NONE', ( #15854 ), #26685, .F. ) ;
#11134=DIRECTION ( 'NONE',  ( -0.000000000000000000, 0.000000000000000000, 1.000000000000000000 ) ) ;
#11137=AXIS2_PLACEMENT_3D ( 'NONE', #24662, #300, #27866 ) ;
#11138=CARTESIAN_POINT ( 'NONE',  ( -70.00000000000000000, 4.559999999999908127, -172.9900000000000091 ) ) ;
#11139=ORIENTED_EDGE ( 'NONE', *, *, #20900, .F. ) ;
#11141=VECTOR ( 'NONE', #8790, 1000.000000000000000 ) ;
#11142=CARTESIAN_POINT ( 'NONE',  ( -445.9999999999999432, -124.9999999999999858, -77.99999999999997158 ) ) ;
#11147=EDGE_CURVE ( 'NONE', #15752, #30776, #14587, .T. ) ;
#11149=VECTOR ( 'NONE', #31685, 1000.000000000000000 ) ;
#11151=ORIENTED_EDGE ( 'NONE', *, *, #18219, .F. ) ;
#11152=EDGE_LOOP ( 'NONE', ( #20593, #20199, #14494, #15189 ) ) ;
#11153=DIRECTION ( 'NONE',  ( 1.000000000000000000, 0.000000000000000000, 0.000000000000000000 ) ) ;
#11155=ORIENTED_EDGE ( 'NONE', *, *, #19808, .F. ) ;
#11161=CARTESIAN_POINT ( 'NONE',  ( 12.00000000000004086, -60.99999999999996447, 155.0000000000000284 ) ) ;
#11162=ORIENTED_EDGE ( 'NONE', *, *, #22794, .T. ) ;
#11163=VERTEX_POINT ( 'NONE', #3871 ) ;
#11170=DIRECTION ( 'NONE',  ( 1.000000000000000000, -0.000000000000000000, -0.000000000000000000 ) ) ;
#11173=DIRECTION ( 'NONE',  ( 0.000000000000000000, 0.000000000000000000, 1.000000000000000000 ) ) ;
#11174=EDGE_CURVE ( 'NONE', #30882, #30602, #19743, .T. ) ;
#11176=ORIENTED_EDGE ( 'NONE', *, *, #2678, .T. ) ;
#11180=MANIFOLD_SOLID_BREP ( 'Trim/Extend7[1]', #14934 ) ;
#11184=VERTEX_POINT ( 'NONE', #17081 ) ;
#11186=DIRECTION ( 'NONE',  ( 0.000000000000000000, 1.000000000000000000, 1.224646799147353207E-16 ) ) ;
#11191=ORIENTED_EDGE ( 'NONE', *, *, #25667, .T. ) ;
#11194=ORIENTED_EDGE ( 'NONE', *, *, #6463, .T. ) ;
#11196=DIRECTION ( 'NONE',  ( -1.000000000000000000, 0.000000000000000000, 0.000000000000000000 ) ) ;
#11201=VERTEX_POINT ( 'NONE', #19567 ) ;
#11203=DIRECTION ( 'NONE',  ( -0.000000000000000000, -0.000000000000000000, -1.000000000000000000 ) ) ;
#11204=CIRCLE ( 'NONE', #28801, 3.999999999999976019 ) ;
#11208=EDGE_LOOP ( 'NONE', ( #24507, #14827, #22333, #28618, #9541, #24273, #13638, #8647 ) ) ;
#11210=LINE ( 'NONE', #29716, #33353 ) ;
#11214=DIRECTION ( 'NONE',  ( -1.292961597001347186E-16, 0.000000000000000000, 1.000000000000000000 ) ) ;
#11217=FACE_OUTER_BOUND ( 'NONE', #31655, .T. ) ;
#11220=DIRECTION ( 'NONE',  ( 0.000000000000000000, 1.000000000000000000, -3.374343856708137958E-53 ) ) ;
#11222=EDGE_CURVE ( 'NONE', #14883, #25692, #22584, .T. ) ;
#11223=CARTESIAN_POINT ( 'NONE',  ( -365.0000000000000000, -125.0000000000000284, 168.9999999999999716 ) ) ;
#11229=VECTOR ( 'NONE', #32861, 1000.000000000000000 ) ;
#11231=ORIENTED_EDGE ( 'NONE', *, *, #28216, .T. ) ;
#11234=MANIFOLD_SOLID_BREP ( 'Trim/Extend4[2]', #27017 ) ;
#11236=VERTEX_POINT ( 'NONE', #1569 ) ;
#11239=VERTEX_POINT ( 'NONE', #34126 ) ;
#11240=DIRECTION ( 'NONE',  ( 0.000000000000000000, -1.000000000000000000, 6.123233995736766036E-17 ) ) ;
#11243=CARTESIAN_POINT ( 'NONE',  ( -414.0000000000000568, 137.0000000000000000, -175.0000000000000000 ) ) ;
#11246=VERTEX_POINT ( 'NONE', #31802 ) ;
#11247=VERTEX_POINT ( 'NONE', #12442 ) ;
#11253=CARTESIAN_POINT ( 'NONE',  ( 11.99999999999999645, 144.9999999999999716, 194.9999999999999716 ) ) ;
#11254=ORIENTED_EDGE ( 'NONE', *, *, #23305, .F. ) ;
#11258=DIRECTION ( 'NONE',  ( 1.000000000000000000, 0.000000000000000000, 0.000000000000000000 ) ) ;
#11259=CYLINDRICAL_SURFACE ( 'NONE', #4396, 4.750000000000004441 ) ;
#11261=ORIENTED_EDGE ( 'NONE', *, *, #33237, .F. ) ;
#11263=DIRECTION ( 'NONE',  ( 0.000000000000000000, 2.309213040847544338E-50, 1.000000000000000000 ) ) ;
#11264=DIRECTION ( 'NONE',  ( -1.292961597001347186E-16, -0.000000000000000000, 1.000000000000000000 ) ) ;
#11266=CARTESIAN_POINT ( 'NONE',  ( -442.0000000000000000, -145.0000000000000000, 154.9999999999999716 ) ) ;
#11276=ADVANCED_FACE ( 'NONE', ( #12788 ), #20611, .F. ) ;
#11280=ORIENTED_EDGE ( 'NONE', *, *, #11720, .T. ) ;
#11281=VECTOR ( 'NONE', #30267, 1000.000000000000000 ) ;
#11282=CIRCLE ( 'NONE', #24831, 7.999999999999979572 ) ;
#11284=LINE ( 'NONE', #19469, #1958 ) ;
#11286=ORIENTED_EDGE ( 'NONE', *, *, #31026, .F. ) ;
#11289=CARTESIAN_POINT ( 'NONE',  ( -19.99999999999998934, -124.9999999999999432, -162.9999999999999432 ) ) ;
#11292=CARTESIAN_POINT ( 'NONE',  ( -12.00000000000001243, 144.9999999999999147, 194.9999999999999716 ) ) ;
#11293=CARTESIAN_POINT ( 'NONE',  ( -442.0000000000000000, 124.9999999999999574, -190.9999999999999716 ) ) ;
#11295=AXIS2_PLACEMENT_3D ( 'NONE', #26868, #16736, #24892 ) ;
#11297=EDGE_LOOP ( 'NONE', ( #5879, #31104, #21036, #8422 ) ) ;
#11300=CARTESIAN_POINT ( 'NONE',  ( -441.9999999999999432, -141.0000000000000000, -155.0000000000000000 ) ) ;
#11304=DIRECTION ( 'NONE',  ( -1.000000000000000000, 0.000000000000000000, 0.000000000000000000 ) ) ;
#11305=EDGE_CURVE ( 'NONE', #34152, #20441, #7411, .T. ) ;
#11310=EDGE_CURVE ( 'NONE', #27322, #32813, #29426, .T. ) ;
#11312=ORIENTED_EDGE ( 'NONE', *, *, #11551, .F. ) ;
#11313=DIRECTION ( 'NONE',  ( -0.000000000000000000, 1.000000000000000000, -0.000000000000000000 ) ) ;
#11317=CARTESIAN_POINT ( 'NONE',  ( -355.0000000000000000, 116.9999999999999858, 126.0000000000000000 ) ) ;
#11318=DIRECTION ( 'NONE',  ( -0.000000000000000000, -0.000000000000000000, -1.000000000000000000 ) ) ;
#11320=ADVANCED_FACE ( 'NONE', ( #23288 ), #23632, .T. ) ;
#11322=VECTOR ( 'NONE', #28051, 1000.000000000000000 ) ;
#11324=DIRECTION ( 'NONE',  ( 0.000000000000000000, 0.000000000000000000, -1.000000000000000000 ) ) ;
#11325=CARTESIAN_POINT ( 'NONE',  ( -442.0000000000000000, -105.0000000000000142, 155.0000000000000568 ) ) ;
#11326=ORIENTED_EDGE ( 'NONE', *, *, #33540, .F. ) ;
#11331=LINE ( 'NONE', #33013, #24391 ) ;
#11333=EDGE_CURVE ( 'NONE', #24957, #29500, #12268, .T. ) ;
#11338=CARTESIAN_POINT ( 'NONE',  ( -418.0000000000000000, -125.0000000000000000, 162.9999999999999716 ) ) ;
#11339=DIRECTION ( 'NONE',  ( 1.000000000000000000, 0.000000000000000000, 0.000000000000000000 ) ) ;
#11341=EDGE_CURVE ( 'NONE', #18446, #29137, #4039, .T. ) ;
#11343=AXIS2_PLACEMENT_3D ( 'NONE', #14197, #25020, #18266 ) ;
#11347=ORIENTED_EDGE ( 'NONE', *, *, #14332, .T. ) ;
#11354=DIRECTION ( 'NONE',  ( 1.000000000000000000, 0.000000000000000000, 0.000000000000000000 ) ) ;
#11355=ORIENTED_EDGE ( 'NONE', *, *, #21891, .T. ) ;
#11356=DIRECTION ( 'NONE',  ( 1.000000000000000000, 0.000000000000000000, -1.848892746611746966E-32 ) ) ;
#11357=FACE_OUTER_BOUND ( 'NONE', #5198, .T. ) ;
#11359=FACE_OUTER_BOUND ( 'NONE', #29395, .T. ) ;
#11361=CARTESIAN_POINT ( 'NONE',  ( -445.9999999999999432, -125.0000000000000000, -101.9999999999999858 ) ) ;
#11362=ORIENTED_EDGE ( 'NONE', *, *, #33677, .F. ) ;
#11365=VERTEX_POINT ( 'NONE', #27000 ) ;
#11366=CARTESIAN_POINT ( 'NONE',  ( -12.00000000000001066, 144.9999999999999716, -158.9999999999999716 ) ) ;
#11368=DIRECTION ( 'NONE',  ( 1.000000000000000000, 0.000000000000000000, 0.000000000000000000 ) ) ;
#11374=VERTEX_POINT ( 'NONE', #29326 ) ;
#11375=CARTESIAN_POINT ( 'NONE',  ( -418.0000000000000000, -125.0000000000000000, 104.0000000000000142 ) ) ;
#11376=LINE ( 'NONE', #11739, #18496 ) ;
#11377=VERTEX_POINT ( 'NONE', #29503 ) ;
#11378=EDGE_LOOP ( 'NONE', ( #15436, #15630, #12576, #2468 ) ) ;
#11382=DIRECTION ( 'NONE',  ( 1.000000000000000000, 0.000000000000000000, -1.232595164407831220E-32 ) ) ;
#11383=ORIENTED_EDGE ( 'NONE', *, *, #19313, .F. ) ;
#11386=FACE_OUTER_BOUND ( 'NONE', #5957, .T. ) ;
#11388=ORIENTED_EDGE ( 'NONE', *, *, #23713, .T. ) ;
#11391=FACE_BOUND ( 'NONE', #18102, .T. ) ;
#11398=VECTOR ( 'NONE', #17747, 1000.000000000000000 ) ;
#11400=ORIENTED_EDGE ( 'NONE', *, *, #2678, .F. ) ;
#11401=EDGE_CURVE ( 'NONE', #25432, #15904, #24664, .T. ) ;
#11417=VERTEX_POINT ( 'NONE', #19005 ) ;
#11419=MECHANICAL_DESIGN_GEOMETRIC_PRESENTATION_REPRESENTATION('',(#31848),#8002);
#11426=CYLINDRICAL_SURFACE ( 'NONE', #20847, 2.000000000000001776 ) ;
#11434=DIRECTION ( 'NONE',  ( 0.000000000000000000, -2.309213040847544338E-50, -1.000000000000000000 ) ) ;
#11436=ORIENTED_EDGE ( 'NONE', *, *, #5430, .F. ) ;
#11440=AXIS2_PLACEMENT_3D ( 'NONE', #32377, #34709, #21182 ) ;
#11441=VECTOR ( 'NONE', #21895, 1000.000000000000000 ) ;
#11444=AXIS2_PLACEMENT_3D ( 'NONE', #13890, #24727, #16041 ) ;
#11445=VERTEX_POINT ( 'NONE', #302 ) ;
#11450=ORIENTED_EDGE ( 'NONE', *, *, #28068, .T. ) ;
#11455=ORIENTED_EDGE ( 'NONE', *, *, #25628, .T. ) ;
#11457=CARTESIAN_POINT ( 'NONE',  ( -12.00000000000001066, 124.9999999999999716, 155.0000000000000000 ) ) ;
#11458=ORIENTED_EDGE ( 'NONE', *, *, #18020, .F. ) ;
#11459=EDGE_CURVE ( 'NONE', #11377, #25387, #7770, .T. ) ;
#11464=EDGE_CURVE ( 'NONE', #25758, #26019, #13313, .T. ) ;
#11465=CARTESIAN_POINT ( 'NONE',  ( -449.9999999999999432, -125.0000000000000000, 162.9999999999999716 ) ) ;
#11471=VECTOR ( 'NONE', #25923, 1000.000000000000000 ) ;
#11473=VERTEX_POINT ( 'NONE', #16338 ) ;
#11480=DIRECTION ( 'NONE',  ( 1.000000000000000000, 0.000000000000000000, 0.000000000000000000 ) ) ;
#11483=CARTESIAN_POINT ( 'NONE',  ( 11.99999999999999645, -109.0000000000000142, -155.0000000000000284 ) ) ;
#11487=AXIS2_PLACEMENT_3D ( 'NONE', #3832, #14550, #9374 ) ;
#11493=ORIENTED_EDGE ( 'NONE', *, *, #13517, .T. ) ;
#11494=AXIS2_PLACEMENT_3D ( 'NONE', #11361, #14032, #14213 ) ;
#11497=ORIENTED_EDGE ( 'NONE', *, *, #22105, .T. ) ;
#11501=ORIENTED_EDGE ( 'NONE', *, *, #2504, .F. ) ;
#11504=DIRECTION ( 'NONE',  ( -1.000000000000000000, 0.000000000000000000, -5.546364386991661285E-52 ) ) ;
#11506=FACE_OUTER_BOUND ( 'NONE', #12908, .T. ) ;
#11508=ORIENTED_EDGE ( 'NONE', *, *, #1691, .T. ) ;
#11512=DIRECTION ( 'NONE',  ( 1.000000000000000000, 3.040835319149746528E-31, 1.232595164407830946E-32 ) ) ;
#11513=CARTESIAN_POINT ( 'NONE',  ( -345.0000000000000000, -125.0000000000000284, 113.9999999999999858 ) ) ;
#11518=CARTESIAN_POINT ( 'NONE',  ( -20.00000000000007461, 112.9999999999999574, 190.9999999999999716 ) ) ;
#11519=EDGE_LOOP ( 'NONE', ( #3533, #25494, #21180, #17939, #31296 ) ) ;
#11528=VECTOR ( 'NONE', #22197, 1000.000000000000000 ) ;
#11529=FACE_OUTER_BOUND ( 'NONE', #19312, .T. ) ;
#11530=ORIENTED_EDGE ( 'NONE', *, *, #17909, .T. ) ;
#11531=CARTESIAN_POINT ( 'NONE',  ( -430.0000000000000000, 130.9999999999999716, 109.9999999999999858 ) ) ;
#11532=CARTESIAN_POINT ( 'NONE',  ( -430.0000000000000000, 118.9999999999999858, 128.0000000000000000 ) ) ;
#11535=EDGE_CURVE ( 'NONE', #7282, #9737, #8380, .T. ) ;
#11538=PLANE ( 'NONE',  #17387 ) ;
#11539=PLANE ( 'NONE',  #16636 ) ;
#11542=CARTESIAN_POINT ( 'NONE',  ( 19.99999999999998934, 136.9999999999999716, -175.0000000000000284 ) ) ;
#11548=DIRECTION ( 'NONE',  ( 0.000000000000000000, 0.000000000000000000, 1.000000000000000000 ) ) ;
#11551=EDGE_CURVE ( 'NONE', #23608, #16235, #652, .T. ) ;
#11554=VERTEX_POINT ( 'NONE', #22364 ) ;
#11556=ORIENTED_EDGE ( 'NONE', *, *, #18335, .F. ) ;
#11564=ORIENTED_EDGE ( 'NONE', *, *, #29447, .T. ) ;
#11568=VERTEX_POINT ( 'NONE', #27522 ) ;
#11570=AXIS2_PLACEMENT_3D ( 'NONE', #12013, #17710, #28020 ) ;
#11574=LINE ( 'NONE', #22425, #8959 ) ;
#11576=LINE ( 'NONE', #19591, #26345 ) ;
#11577=EDGE_CURVE ( 'NONE', #3035, #30605, #19528, .T. ) ;
#11583=DIRECTION ( 'NONE',  ( -0.000000000000000000, 1.000000000000000000, -0.000000000000000000 ) ) ;
#11584=FACE_OUTER_BOUND ( 'NONE', #32371, .T. ) ;
#11588=ORIENTED_EDGE ( 'NONE', *, *, #19019, .F. ) ;
#11590=EDGE_CURVE ( 'NONE', #31738, #1594, #20057, .T. ) ;
#11597=VERTEX_POINT ( 'NONE', #19883 ) ;
#11604=ORIENTED_EDGE ( 'NONE', *, *, #6962, .T. ) ;
#11606=AXIS2_PLACEMENT_3D ( 'NONE', #1416, #7084, #33978 ) ;
#11608=EDGE_CURVE ( 'NONE', #904, #28532, #19760, .T. ) ;
#11610=DIRECTION ( 'NONE',  ( 1.000000000000000000, 3.469446951953834515E-18, 0.000000000000000000 ) ) ;
#11612=VERTEX_POINT ( 'NONE', #22726 ) ;
#11614=CARTESIAN_POINT ( 'NONE',  ( 11.99999999999999645, 134.9999999999999432, -162.9999999999999432 ) ) ;
#11615=CARTESIAN_POINT ( 'NONE',  ( -19.99999999999996092, -137.0000000000000284, 155.0000000000000000 ) ) ;
#11616=ORIENTED_EDGE ( 'NONE', *, *, #18537, .F. ) ;
#11617=CARTESIAN_POINT ( 'NONE',  ( -418.0000000000000000, 104.9999999999999858, -187.0000000000000000 ) ) ;
#11618=EDGE_CURVE ( 'NONE', #9444, #10934, #33561, .T. ) ;
#11622=CARTESIAN_POINT ( 'NONE',  ( -345.0000000000000000, 124.9999999999999432, 181.0000000000000000 ) ) ;
#11624=ADVANCED_FACE ( 'NONE', ( #34264 ), #26078, .T. ) ;
#11627=CARTESIAN_POINT ( 'NONE',  ( -418.0000000000000000, -104.9999999999999858, -194.9999999999999716 ) ) ;
#11628=CARTESIAN_POINT ( 'NONE',  ( -365.0000000000000000, 130.9999999999999716, 110.0000000000000000 ) ) ;
#11631=VECTOR ( 'NONE', #6999, 1000.000000000000000 ) ;
#11632=ORIENTED_EDGE ( 'NONE', *, *, #6856, .F. ) ;
#11633=AXIS2_PLACEMENT_3D ( 'NONE', #13067, #23895, #21238 ) ;
#11637=DIRECTION ( 'NONE',  ( -0.000000000000000000, 5.145227585319922065E-49, 1.000000000000000000 ) ) ;
#11639=VERTEX_POINT ( 'NONE', #12052 ) ;
#11643=EDGE_LOOP ( 'NONE', ( #11455, #31372, #32326, #6304 ) ) ;
#11646=ORIENTED_EDGE ( 'NONE', *, *, #15353, .F. ) ;
#11647=VERTEX_POINT ( 'NONE', #9546 ) ;
#11648=PLANE ( 'NONE',  #31053 ) ;
#11653=CARTESIAN_POINT ( 'NONE',  ( -12.00000000000001066, 144.9999999999999716, 190.9999999999999716 ) ) ;
#11655=CARTESIAN_POINT ( 'NONE',  ( 19.99999999999998224, 144.9999999999999716, -162.9999999999999432 ) ) ;
#11657=CIRCLE ( 'NONE', #31500, 7.999999999999992895 ) ;
#11659=EDGE_LOOP ( 'NONE', ( #20607, #24920, #12100, #29352 ) ) ;
#11671=LINE ( 'NONE', #22521, #33775 ) ;
#11674=AXIS2_PLACEMENT_3D ( 'NONE', #23192, #6970, #17688 ) ;
#11675=VERTEX_POINT ( 'NONE', #28409 ) ;
#11677=DIRECTION ( 'NONE',  ( 0.000000000000000000, -1.224646799147353207E-16, 1.000000000000000000 ) ) ;
#11682=ORIENTED_EDGE ( 'NONE', *, *, #4109, .T. ) ;
#11683=PLANE ( 'NONE',  #15674 ) ;
#11688=DIRECTION ( 'NONE',  ( -3.469446951953832974E-18, -1.000000000000000000, -7.888609052210116302E-31 ) ) ;
#11694=CARTESIAN_POINT ( 'NONE',  ( -414.0000000000000568, -137.0000000000000000, -175.0000000000000000 ) ) ;
#11701=AXIS2_PLACEMENT_3D ( 'NONE', #15026, #25870, #970 ) ;
#11705=DIRECTION ( 'NONE',  ( 0.000000000000000000, 0.000000000000000000, 1.000000000000000000 ) ) ;
#11708=ORIENTED_EDGE ( 'NONE', *, *, #10961, .T. ) ;
#11714=ORIENTED_EDGE ( 'NONE', *, *, #10434, .F. ) ;
#11716=ADVANCED_FACE ( 'NONE', ( #22895 ), #7023, .F. ) ;
#11717=DIRECTION ( 'NONE',  ( 0.000000000000000000, -5.053935297177146739E-49, -1.000000000000000000 ) ) ;
#11718=DIRECTION ( 'NONE',  ( -1.000000000000000000, 0.000000000000000000, 0.000000000000000000 ) ) ;
#11720=EDGE_CURVE ( 'NONE', #7256, #34152, #33741, .T. ) ;
#11721=ORIENTED_EDGE ( 'NONE', *, *, #11104, .T. ) ;
#11724=EDGE_LOOP ( 'NONE', ( #27088, #23566, #33815, #8143 ) ) ;
#11727=EDGE_CURVE ( 'NONE', #5950, #28571, #6699, .T. ) ;
#11729=DIRECTION ( 'NONE',  ( 0.000000000000000000, 0.000000000000000000, 1.000000000000000000 ) ) ;
#11732=ORIENTED_EDGE ( 'NONE', *, *, #16910, .T. ) ;
#11735=EDGE_LOOP ( 'NONE', ( #10099, #24259, #20698, #4583 ) ) ;
#11736=DIRECTION ( 'NONE',  ( -1.232595164407830946E-32, 0.000000000000000000, -1.000000000000000000 ) ) ;
#11739=CARTESIAN_POINT ( 'NONE',  ( -12.00000000000001066, 134.9999999999998863, 155.0000000000000000 ) ) ;
#11742=CIRCLE ( 'NONE', #935, 7.999999999999979572 ) ;
#11747=DIRECTION ( 'NONE',  ( 0.000000000000000000, 1.000000000000000000, 5.053935297177146739E-49 ) ) ;
#11749=ORIENTED_EDGE ( 'NONE', *, *, #6943, .T. ) ;
#11755=ORIENTED_EDGE ( 'NONE', *, *, #3119, .T. ) ;
#11759=DIRECTION ( 'NONE',  ( 1.848892746611746419E-32, 6.842277657836020854E-49, -1.000000000000000000 ) ) ;
#11762=EDGE_CURVE ( 'NONE', #27942, #14836, #23078, .T. ) ;
#11764=DIRECTION ( 'NONE',  ( 1.000000000000000000, 0.000000000000000000, 0.000000000000000000 ) ) ;
#11767=ORIENTED_EDGE ( 'NONE', *, *, #26142, .T. ) ;
#11770=ORIENTED_EDGE ( 'NONE', *, *, #29202, .F. ) ;
#11776=CARTESIAN_POINT ( 'NONE',  ( 15.99999999999998579, 136.9999999999999716, 155.0000000000000000 ) ) ;
#11781=EDGE_CURVE ( 'NONE', #30234, #18803, #34799, .T. ) ;
#11785=DIRECTION ( 'NONE',  ( -1.232595164407830946E-32, -7.496237820289040735E-63, 1.000000000000000000 ) ) ;
#11786=ORIENTED_EDGE ( 'NONE', *, *, #6338, .F. ) ;
#11787=VERTEX_POINT ( 'NONE', #16114 ) ;
#11788=DIRECTION ( 'NONE',  ( 0.000000000000000000, 1.000000000000000000, 5.053935297177146739E-49 ) ) ;
#11791=DIRECTION ( 'NONE',  ( 0.000000000000000000, 1.000000000000000000, -3.374343856708137958E-53 ) ) ;
#11796=PRODUCT_DEFINITION_SHAPE ( 'NONE', 'NONE',  #13389 ) ;
#11799=PLANE ( 'NONE',  #27709 ) ;
#11800=AXIS2_PLACEMENT_3D ( 'NONE', #13099, #10605, #33801 ) ;
#11801=DIRECTION ( 'NONE',  ( -1.848892746611746966E-32, 6.842277657836020854E-49, -1.000000000000000000 ) ) ;
#11804=CARTESIAN_POINT ( 'NONE',  ( -418.0000000000000000, -137.0000000000000000, -155.0000000000000000 ) ) ;
#11808=UNCERTAINTY_MEASURE_WITH_UNIT (LENGTH_MEASURE( 1.000000000000000082E-05 ), #9432, 'distance_accuracy_value', 'NONE');
#11809=DIRECTION ( 'NONE',  ( 0.000000000000000000, 2.309213040847544338E-50, 1.000000000000000000 ) ) ;
#11811=VERTEX_POINT ( 'NONE', #32113 ) ;
#11814=VECTOR ( 'NONE', #8122, 1000.000000000000000 ) ;
#11815=EDGE_LOOP ( 'NONE', ( #13504, #27421, #15013, #10180 ) ) ;
#11818=ORIENTED_EDGE ( 'NONE', *, *, #34181, .F. ) ;
#11820=EDGE_LOOP ( 'NONE', ( #30355, #25087, #21618, #19228 ) ) ;
#11821=LINE ( 'NONE', #22669, #4764 ) ;
#11824=DIRECTION ( 'NONE',  ( 0.000000000000000000, 0.000000000000000000, -1.000000000000000000 ) ) ;
#11829=CARTESIAN_POINT ( 'NONE',  ( -361.0000000000000000, 124.9999999999999432, 181.0000000000000000 ) ) ;
#11831=VERTEX_POINT ( 'NONE', #27124 ) ;
#11835=MANIFOLD_SOLID_BREP ( 'Square tube 40 X 40 X 4(1)[14]', #17781 ) ;
#11839=VERTEX_POINT ( 'NONE', #31929 ) ;
#11847=CARTESIAN_POINT ( 'NONE',  ( -363.0000000000000000, -125.0000000000000284, 168.9999999999999716 ) ) ;
#11848=CARTESIAN_POINT ( 'NONE',  ( -349.0000000000000000, -125.0000000000000284, 168.9999999999999716 ) ) ;
#11849=AXIS2_PLACEMENT_3D ( 'NONE', #19659, #18952, #8250 ) ;
#11850=LINE ( 'NONE', #33535, #3042 ) ;
#11851=ORIENTED_EDGE ( 'NONE', *, *, #20531, .F. ) ;
#11854=CARTESIAN_POINT ( 'NONE',  ( -19.99999999999998934, 134.9999999999999432, -186.9999999999999716 ) ) ;
#11855=AXIS2_PLACEMENT_3D ( 'NONE', #7625, #5346, #27032 ) ;
#11857=CARTESIAN_POINT ( 'NONE',  ( 11.99999999999999645, -137.0000000000000000, 174.9999999999999432 ) ) ;
#11858=ORIENTED_EDGE ( 'NONE', *, *, #27755, .T. ) ;
#11870=AXIS2_PLACEMENT_3D ( 'NONE', #16597, #16778, #3219 ) ;
#11872=PLANE ( 'NONE',  #34728 ) ;
#11874=ORIENTED_EDGE ( 'NONE', *, *, #23785, .F. ) ;
#11876=CARTESIAN_POINT ( 'NONE',  ( -430.0000000000000000, 116.9999999999999716, 113.9999999999999858 ) ) ;
#11878=DIRECTION ( 'NONE',  ( 0.000000000000000000, 0.000000000000000000, -1.000000000000000000 ) ) ;
#11885=DIRECTION ( 'NONE',  ( 0.000000000000000000, -1.224646799147353207E-16, 1.000000000000000000 ) ) ;
#11886=VECTOR ( 'NONE', #28059, 1000.000000000000000 ) ;
#11887=CARTESIAN_POINT ( 'NONE',  ( -349.0000000000000000, -135.0000000000000000, 109.9999999999999858 ) ) ;
#11888=ORIENTED_EDGE ( 'NONE', *, *, #31740, .T. ) ;
#11889=CARTESIAN_POINT ( 'NONE',  ( -365.0000000000000000, 118.9999999999999858, 128.0000000000000000 ) ) ;
#11891=LINE ( 'NONE', #14208, #24713 ) ;
#11895=DIRECTION ( 'NONE',  ( -1.232595164407830946E-32, 0.000000000000000000, -1.000000000000000000 ) ) ;
#11896=DIRECTION ( 'NONE',  ( 0.000000000000000000, 1.310824597558155437E-49, 1.000000000000000000 ) ) ;
#11899=AXIS2_PLACEMENT_3D ( 'NONE', #27425, #24225, #8554 ) ;
#11912=ORIENTED_EDGE ( 'NONE', *, *, #16108, .T. ) ;
#11914=DIRECTION ( 'NONE',  ( 1.000000000000000000, 3.469446951953834515E-18, 0.000000000000000000 ) ) ;
#11915=DIRECTION ( 'NONE',  ( 1.000000000000000000, 0.000000000000000000, 0.000000000000000000 ) ) ;
#11918=ORIENTED_EDGE ( 'NONE', *, *, #2677, .T. ) ;
#11919=ADVANCED_FACE ( 'NONE', ( #8969 ), #3434, .T. ) ;
#11920=LINE ( 'NONE', #33969, #5489 ) ;
#11922=VERTEX_POINT ( 'NONE', #24801 ) ;
#11924=EDGE_CURVE ( 'NONE', #11597, #24095, #601, .T. ) ;
#11925=CARTESIAN_POINT ( 'NONE',  ( -12.00000000000003908, -134.9999999999999716, -154.9999999999999716 ) ) ;
#11926=ORIENTED_EDGE ( 'NONE', *, *, #32742, .F. ) ;
#11927=EDGE_CURVE ( 'NONE', #33325, #31534, #32978, .T. ) ;
#11930=PLANE ( 'NONE',  #25975 ) ;
#11932=VERTEX_POINT ( 'NONE', #30682 ) ;
#11933=CARTESIAN_POINT ( 'NONE',  ( -20.00000000000004619, 112.9999999999999574, -194.9999999999999432 ) ) ;
#11934=DIRECTION ( 'NONE',  ( 0.000000000000000000, -1.000000000000000000, 0.000000000000000000 ) ) ;
#11936=AXIS2_PLACEMENT_3D ( 'NONE', #8638, #3123, #34033 ) ;
#11938=DIRECTION ( 'NONE',  ( 0.000000000000000000, 0.000000000000000000, -1.000000000000000000 ) ) ;
#11939=( LENGTH_UNIT ( ) NAMED_UNIT ( * ) SI_UNIT ( .MILLI., .METRE. ) );
#11942=ORIENTED_EDGE ( 'NONE', *, *, #9797, .F. ) ;
#11954=EDGE_CURVE ( 'NONE', #27889, #28881, #25329, .T. ) ;
#11965=FACE_OUTER_BOUND ( 'NONE', #29026, .T. ) ;
#11974=DIRECTION ( 'NONE',  ( 0.000000000000000000, -7.888609052210118054E-31, -1.000000000000000000 ) ) ;
#11976=DIRECTION ( 'NONE',  ( -0.000000000000000000, -0.000000000000000000, -1.000000000000000000 ) ) ;
#11988=VERTEX_POINT ( 'NONE', #30143 ) ;
#11994=CARTESIAN_POINT ( 'NONE',  ( 11.99999999999995559, -134.9999999999999716, -162.9999999999999432 ) ) ;
#11996=ORIENTED_EDGE ( 'NONE', *, *, #30431, .F. ) ;
#11997=ORIENTED_EDGE ( 'NONE', *, *, #24859, .F. ) ;
#12007=DIRECTION ( 'NONE',  ( 1.232595164407830946E-32, 0.000000000000000000, 1.000000000000000000 ) ) ;
#12008=CARTESIAN_POINT ( 'NONE',  ( -361.0000000000000000, -125.0000000000000284, 110.0000000000000000 ) ) ;
#12013=CARTESIAN_POINT ( 'NONE',  ( 11.99999999999999645, 144.9999999999999716, -162.9999999999999432 ) ) ;
#12014=DIRECTION ( 'NONE',  ( 1.000000000000000000, 0.000000000000000000, 0.000000000000000000 ) ) ;
#12015=CARTESIAN_POINT ( 'NONE',  ( -12.00000000000003908, -134.9999999999999716, -194.9999999999999432 ) ) ;
#12019=LINE ( 'NONE', #17551, #18416 ) ;
#12021=ORIENTED_EDGE ( 'NONE', *, *, #15033, .T. ) ;
#12025=CARTESIAN_POINT ( 'NONE',  ( -445.9999999999999432, 104.9999999999999858, -162.9999999999999716 ) ) ;
#12026=ADVANCED_FACE ( 'NONE', ( #3958 ), #31547, .F. ) ;
#12030=VECTOR ( 'NONE', #19843, 1000.000000000000000 ) ;
#12031=EDGE_CURVE ( 'NONE', #29779, #15405, #4306, .T. ) ;
#12037=ORIENTED_EDGE ( 'NONE', *, *, #34636, .F. ) ;
#12039=CYLINDRICAL_SURFACE ( 'NONE', #3671, 2.000000000000001776 ) ;
#12041=FACE_BOUND ( 'NONE', #4556, .T. ) ;
#12046=ORIENTED_EDGE ( 'NONE', *, *, #32844, .F. ) ;
#12049=CARTESIAN_POINT ( 'NONE',  ( -499.9999999999999432, 112.9999999999999574, -155.0000000000000000 ) ) ;
#12051=AXIS2_PLACEMENT_3D ( 'NONE', #26702, #13538, #366 ) ;
#12052=CARTESIAN_POINT ( 'NONE',  ( 19.99999999999998934, 144.9999999999999716, -162.9999999999999432 ) ) ;
#12053=FACE_OUTER_BOUND ( 'NONE', #34006, .T. ) ;
#12054=DIRECTION ( 'NONE',  ( 1.000000000000000000, -0.000000000000000000, -0.000000000000000000 ) ) ;
#12055=FACE_OUTER_BOUND ( 'NONE', #31079, .T. ) ;
#12056=CARTESIAN_POINT ( 'NONE',  ( -12.00000000000001066, 134.9999999999998863, 187.0000000000000000 ) ) ;
#12057=ORIENTED_EDGE ( 'NONE', *, *, #27974, .F. ) ;
#12060=LINE ( 'NONE', #9379, #21146 ) ;
#12061=VECTOR ( 'NONE', #16160, 1000.000000000000000 ) ;
#12062=DIRECTION ( 'NONE',  ( 0.000000000000000000, -1.000000000000000000, 5.053935297177146739E-49 ) ) ;
#12063=ORIENTED_EDGE ( 'NONE', *, *, #1841, .T. ) ;
#12069=VECTOR ( 'NONE', #23987, 1000.000000000000000 ) ;
#12070=EDGE_CURVE ( 'NONE', #13149, #15074, #4422, .T. ) ;
#12071=VECTOR ( 'NONE', #1017, 1000.000000000000000 ) ;
#12075=CARTESIAN_POINT ( 'NONE',  ( 11.99999999999999645, -141.0000000000000000, 155.0000000000000000 ) ) ;
#12080=DIRECTION ( 'NONE',  ( 0.000000000000000000, 0.000000000000000000, 1.000000000000000000 ) ) ;
#12082=DIRECTION ( 'NONE',  ( -1.000000000000000000, 0.000000000000000000, 0.000000000000000000 ) ) ;
#12085=PLANE ( 'NONE',  #43 ) ;
#12088=EDGE_LOOP ( 'NONE', ( #18071, #19683, #34676, #9459 ) ) ;
#12089=ORIENTED_EDGE ( 'NONE', *, *, #10011, .T. ) ;
#12091=( NAMED_UNIT ( * ) PLANE_ANGLE_UNIT ( ) SI_UNIT ( $, .RADIAN. ) );
#12094=CARTESIAN_POINT ( 'NONE',  ( 11.99999999999999645, 136.9999999999999716, -175.0000000000000284 ) ) ;
#12095=AXIS2_PLACEMENT_3D ( 'NONE', #13366, #26047, #18714 ) ;
#12096=VECTOR ( 'NONE', #17718, 1000.000000000000000 ) ;
#12098=MECHANICAL_DESIGN_GEOMETRIC_PRESENTATION_REPRESENTATION('',(#22882),#7511);
#12100=ORIENTED_EDGE ( 'NONE', *, *, #1025, .F. ) ;
#12104=PLANE ( 'NONE',  #11800 ) ;
#12105=EDGE_CURVE ( 'NONE', #7140, #12748, #12348, .T. ) ;
#12109=CARTESIAN_POINT ( 'NONE',  ( -12.00000000000001066, 144.9999999999999716, 155.0000000000000000 ) ) ;
#12110=ADVANCED_FACE ( 'NONE', ( #28705 ), #4133, .T. ) ;
#12113=DIRECTION ( 'NONE',  ( -0.000000000000000000, 1.000000000000000000, -0.000000000000000000 ) ) ;
#12116=FACE_OUTER_BOUND ( 'NONE', #18041, .T. ) ;
#12118=ORIENTED_EDGE ( 'NONE', *, *, #18806, .F. ) ;
#12123=AXIS2_PLACEMENT_3D ( 'NONE', #15601, #26788, #7208 ) ;
#12126=LINE ( 'NONE', #3558, #481 ) ;
#12128=EDGE_LOOP ( 'NONE', ( #27441, #5758, #9864, #8964 ) ) ;
#12134=EDGE_LOOP ( 'NONE', ( #19018, #22723, #14662, #17485 ) ) ;
#12137=CARTESIAN_POINT ( 'NONE',  ( -499.9999999999999432, 136.9999999999999432, 190.9999999999999716 ) ) ;
#12141=CARTESIAN_POINT ( 'NONE',  ( -12.00000000000001066, -145.0000000000000000, 159.0000000000000000 ) ) ;
#12143=LINE ( 'NONE', #34496, #34234 ) ;
#12147=DIRECTION ( 'NONE',  ( 0.000000000000000000, -7.888609052210118054E-31, -1.000000000000000000 ) ) ;
#12150=CARTESIAN_POINT ( 'NONE',  ( -349.0000000000000000, -125.0000000000000284, 128.0000000000000000 ) ) ;
#12153=CARTESIAN_POINT ( 'NONE',  ( -445.9999999999999432, 137.0000000000000000, -175.0000000000000000 ) ) ;
#12156=DIRECTION ( 'NONE',  ( 1.000000000000000000, 0.000000000000000000, 0.000000000000000000 ) ) ;
#12157=LINE ( 'NONE', #4455, #12697 ) ;
#12161=EDGE_LOOP ( 'NONE', ( #9956, #17862, #20973, #33833, #9612 ) ) ;
#12162=EDGE_CURVE ( 'NONE', #35069, #2443, #15908, .T. ) ;
#12164=ORIENTED_EDGE ( 'NONE', *, *, #31257, .T. ) ;
#12169=ORIENTED_EDGE ( 'NONE', *, *, #14532, .F. ) ;
#12172=DIRECTION ( 'NONE',  ( -1.000000000000000000, 0.000000000000000000, 0.000000000000000000 ) ) ;
#12181=CARTESIAN_POINT ( 'NONE',  ( -410.0000000000000568, -124.9999999999999716, 132.0000000000000000 ) ) ;
#12184=LINE ( 'NONE', #20190, #12030 ) ;
#12185=ORIENTED_EDGE ( 'NONE', *, *, #1570, .T. ) ;
#12187=DIRECTION ( 'NONE',  ( 0.000000000000000000, -0.000000000000000000, -1.000000000000000000 ) ) ;
#12188=CARTESIAN_POINT ( 'NONE',  ( 12.00000000000001066, -134.9999999999999716, 187.0000000000000000 ) ) ;
#12189=AXIS2_PLACEMENT_3D ( 'NONE', #17037, #9005, #3303 ) ;
#12192=ORIENTED_EDGE ( 'NONE', *, *, #34837, .T. ) ;
#12195=CARTESIAN_POINT ( 'NONE',  ( -349.0000000000000000, -125.0000000000000284, 183.0000000000000000 ) ) ;
#12196=PRODUCT_DEFINITION_FORMATION_WITH_SPECIFIED_SOURCE ( 'ANY', '', #695, .NOT_KNOWN. ) ;
#12199=VECTOR ( 'NONE', #12327, 1000.000000000000000 ) ;
#12200=AXIS2_PLACEMENT_3D ( 'NONE', #17717, #1155, #19857 ) ;
#12201=CARTESIAN_POINT ( 'NONE',  ( -349.0000000000000000, -135.0000000000000000, 126.0000000000000000 ) ) ;
#12204=DIRECTION ( 'NONE',  ( 0.000000000000000000, 3.374343856708137958E-53, -1.000000000000000000 ) ) ;
#12207=VERTEX_POINT ( 'NONE', #31717 ) ;
#12213=VECTOR ( 'NONE', #29446, 1000.000000000000000 ) ;
#12224=ORIENTED_EDGE ( 'NONE', *, *, #924, .T. ) ;
#12225=ORIENTED_EDGE ( 'NONE', *, *, #13585, .T. ) ;
#12230=EDGE_CURVE ( 'NONE', #17921, #33397, #26556, .T. ) ;
#12235=CARTESIAN_POINT ( 'NONE',  ( -20.00000000000007461, 104.9999999999999858, 187.0000000000000000 ) ) ;
#12240=LINE ( 'NONE', #19715, #6344 ) ;
#12242=ORIENTED_EDGE ( 'NONE', *, *, #687, .F. ) ;
#12243=VECTOR ( 'NONE', #3388, 1000.000000000000000 ) ;
#12245=DIRECTION ( 'NONE',  ( 0.000000000000000000, 0.000000000000000000, 1.000000000000000000 ) ) ;
#12251=VECTOR ( 'NONE', #26884, 1000.000000000000000 ) ;
#12259=FACE_OUTER_BOUND ( 'NONE', #9003, .T. ) ;
#12260=CIRCLE ( 'NONE', #8274, 7.999999999999979572 ) ;
#12261=CYLINDRICAL_SURFACE ( 'NONE', #17369, 4.000000000000003553 ) ;
#12264=VERTEX_POINT ( 'NONE', #13221 ) ;
#12266=ORIENTED_EDGE ( 'NONE', *, *, #21763, .T. ) ;
#12268=LINE ( 'NONE', #31124, #24864 ) ;
#12269=VECTOR ( 'NONE', #26084, 1000.000000000000000 ) ;
#12277=DIRECTION ( 'NONE',  ( -0.000000000000000000, -1.000000000000000000, -0.000000000000000000 ) ) ;
#12282=CARTESIAN_POINT ( 'NONE',  ( -500.0000000000000000, -113.0000000000000000, 190.9999999999999716 ) ) ;
#12284=ORIENTED_EDGE ( 'NONE', *, *, #34112, .T. ) ;
#12287=FACE_BOUND ( 'NONE', #23759, .T. ) ;
#12288=AXIS2_PLACEMENT_3D ( 'NONE', #11119, #30681, #13786 ) ;
#12290=DIRECTION ( 'NONE',  ( 1.000000000000000000, 0.000000000000000000, 0.000000000000000000 ) ) ;
#12294=EDGE_LOOP ( 'NONE', ( #31138, #6796, #7185, #20705, #24433, #26340, #5425, #21031 ) ) ;
#12300=DIRECTION ( 'NONE',  ( 1.000000000000000000, 0.000000000000000000, -0.000000000000000000 ) ) ;
#12302=DIRECTION ( 'NONE',  ( 1.000000000000000000, 0.000000000000000000, -1.848892746611746966E-32 ) ) ;
#12305=CIRCLE ( 'NONE', #29344, 4.750000000000004441 ) ;
#12307=LINE ( 'NONE', #15146, #16760 ) ;
#12308=CYLINDRICAL_SURFACE ( 'NONE', #32876, 7.999999999999979572 ) ;
#12311=LINE ( 'NONE', #20316, #12894 ) ;
#12319=VERTEX_POINT ( 'NONE', #2865 ) ;
#12327=DIRECTION ( 'NONE',  ( 0.000000000000000000, 5.053935297177146739E-49, 1.000000000000000000 ) ) ;
#12329=ORIENTED_EDGE ( 'NONE', *, *, #2842, .T. ) ;
#12332=VECTOR ( 'NONE', #1999, 1000.000000000000000 ) ;
#12333=ORIENTED_EDGE ( 'NONE', *, *, #25258, .F. ) ;
#12336=DIRECTION ( 'NONE',  ( -1.000000000000000000, 0.000000000000000000, 0.000000000000000000 ) ) ;
#12339=ORIENTED_EDGE ( 'NONE', *, *, #31026, .T. ) ;
#12341=EDGE_CURVE ( 'NONE', #15752, #1095, #16409, .T. ) ;
#12344=LINE ( 'NONE', #25857, #31342 ) ;
#12345=ORIENTED_EDGE ( 'NONE', *, *, #22390, .T. ) ;
#12348=LINE ( 'NONE', #17874, #24325 ) ;
#12351=ADVANCED_FACE ( 'NONE', ( #24573 ), #19096, .T. ) ;
#12352=FACE_OUTER_BOUND ( 'NONE', #29460, .T. ) ;
#12355=EDGE_LOOP ( 'NONE', ( #15753, #33728, #20863, #27836 ) ) ;
#12357=AXIS2_PLACEMENT_3D ( 'NONE', #15638, #2436, #20619 ) ;
#12359=CARTESIAN_POINT ( 'NONE',  ( -499.9999999999999432, 104.9999999999999858, -187.0000000000000000 ) ) ;
#12360=EDGE_CURVE ( 'NONE', #31191, #639, #10733, .T. ) ;
#12362=CARTESIAN_POINT ( 'NONE',  ( -418.0000000000000000, -105.0000000000000142, 135.9999999999999716 ) ) ;
#12368=CARTESIAN_POINT ( 'NONE',  ( -499.9999999999999432, 112.9999999999999574, 194.9999999999999716 ) ) ;
#12388=DIRECTION ( 'NONE',  ( -1.000000000000000000, 0.000000000000000000, 0.000000000000000000 ) ) ;
#12392=ORIENTED_EDGE ( 'NONE', *, *, #130, .T. ) ;
#12393=ORIENTED_EDGE ( 'NONE', *, *, #23070, .F. ) ;
#12395=DIRECTION ( 'NONE',  ( -1.000000000000000000, 0.000000000000000000, -1.292961597001347186E-16 ) ) ;
#12397=EDGE_CURVE ( 'NONE', #19123, #108, #33610, .T. ) ;
#12398=CARTESIAN_POINT ( 'NONE',  ( -445.9999999999999432, 137.0000000000000000, -155.0000000000000000 ) ) ;
#12399=CARTESIAN_POINT ( 'NONE',  ( -12.00000000000001066, 124.9999999999999716, 155.0000000000000000 ) ) ;
#12400=VERTEX_POINT ( 'NONE', #22104 ) ;
#12404=EDGE_CURVE ( 'NONE', #8355, #28881, #30621, .T. ) ;
#12406=ORIENTED_EDGE ( 'NONE', *, *, #24178, .F. ) ;
#12408=CARTESIAN_POINT ( 'NONE',  ( -442.0000000000000000, 124.9999999999999432, -159.0000000000000000 ) ) ;
#12409=CARTESIAN_POINT ( 'NONE',  ( -20.00000000000004619, -134.9999999999999716, -186.9999999999999716 ) ) ;
#12415=VERTEX_POINT ( 'NONE', #27257 ) ;
#12417=CARTESIAN_POINT ( 'NONE',  ( -500.0000000000000000, -137.0000000000000000, 155.0000000000000000 ) ) ;
#12419=VECTOR ( 'NONE', #8082, 1000.000000000000000 ) ;
#12421=DIRECTION ( 'NONE',  ( 0.000000000000000000, 0.000000000000000000, 1.000000000000000000 ) ) ;
#12422=CARTESIAN_POINT ( 'NONE',  ( -418.0000000000000000, -125.0000000000000000, -101.9999999999999858 ) ) ;
#12423=EDGE_CURVE ( 'NONE', #30526, #15904, #32308, .T. ) ;
#12425=EDGE_CURVE ( 'NONE', #10776, #28035, #11075, .T. ) ;
#12427=VECTOR ( 'NONE', #14802, 1000.000000000000000 ) ;
#12429=ORIENTED_EDGE ( 'NONE', *, *, #6455, .F. ) ;
#12435=CIRCLE ( 'NONE', #5555, 4.000000000000003553 ) ;
#12437=LINE ( 'NONE', #10095, #3439 ) ;
#12439=ORIENTED_EDGE ( 'NONE', *, *, #29512, .T. ) ;
#12442=CARTESIAN_POINT ( 'NONE',  ( -430.0000000000000000, -133.0000000000000000, 126.0000000000000000 ) ) ;
#12443=CARTESIAN_POINT ( 'NONE',  ( -442.0000000000000000, 144.9999999999999716, 155.0000000000000000 ) ) ;
#12444=CIRCLE ( 'NONE', #7894, 2.000000000000001776 ) ;
#12445=CARTESIAN_POINT ( 'NONE',  ( -499.9999999999999432, -113.0000000000000000, -159.0000000000000000 ) ) ;
#12446=CYLINDRICAL_SURFACE ( 'NONE', #27874, 2.000000000000001776 ) ;
#12448=CARTESIAN_POINT ( 'NONE',  ( 11.99999999999999645, 144.9999999999999716, -162.9999999999999432 ) ) ;
#12453=VERTEX_POINT ( 'NONE', #8211 ) ;
#12456=ORIENTED_EDGE ( 'NONE', *, *, #16649, .F. ) ;
#12463=EDGE_LOOP ( 'NONE', ( #788, #4068 ) ) ;
#12465=EDGE_CURVE ( 'NONE', #17491, #20271, #12444, .T. ) ;
#12472=CARTESIAN_POINT ( 'NONE',  ( -15.99999999999998579, 75.55999999999990280, 168.2400000000000091 ) ) ;
#12475=DIRECTION ( 'NONE',  ( -1.848892746611746419E-32, -6.842277657836020854E-49, 1.000000000000000000 ) ) ;
#12477=DIRECTION ( 'NONE',  ( 0.000000000000000000, 0.000000000000000000, -1.000000000000000000 ) ) ;
#12480=ORIENTED_EDGE ( 'NONE', *, *, #29998, .T. ) ;
#12481=DIRECTION ( 'NONE',  ( -1.000000000000000000, 0.000000000000000000, -5.546364386991661285E-52 ) ) ;
#12482=MANIFOLD_SOLID_BREP ( 'Square tube 40 X 40 X 4(1)[15]', #30985 ) ;
#12485=ORIENTED_EDGE ( 'NONE', *, *, #15512, .T. ) ;
#12487=LINE ( 'NONE', #34535, #19722 ) ;
#12489=EDGE_CURVE ( 'NONE', #24841, #33545, #17975, .T. ) ;
#12490=DIRECTION ( 'NONE',  ( -0.000000000000000000, -1.000000000000000000, -0.000000000000000000 ) ) ;
#12493=CARTESIAN_POINT ( 'NONE',  ( -442.0000000000000000, -125.0000000000000000, 162.9999999999999716 ) ) ;
#12495=LINE ( 'NONE', #9808, #32724 ) ;
#12498=DIRECTION ( 'NONE',  ( -0.000000000000000000, -0.000000000000000000, 1.000000000000000000 ) ) ;
#12499=DIRECTION ( 'NONE',  ( 0.000000000000000000, 0.000000000000000000, -1.000000000000000000 ) ) ;
#12501=EDGE_CURVE ( 'NONE', #15497, #7557, #1642, .T. ) ;
#12502=ADVANCED_FACE ( 'NONE', ( #18494 ), #4564, .F. ) ;
#12509=EDGE_LOOP ( 'NONE', ( #20956, #34857, #30946, #21876 ) ) ;
#12512=PLANE ( 'NONE',  #11674 ) ;
#12516=VERTEX_POINT ( 'NONE', #34132 ) ;
#12521=CARTESIAN_POINT ( 'NONE',  ( -445.9999999999999432, 104.9999999999999858, -187.0000000000000000 ) ) ;
#12522=PLANE ( 'NONE',  #10870 ) ;
#12526=PLANE ( 'NONE',  #10799 ) ;
#12531=CARTESIAN_POINT ( 'NONE',  ( -19.99999999999998934, 75.55999999999990280, -172.9900000000000091 ) ) ;
#12532=CARTESIAN_POINT ( 'NONE',  ( -442.0000000000000000, 105.0000000000000142, -101.9999999999999858 ) ) ;
#12534=EDGE_CURVE ( 'NONE', #29191, #26985, #26653, .T. ) ;
#12536=ORIENTED_EDGE ( 'NONE', *, *, #2677, .F. ) ;
#12537=DIRECTION ( 'NONE',  ( 0.000000000000000000, 1.000000000000000000, 0.000000000000000000 ) ) ;
#12539=DIRECTION ( 'NONE',  ( -1.000000000000000000, 0.000000000000000000, 0.000000000000000000 ) ) ;
#12541=ADVANCED_FACE ( 'NONE', ( #31636 ), #20449, .F. ) ;
#12542=VERTEX_POINT ( 'NONE', #6895 ) ;
#12543=CIRCLE ( 'NONE', #32412, 2.000000000000001776 ) ;
#12546=ORIENTED_EDGE ( 'NONE', *, *, #24169, .F. ) ;
#12550=ORIENTED_EDGE ( 'NONE', *, *, #7486, .F. ) ;
#12552=AXIS2_PLACEMENT_3D ( 'NONE', #32501, #8652, #16339 ) ;
#12554=EDGE_CURVE ( 'NONE', #2370, #8068, #5275, .T. ) ;
#12556=LINE ( 'NONE', #18092, #21459 ) ;
#12557=CARTESIAN_POINT ( 'NONE',  ( -500.0000000000000000, -137.0000000000000000, 162.9999999999999716 ) ) ;
#12561=CARTESIAN_POINT ( 'NONE',  ( -12.00000000000001066, -124.9999999999999432, -154.9999999999999716 ) ) ;
#12574=FACE_OUTER_BOUND ( 'NONE', #20985, .T. ) ;
#12575=LINE ( 'NONE', #1875, #5247 ) ;
#12576=ORIENTED_EDGE ( 'NONE', *, *, #12707, .F. ) ;
#12577=DIRECTION ( 'NONE',  ( 1.000000000000000000, 0.000000000000000000, 0.000000000000000000 ) ) ;
#12580=FACE_OUTER_BOUND ( 'NONE', #20078, .T. ) ;
#12581=CARTESIAN_POINT ( 'NONE',  ( -20.00000000000007461, 136.9999999999999432, -159.0000000000000000 ) ) ;
#12582=DIRECTION ( 'NONE',  ( 0.000000000000000000, -0.000000000000000000, 1.000000000000000000 ) ) ;
#12583=VECTOR ( 'NONE', #6099, 1000.000000000000000 ) ;
#12585=DIRECTION ( 'NONE',  ( 0.000000000000000000, 1.000000000000000000, -3.374343856708137958E-53 ) ) ;
#12586=DIRECTION ( 'NONE',  ( 0.000000000000000000, 0.000000000000000000, 1.000000000000000000 ) ) ;
#12587=ADVANCED_FACE ( 'NONE', ( #27007 ), #30195, .T. ) ;
#12589=ORIENTED_EDGE ( 'NONE', *, *, #1463, .T. ) ;
#12591=EDGE_CURVE ( 'NONE', #13149, #5999, #16694, .T. ) ;
#12594=CIRCLE ( 'NONE', #23380, 3.999999999999976019 ) ;
#12595=EDGE_LOOP ( 'NONE', ( #97, #21219, #1436, #313 ) ) ;
#12597=EDGE_LOOP ( 'NONE', ( #24455, #11564, #20783, #23848, #20384, #25425, #32022, #18339 ) ) ;
#12598=LINE ( 'NONE', #1385, #26389 ) ;
#12599=CARTESIAN_POINT ( 'NONE',  ( -12.00000000000001066, 134.9999999999999432, -194.9999999999999432 ) ) ;
#12600=LINE ( 'NONE', #1211, #18621 ) ;
#12611=DIRECTION ( 'NONE',  ( 1.000000000000000000, 0.000000000000000000, 0.000000000000000000 ) ) ;
#12618=DIRECTION ( 'NONE',  ( -0.000000000000000000, -1.000000000000000000, -0.000000000000000000 ) ) ;
#12621=EDGE_CURVE ( 'NONE', #842, #10465, #22019, .T. ) ;
#12627=VERTEX_POINT ( 'NONE', #32862 ) ;
#12628=MECHANICAL_DESIGN_GEOMETRIC_PRESENTATION_REPRESENTATION('',(#4077),#23408);
#12630=CARTESIAN_POINT ( 'NONE',  ( -361.0000000000000000, -125.0000000000000284, 166.9999999999999716 ) ) ;
#12631=DIRECTION ( 'NONE',  ( 0.000000000000000000, 0.000000000000000000, 1.000000000000000000 ) ) ;
#12632=CARTESIAN_POINT ( 'NONE',  ( -361.0000000000000000, -125.0000000000000284, 181.0000000000000000 ) ) ;
#12635=ORIENTED_EDGE ( 'NONE', *, *, #29374, .T. ) ;
#12636=EDGE_CURVE ( 'NONE', #19693, #4380, #29505, .T. ) ;
#12637=EDGE_CURVE ( 'NONE', #15405, #18132, #24348, .T. ) ;
#12639=VERTEX_POINT ( 'NONE', #10464 ) ;
#12642=CARTESIAN_POINT ( 'NONE',  ( -442.0000000000000000, -105.0000000000000142, 159.0000000000000000 ) ) ;
#12652=ORIENTED_EDGE ( 'NONE', *, *, #17340, .F. ) ;
#12665=DIRECTION ( 'NONE',  ( 0.000000000000000000, -1.000000000000000000, 6.123233995736766036E-17 ) ) ;
#12672=CIRCLE ( 'NONE', #13807, 3.999999999999976019 ) ;
#12678=( NAMED_UNIT ( * ) PLANE_ANGLE_UNIT ( ) SI_UNIT ( $, .RADIAN. ) );
#12683=CARTESIAN_POINT ( 'NONE',  ( -20.00000000000007461, 144.9999999999999432, -187.0000000000000000 ) ) ;
#12686=ORIENTED_EDGE ( 'NONE', *, *, #32593, .F. ) ;
#12687=ORIENTED_EDGE ( 'NONE', *, *, #24169, .T. ) ;
#12692=ORIENTED_EDGE ( 'NONE', *, *, #1128, .T. ) ;
#12695=PLANE ( 'NONE',  #4041 ) ;
#12697=VECTOR ( 'NONE', #34371, 1000.000000000000000 ) ;
#12698=ORIENTED_EDGE ( 'NONE', *, *, #33503, .F. ) ;
#12699=AXIS2_PLACEMENT_3D ( 'NONE', #11847, #12014, #31050 ) ;
#12700=CARTESIAN_POINT ( 'NONE',  ( -499.9999999999999432, 144.9999999999999716, 187.0000000000000000 ) ) ;
#12701=CARTESIAN_POINT ( 'NONE',  ( -361.0000000000000000, -125.0000000000000284, 166.9999999999999716 ) ) ;
#12706=ORIENTED_EDGE ( 'NONE', *, *, #29369, .T. ) ;
#12707=EDGE_CURVE ( 'NONE', #4626, #24390, #3489, .T. ) ;
#12709=CARTESIAN_POINT ( 'NONE',  ( -355.0000000000000000, 118.9999999999999716, 130.0000000000000000 ) ) ;
#12711=DIRECTION ( 'NONE',  ( -1.000000000000000000, 0.000000000000000000, 0.000000000000000000 ) ) ;
#12716=DIRECTION ( 'NONE',  ( 0.000000000000000000, 1.000000000000000000, 5.053935297177146739E-49 ) ) ;
#12718=VECTOR ( 'NONE', #11264, 1000.000000000000000 ) ;
#12724=VECTOR ( 'NONE', #32995, 1000.000000000000000 ) ;
#12725=ORIENTED_EDGE ( 'NONE', *, *, #11459, .T. ) ;
#12726=DIRECTION ( 'NONE',  ( -0.000000000000000000, -2.309213040847544338E-50, -1.000000000000000000 ) ) ;
#12728=EDGE_LOOP ( 'NONE', ( #1988, #26335, #33246, #6193, #4436, #21000, #3188, #25962 ) ) ;
#12732=CARTESIAN_POINT ( 'NONE',  ( -500.0000000000000000, 136.9999999999999432, -155.0000000000000000 ) ) ;
#12736=ORIENTED_EDGE ( 'NONE', *, *, #3252, .F. ) ;
#12738=DIRECTION ( 'NONE',  ( 0.000000000000000000, 1.000000000000000000, -3.374343856708137958E-53 ) ) ;
#12739=DIRECTION ( 'NONE',  ( 0.000000000000000000, -1.000000000000000000, 3.374343856708137958E-53 ) ) ;
#12742=EDGE_CURVE ( 'NONE', #25655, #2254, #25379, .T. ) ;
#12743=DIRECTION ( 'NONE',  ( 0.000000000000000000, 1.310824597558155437E-49, 1.000000000000000000 ) ) ;
#12744=CARTESIAN_POINT ( 'NONE',  ( -499.9999999999999432, 136.9999999999999432, -187.0000000000000000 ) ) ;
#12745=UNCERTAINTY_MEASURE_WITH_UNIT (LENGTH_MEASURE( 1.000000000000000082E-05 ), #33072, 'distance_accuracy_value', 'NONE');
#12748=VERTEX_POINT ( 'NONE', #11518 ) ;
#12751=AXIS2_PLACEMENT_3D ( 'NONE', #21940, #32788, #30121 ) ;
#12754=ORIENTED_EDGE ( 'NONE', *, *, #14404, .T. ) ;
#12755=EDGE_CURVE ( 'NONE', #18803, #31336, #2758, .T. ) ;
#12756=CARTESIAN_POINT ( 'NONE',  ( -410.0000000000000568, -125.0000000000000000, 162.9999999999999716 ) ) ;
#12765=ADVANCED_FACE ( 'NONE', ( #30560 ), #20063, .T. ) ;
#12766=AXIS2_PLACEMENT_3D ( 'NONE', #2249, #34833, #29838 ) ;
#12775=CIRCLE ( 'NONE', #13333, 8.000000000000007105 ) ;
#12778=ORIENTED_EDGE ( 'NONE', *, *, #15174, .T. ) ;
#12781=FACE_OUTER_BOUND ( 'NONE', #11519, .T. ) ;
#12783=DIRECTION ( 'NONE',  ( 1.000000000000000000, 0.000000000000000000, -1.848892746611746966E-32 ) ) ;
#12787=ORIENTED_EDGE ( 'NONE', *, *, #23509, .F. ) ;
#12788=FACE_OUTER_BOUND ( 'NONE', #22531, .T. ) ;
#12790=FACE_OUTER_BOUND ( 'NONE', #24394, .T. ) ;
#12795=( NAMED_UNIT ( * ) SI_UNIT ( $, .STERADIAN. ) SOLID_ANGLE_UNIT ( ) );
#12796=ORIENTED_EDGE ( 'NONE', *, *, #15077, .T. ) ;
#12801=LINE ( 'NONE', #8483, #6549 ) ;
#12802=CARTESIAN_POINT ( 'NONE',  ( -410.0000000000000568, -137.0000000000000000, 154.9999999999999716 ) ) ;
#12804=AXIS2_PLACEMENT_3D ( 'NONE', #6604, #17505, #6780 ) ;
#12805=EDGE_CURVE ( 'NONE', #29324, #14034, #9020, .T. ) ;
#12807=DIRECTION ( 'NONE',  ( -0.000000000000000000, 1.000000000000000000, -0.000000000000000000 ) ) ;
#12811=PLANE ( 'NONE',  #4186 ) ;
#12813=LINE ( 'NONE', #1588, #14508 ) ;
#12814=DIRECTION ( 'NONE',  ( -1.300283923313630633E-47, 0.000000000000000000, -1.000000000000000000 ) ) ;
#12819=AXIS2_PLACEMENT_3D ( 'NONE', #8842, #32865, #16520 ) ;
#12822=VECTOR ( 'NONE', #23456, 1000.000000000000000 ) ;
#12824=PLANE ( 'NONE',  #26373 ) ;
#12825=DIRECTION ( 'NONE',  ( 0.000000000000000000, 1.131431318426415506E-52, 1.000000000000000000 ) ) ;
#12827=ORIENTED_EDGE ( 'NONE', *, *, #16062, .F. ) ;
#12828=CIRCLE ( 'NONE', #6560, 3.999999999999976019 ) ;
#12830=LINE ( 'NONE', #9456, #21293 ) ;
#12831=DIRECTION ( 'NONE',  ( -1.232595164407830946E-32, -3.421138828918010427E-49, 1.000000000000000000 ) ) ;
#12832=ORIENTED_EDGE ( 'NONE', *, *, #1751, .F. ) ;
#12833=VERTEX_POINT ( 'NONE', #658 ) ;
#12839=AXIS2_PLACEMENT_3D ( 'NONE', #5263, #13130, #16158 ) ;
#12840=DIRECTION ( 'NONE',  ( 0.000000000000000000, 1.310824597558155437E-49, 1.000000000000000000 ) ) ;
#12841=ADVANCED_FACE ( 'NONE', ( #3140 ), #6329, .F. ) ;
#12843=ORIENTED_EDGE ( 'NONE', *, *, #28977, .T. ) ;
#12844=CARTESIAN_POINT ( 'NONE',  ( 11.99999999999999822, -115.0000000000000142, 155.0000000000000000 ) ) ;
#12845=CARTESIAN_POINT ( 'NONE',  ( -430.0000000000000000, -131.0000000000000000, 130.0000000000000000 ) ) ;
#12847=CYLINDRICAL_SURFACE ( 'NONE', #17364, 4.000000000000003553 ) ;
#12851=LINE ( 'NONE', #21023, #10506 ) ;
#12853=AXIS2_PLACEMENT_3D ( 'NONE', #13412, #24066, #28684 ) ;
#12854=EDGE_CURVE ( 'NONE', #24248, #27019, #7375, .T. ) ;
#12855=EDGE_LOOP ( 'NONE', ( #13695, #3364, #1118, #15492 ) ) ;
#12861=AXIS2_PLACEMENT_3D ( 'NONE', #20008, #30853, #7148 ) ;
#12864=ORIENTED_EDGE ( 'NONE', *, *, #4115, .F. ) ;
#12868=AXIS2_PLACEMENT_3D ( 'NONE', #3923, #26303, #19803 ) ;
#12881=FACE_OUTER_BOUND ( 'NONE', #29316, .T. ) ;
#12885=DIRECTION ( 'NONE',  ( -1.000000000000000000, -3.469446951953834515E-18, 0.000000000000000000 ) ) ;
#12886=DIRECTION ( 'NONE',  ( 1.000000000000000000, 0.000000000000000000, 0.000000000000000000 ) ) ;
#12890=CARTESIAN_POINT ( 'NONE',  ( 12.00000000000001066, -28.99999999999999645, 154.9999999999999716 ) ) ;
#12894=VECTOR ( 'NONE', #12481, 1000.000000000000000 ) ;
#12896=DIRECTION ( 'NONE',  ( 0.000000000000000000, 1.000000000000000000, 0.000000000000000000 ) ) ;
#12900=DIRECTION ( 'NONE',  ( 0.000000000000000000, -1.000000000000000000, -2.465190328815662439E-32 ) ) ;
#12903=FACE_BOUND ( 'NONE', #31352, .T. ) ;
#12906=EDGE_CURVE ( 'NONE', #28422, #20858, #2054, .T. ) ;
#12908=EDGE_LOOP ( 'NONE', ( #13992, #15521, #15968, #16779 ) ) ;
#12909=DIRECTION ( 'NONE',  ( -1.000000000000000000, 0.000000000000000000, 0.000000000000000000 ) ) ;
#12915=DIRECTION ( 'NONE',  ( 1.000000000000000000, 0.000000000000000000, -1.232595164407831220E-32 ) ) ;
#12918=ORIENTED_EDGE ( 'NONE', *, *, #26274, .T. ) ;
#12920=CARTESIAN_POINT ( 'NONE',  ( -349.0000000000000000, 124.9999999999999432, 181.0000000000000000 ) ) ;
#12922=CARTESIAN_POINT ( 'NONE',  ( -418.0000000000000000, -104.9999999999999858, -162.9999999999999716 ) ) ;
#12926=CARTESIAN_POINT ( 'NONE',  ( -19.99999999999998934, -32.99999999999997158, -175.0000000000000000 ) ) ;
#12928=CIRCLE ( 'NONE', #32796, 7.999999999999979572 ) ;
#12931=DIRECTION ( 'NONE',  ( 1.000000000000000000, 0.000000000000000000, 0.000000000000000000 ) ) ;
#12932=ORIENTED_EDGE ( 'NONE', *, *, #30322, .T. ) ;
#12935=CARTESIAN_POINT ( 'NONE',  ( -442.0000000000000000, 105.0000000000000142, 159.0000000000000000 ) ) ;
#12936=VERTEX_POINT ( 'NONE', #26087 ) ;
#12938=CARTESIAN_POINT ( 'NONE',  ( -15.99999999999998579, -32.99999999999997158, -154.9999999999999716 ) ) ;
#12939=AXIS2_PLACEMENT_3D ( 'NONE', #5185, #26911, #15544 ) ;
#12942=DIRECTION ( 'NONE',  ( 1.000000000000000000, 0.000000000000000000, 0.000000000000000000 ) ) ;
#12945=ORIENTED_EDGE ( 'NONE', *, *, #4431, .T. ) ;
#12948=ADVANCED_FACE ( 'NONE', ( #23768 ), #10066, .F. ) ;
#12954=DIRECTION ( 'NONE',  ( -2.891205793294674875E-16, -7.888609052210118054E-31, -1.000000000000000000 ) ) ;
#12958=ORIENTED_EDGE ( 'NONE', *, *, #7333, .T. ) ;
#12959=ORIENTED_EDGE ( 'NONE', *, *, #22190, .T. ) ;
#12961=DIRECTION ( 'NONE',  ( -2.736911063134582149E-48, 7.888609052210118054E-31, 1.000000000000000000 ) ) ;
#12963=CIRCLE ( 'NONE', #27730, 4.750000000000004441 ) ;
#12966=LINE ( 'NONE', #21318, #24263 ) ;
#12975=LINE ( 'NONE', #17801, #24531 ) ;
#12979=EDGE_CURVE ( 'NONE', #10757, #4201, #15073, .T. ) ;
#12982=CARTESIAN_POINT ( 'NONE',  ( -15.99999999999998579, 4.559999999999908127, 172.9900000000000091 ) ) ;
#12983=EDGE_CURVE ( 'NONE', #31630, #2660, #17580, .T. ) ;
#12986=VERTEX_POINT ( 'NONE', #23084 ) ;
#12991=DIRECTION ( 'NONE',  ( 0.000000000000000000, 5.053935297177146739E-49, 1.000000000000000000 ) ) ;
#12996=LINE ( 'NONE', #10495, #26152 ) ;
#13003=ADVANCED_FACE ( 'NONE', ( #18962 ), #5410, .F. ) ;
#13006=AXIS2_PLACEMENT_3D ( 'NONE', #9967, #34527, #4961 ) ;
#13007=EDGE_LOOP ( 'NONE', ( #1034, #11033, #5520, #4438 ) ) ;
#13008=ORIENTED_EDGE ( 'NONE', *, *, #12906, .F. ) ;
#13010=ORIENTED_EDGE ( 'NONE', *, *, #19064, .F. ) ;
#13011=DIRECTION ( 'NONE',  ( -1.000000000000000000, 0.000000000000000000, -1.300283923313630633E-47 ) ) ;
#13015=CARTESIAN_POINT ( 'NONE',  ( -15.99999999999998579, 112.9999999999999574, -175.0000000000000284 ) ) ;
#13019=ORIENTED_EDGE ( 'NONE', *, *, #12423, .T. ) ;
#13022=DIRECTION ( 'NONE',  ( 0.000000000000000000, -1.000000000000000000, -1.224646799147353207E-16 ) ) ;
#13023=VECTOR ( 'NONE', #14732, 1000.000000000000000 ) ;
#13025=DIRECTION ( 'NONE',  ( 0.000000000000000000, 1.000000000000000000, -3.374343856708137958E-53 ) ) ;
#13026=DIRECTION ( 'NONE',  ( 0.000000000000000000, 1.000000000000000000, 5.145227585319922065E-49 ) ) ;
#13031=ORIENTED_EDGE ( 'NONE', *, *, #10213, .F. ) ;
#13034=VECTOR ( 'NONE', #20050, 1000.000000000000000 ) ;
#13035=ADVANCED_FACE ( 'NONE', ( #18445 ), #13271, .F. ) ;
#13040=EDGE_LOOP ( 'NONE', ( #22858, #13505, #21745, #17163 ) ) ;
#13041=DIRECTION ( 'NONE',  ( -1.000000000000000000, 0.000000000000000000, 0.000000000000000000 ) ) ;
#13045=EDGE_LOOP ( 'NONE', ( #11355, #32619, #21428, #10856 ) ) ;
#13047=CARTESIAN_POINT ( 'NONE',  ( 15.99999999999998579, 75.55999999999990280, -172.9900000000000091 ) ) ;
#13049=PLANE ( 'NONE',  #23835 ) ;
#13053=ORIENTED_EDGE ( 'NONE', *, *, #20298, .T. ) ;
#13054=LINE ( 'NONE', #13404, #33963 ) ;
#13055=DIRECTION ( 'NONE',  ( 1.000000000000000000, 0.000000000000000000, 0.000000000000000000 ) ) ;
#13058=EDGE_CURVE ( 'NONE', #18790, #26143, #10600, .T. ) ;
#13059=CARTESIAN_POINT ( 'NONE',  ( -347.0000000000000000, -125.0000000000000284, 114.0000000000000000 ) ) ;
#13062=DIRECTION ( 'NONE',  ( 0.000000000000000000, 1.000000000000000000, 1.224646799147353207E-16 ) ) ;
#13063=ADVANCED_FACE ( 'NONE', ( #16122 ), #15775, .F. ) ;
#13066=ORIENTED_EDGE ( 'NONE', *, *, #18944, .F. ) ;
#13067=CARTESIAN_POINT ( 'NONE',  ( -442.0000000000000000, 124.9999999999999574, -187.0000000000000000 ) ) ;
#13069=CARTESIAN_POINT ( 'NONE',  ( -355.0000000000000000, 130.9999999999999716, 111.9999999999999858 ) ) ;
#13072=ORIENTED_EDGE ( 'NONE', *, *, #16795, .T. ) ;
#13073=DIRECTION ( 'NONE',  ( 1.000000000000000000, 0.000000000000000000, 0.000000000000000000 ) ) ;
#13074=VERTEX_POINT ( 'NONE', #81 ) ;
#13079=CARTESIAN_POINT ( 'NONE',  ( -442.0000000000000000, -105.0000000000000142, 162.9999999999999716 ) ) ;
#13081=ORIENTED_EDGE ( 'NONE', *, *, #13239, .F. ) ;
#13082=DIRECTION ( 'NONE',  ( 1.000000000000000000, 3.040835319149746090E-31, 1.232595164407830946E-32 ) ) ;
#13083=DIRECTION ( 'NONE',  ( 0.000000000000000000, -1.000000000000000000, 0.000000000000000000 ) ) ;
#13085=ORIENTED_EDGE ( 'NONE', *, *, #12755, .F. ) ;
#13087=CARTESIAN_POINT ( 'NONE',  ( 19.99999999999998934, 144.9999999999999716, 162.9999999999999716 ) ) ;
#13088=CYLINDRICAL_SURFACE ( 'NONE', #18629, 4.750000000000004441 ) ;
#13089=CARTESIAN_POINT ( 'NONE',  ( -19.99999999999998934, 134.9999999999998863, 162.9999999999999716 ) ) ;
#13090=DIRECTION ( 'NONE',  ( 0.000000000000000000, 0.000000000000000000, -1.000000000000000000 ) ) ;
#13091=CARTESIAN_POINT ( 'NONE',  ( -442.0000000000000000, -105.0000000000000142, 132.0000000000000000 ) ) ;
#13092=ORIENTED_EDGE ( 'NONE', *, *, #7857, .T. ) ;
#13095=FACE_OUTER_BOUND ( 'NONE', #18643, .T. ) ;
#13096=ORIENTED_EDGE ( 'NONE', *, *, #11055, .T. ) ;
#13097=FACE_OUTER_BOUND ( 'NONE', #28017, .T. ) ;
#13099=CARTESIAN_POINT ( 'NONE',  ( 11.99999999999999645, 144.9999999999999716, -175.0000000000000284 ) ) ;
#13100=ORIENTED_EDGE ( 'NONE', *, *, #32383, .T. ) ;
#13104=ADVANCED_FACE ( 'NONE', ( #13095 ), #18619, .T. ) ;
#13105=CARTESIAN_POINT ( 'NONE',  ( -499.9999999999999432, -113.0000000000000000, -155.0000000000000000 ) ) ;
#13108=DIRECTION ( 'NONE',  ( 0.000000000000000000, 1.000000000000000000, -6.842277657836020854E-49 ) ) ;
#13109=DIRECTION ( 'NONE',  ( 0.000000000000000000, 1.310824597558155437E-49, 1.000000000000000000 ) ) ;
#13113=ADVANCED_FACE ( 'NONE', ( #6465 ), #17366, .F. ) ;
#13115=ORIENTED_EDGE ( 'NONE', *, *, #24288, .F. ) ;
#13118=EDGE_LOOP ( 'NONE', ( #11501, #5227, #4835, #6720 ) ) ;
#13121=FACE_OUTER_BOUND ( 'NONE', #2389, .T. ) ;
#13126=ORIENTED_EDGE ( 'NONE', *, *, #27672, .F. ) ;
#13127=ORIENTED_EDGE ( 'NONE', *, *, #32454, .F. ) ;
#13128=AXIS2_PLACEMENT_3D ( 'NONE', #4197, #15608, #1192 ) ;
#13130=DIRECTION ( 'NONE',  ( -3.469446951953832974E-18, -1.000000000000000000, -7.888609052210116302E-31 ) ) ;
#13133=CARTESIAN_POINT ( 'NONE',  ( 15.99999999999998579, 75.55999999999990280, -168.2400000000000091 ) ) ;
#13135=FACE_OUTER_BOUND ( 'NONE', #20558, .T. ) ;
#13136=CARTESIAN_POINT ( 'NONE',  ( 15.99999999999998579, -32.99999999999997158, -175.0000000000000000 ) ) ;
#13137=DIRECTION ( 'NONE',  ( 0.000000000000000000, 2.309213040847544338E-50, 1.000000000000000000 ) ) ;
#13139=AXIS2_PLACEMENT_3D ( 'NONE', #19885, #25377, #3487 ) ;
#13140=EDGE_CURVE ( 'NONE', #24525, #28865, #17608, .T. ) ;
#13145=DIRECTION ( 'NONE',  ( 1.000000000000000000, 3.469446951953834515E-18, 0.000000000000000000 ) ) ;
#13149=VERTEX_POINT ( 'NONE', #11300 ) ;
#13150=CYLINDRICAL_SURFACE ( 'NONE', #14918, 7.999999999999979572 ) ;
#13157=FACE_OUTER_BOUND ( 'NONE', #5922, .T. ) ;
#13158=VECTOR ( 'NONE', #18191, 1000.000000000000000 ) ;
#13163=CARTESIAN_POINT ( 'NONE',  ( 18.92820323027550344, -124.9999999999999432, -158.9999999999999716 ) ) ;
#13164=AXIS2_PLACEMENT_3D ( 'NONE', #34041, #1646, #34570 ) ;
#13165=CARTESIAN_POINT ( 'NONE',  ( -500.0000000000000000, -141.0000000000000000, 162.9999999999999716 ) ) ;
#13167=CYLINDRICAL_SURFACE ( 'NONE', #25572, 8.000000000000007105 ) ;
#13170=LINE ( 'NONE', #21529, #23778 ) ;
#13172=DIRECTION ( 'NONE',  ( 1.000000000000000000, 0.000000000000000000, 0.000000000000000000 ) ) ;
#13175=VERTEX_POINT ( 'NONE', #27659 ) ;
#13176=DIRECTION ( 'NONE',  ( 0.000000000000000000, 0.000000000000000000, 1.000000000000000000 ) ) ;
#13177=VECTOR ( 'NONE', #14211, 1000.000000000000000 ) ;
#13179=ORIENTED_EDGE ( 'NONE', *, *, #17273, .T. ) ;
#13184=LINE ( 'NONE', #29193, #5165 ) ;
#13189=ORIENTED_EDGE ( 'NONE', *, *, #17932, .T. ) ;
#13190=EDGE_CURVE ( 'NONE', #10395, #21456, #3619, .T. ) ;
#13195=CARTESIAN_POINT ( 'NONE',  ( -418.0000000000000000, -105.0000000000000142, -155.0000000000000000 ) ) ;
#13197=CARTESIAN_POINT ( 'NONE',  ( -445.9999999999999432, -105.0000000000000142, -77.99999999999997158 ) ) ;
#13199=DIRECTION ( 'NONE',  ( -1.000000000000000000, 0.000000000000000000, 0.000000000000000000 ) ) ;
#13201=AXIS2_PLACEMENT_3D ( 'NONE', #33983, #9438, #6572 ) ;
#13209=VECTOR ( 'NONE', #29686, 1000.000000000000000 ) ;
#13210=ORIENTED_EDGE ( 'NONE', *, *, #34109, .T. ) ;
#13211=ORIENTED_EDGE ( 'NONE', *, *, #17782, .F. ) ;
#13220=CLOSED_SHELL ( 'NONE', ( #31020, #31771, #4026, #27427, #26992, #25080, #20239, #18103, #12765, #857, #17289, #26550, #7582, #24003, #11320, #20974, #15491, #18656, #24778, #3115, #17396, #6164, #19459, #27512, #4718, #9088, #22555 ) ) ;
#13221=CARTESIAN_POINT ( 'NONE',  ( -414.0000000000000568, -104.9999999999999858, -162.9999999999999716 ) ) ;
#13225=DIRECTION ( 'NONE',  ( 1.000000000000000000, 0.000000000000000000, 0.000000000000000000 ) ) ;
#13228=DIRECTION ( 'NONE',  ( 0.000000000000000000, 7.888609052210118054E-31, 1.000000000000000000 ) ) ;
#13230=VECTOR ( 'NONE', #24071, 1000.000000000000000 ) ;
#13231=AXIS2_PLACEMENT_3D ( 'NONE', #4191, #1539, #30911 ) ;
#13234=CARTESIAN_POINT ( 'NONE',  ( -418.0000000000000000, 109.0000000000000142, 154.9999999999999716 ) ) ;
#13237=LINE ( 'NONE', #31897, #18469 ) ;
#13239=EDGE_CURVE ( 'NONE', #22194, #33693, #30330, .T. ) ;
#13240=EDGE_CURVE ( 'NONE', #17691, #19198, #31775, .T. ) ;
#13242=ORIENTED_EDGE ( 'NONE', *, *, #14879, .T. ) ;
#13244=LINE ( 'NONE', #26928, #25950 ) ;
#13245=ORIENTED_EDGE ( 'NONE', *, *, #24251, .T. ) ;
#13247=ORIENTED_EDGE ( 'NONE', *, *, #22419, .T. ) ;
#13248=ADVANCED_FACE ( 'NONE', ( #33888, #6990 ), #23545, .F. ) ;
#13253=EDGE_LOOP ( 'NONE', ( #4347, #16089, #16877, #11176 ) ) ;
#13259=DIRECTION ( 'NONE',  ( 0.000000000000000000, 0.000000000000000000, 1.000000000000000000 ) ) ;
#13263=ORIENTED_EDGE ( 'NONE', *, *, #24443, .T. ) ;
#13264=CARTESIAN_POINT ( 'NONE',  ( -365.0000000000000000, 132.9999999999999716, 113.9999999999999858 ) ) ;
#13271=PLANE ( 'NONE',  #34632 ) ;
#13272=ORIENTED_EDGE ( 'NONE', *, *, #25574, .F. ) ;
#13273=DIRECTION ( 'NONE',  ( -0.000000000000000000, 1.000000000000000000, 0.000000000000000000 ) ) ;
#13274=DIRECTION ( 'NONE',  ( -0.000000000000000000, 0.000000000000000000, 1.000000000000000000 ) ) ;
#13275=CARTESIAN_POINT ( 'NONE',  ( 11.99999999999999645, -141.0000000000000000, 174.9999999999999432 ) ) ;
#13276=VERTEX_POINT ( 'NONE', #28714 ) ;
#13278=LINE ( 'NONE', #34810, #29709 ) ;
#13280=AXIS2_PLACEMENT_3D ( 'NONE', #1543, #841, #9385 ) ;
#13281=ADVANCED_FACE ( 'NONE', ( #4315 ), #12526, .F. ) ;
#13282=ADVANCED_FACE ( 'NONE', ( #31556 ), #20367, .T. ) ;
#13283=AXIS2_PLACEMENT_3D ( 'NONE', #7295, #13022, #1451 ) ;
#13284=DIRECTION ( 'NONE',  ( 0.000000000000000000, -1.000000000000000000, -1.224646799147353207E-16 ) ) ;
#13290=DIRECTION ( 'NONE',  ( -0.000000000000000000, -1.000000000000000000, -0.000000000000000000 ) ) ;
#13293=EDGE_CURVE ( 'NONE', #27359, #11247, #4141, .T. ) ;
#13298=ORIENTED_EDGE ( 'NONE', *, *, #18967, .F. ) ;
#13301=EDGE_CURVE ( 'NONE', #8875, #29676, #25874, .T. ) ;
#13303=EDGE_CURVE ( 'NONE', #34313, #13897, #34232, .T. ) ;
#13304=AXIS2_PLACEMENT_3D ( 'NONE', #10380, #7517, #21236 ) ;
#13311=ORIENTED_EDGE ( 'NONE', *, *, #16050, .F. ) ;
#13312=DIRECTION ( 'NONE',  ( 1.000000000000000000, 0.000000000000000000, -1.232595164407831220E-32 ) ) ;
#13313=LINE ( 'NONE', #5448, #6082 ) ;
#13314=ADVANCED_FACE ( 'NONE', ( #9669 ), #9843, .F. ) ;
#13320=ORIENTED_EDGE ( 'NONE', *, *, #25602, .F. ) ;
#13322=DIRECTION ( 'NONE',  ( 1.000000000000000000, 0.000000000000000000, 0.000000000000000000 ) ) ;
#13326=CARTESIAN_POINT ( 'NONE',  ( -442.0000000000000000, 141.0000000000000000, -175.0000000000000000 ) ) ;
#13330=CYLINDRICAL_SURFACE ( 'NONE', #17312, 7.999999999999979572 ) ;
#13332=ORIENTED_EDGE ( 'NONE', *, *, #34592, .T. ) ;
#13333=AXIS2_PLACEMENT_3D ( 'NONE', #8943, #6609, #19815 ) ;
#13337=AXIS2_PLACEMENT_3D ( 'NONE', #21526, #29360, #15489 ) ;
#13338=VERTEX_POINT ( 'NONE', #28885 ) ;
#13342=FACE_OUTER_BOUND ( 'NONE', #34635, .T. ) ;
#13348=AXIS2_PLACEMENT_3D ( 'NONE', #5563, #8956, #19830 ) ;
#13352=CARTESIAN_POINT ( 'NONE',  ( -442.0000000000000000, -109.0000000000000142, -174.9999999999999716 ) ) ;
#13354=LINE ( 'NONE', #24188, #16201 ) ;
#13356=CIRCLE ( 'NONE', #17917, 3.999999999999976019 ) ;
#13361=VERTEX_POINT ( 'NONE', #9400 ) ;
#13364=EDGE_LOOP ( 'NONE', ( #21199, #14823, #6385, #12754 ) ) ;
#13365=DIRECTION ( 'NONE',  ( 0.000000000000000000, 1.000000000000000000, 5.145227585319922065E-49 ) ) ;
#13366=CARTESIAN_POINT ( 'NONE',  ( -20.00000000000007461, 112.9999999999999574, -187.0000000000000000 ) ) ;
#13367=ORIENTED_EDGE ( 'NONE', *, *, #1342, .F. ) ;
#13369=CARTESIAN_POINT ( 'NONE',  ( -349.0000000000000000, -135.0000000000000000, 113.9999999999999858 ) ) ;
#13371=CARTESIAN_POINT ( 'NONE',  ( 19.99999999999998224, 144.9999999999999716, -162.9999999999999432 ) ) ;
#13372=CIRCLE ( 'NONE', #25854, 7.999999999999992895 ) ;
#13373=CARTESIAN_POINT ( 'NONE',  ( 19.99999999999998934, 75.55999999999990280, -168.2400000000000091 ) ) ;
#13375=CARTESIAN_POINT ( 'NONE',  ( 11.99999999999999645, -55.00000000000000711, 162.9999999999999716 ) ) ;
#13382=AXIS2_PLACEMENT_3D ( 'NONE', #618, #30699, #28382 ) ;
#13383=ORIENTED_EDGE ( 'NONE', *, *, #11222, .F. ) ;
#13384=ADVANCED_FACE ( 'NONE', ( #14576 ), #27898, .T. ) ;
#13389=PRODUCT_DEFINITION ( 'UNKNOWN', '', #12196, #27440 ) ;
#13396=VERTEX_POINT ( 'NONE', #14217 ) ;
#13404=CARTESIAN_POINT ( 'NONE',  ( -12.00000000000001066, 124.9999999999999716, 190.9999999999999716 ) ) ;
#13409=CARTESIAN_POINT ( 'NONE',  ( 11.99999999999995559, -134.9999999999999716, -162.9999999999999432 ) ) ;
#13412=CARTESIAN_POINT ( 'NONE',  ( -11.99999999999998224, -134.9999999999999716, 162.9999999999999716 ) ) ;
#13414=ORIENTED_EDGE ( 'NONE', *, *, #14391, .T. ) ;
#13417=CARTESIAN_POINT ( 'NONE',  ( -500.0000000000000000, -105.0000000000000142, 187.0000000000000000 ) ) ;
#13420=CARTESIAN_POINT ( 'NONE',  ( -12.00000000000001066, -24.99999999999999289, -175.0000000000000000 ) ) ;
#13430=AXIS2_PLACEMENT_3D ( 'NONE', #24904, #19592, #30437 ) ;
#13431=LINE ( 'NONE', #27473, #29434 ) ;
#13435=ORIENTED_EDGE ( 'NONE', *, *, #3240, .T. ) ;
#13440=LINE ( 'NONE', #11124, #14289 ) ;
#13442=AXIS2_PLACEMENT_3D ( 'NONE', #22847, #33694, #31035 ) ;
#13443=DIRECTION ( 'NONE',  ( 0.000000000000000000, 0.000000000000000000, 1.000000000000000000 ) ) ;
#13446=DIRECTION ( 'NONE',  ( 8.433758354584418579E-81, -1.000000000000000000, -3.421138828918010427E-49 ) ) ;
#13447=CARTESIAN_POINT ( 'NONE',  ( -349.0000000000000000, 134.9999999999999716, 128.0000000000000000 ) ) ;
#13452=CARTESIAN_POINT ( 'NONE',  ( 19.99999999999996092, -134.9999999999999716, 162.9999999999999716 ) ) ;
#13453=ORIENTED_EDGE ( 'NONE', *, *, #31449, .T. ) ;
#13454=CARTESIAN_POINT ( 'NONE',  ( 19.99999999999998224, -55.00000000000000711, -158.9999999999999716 ) ) ;
#13456=ORIENTED_EDGE ( 'NONE', *, *, #4477, .F. ) ;
#13461=VECTOR ( 'NONE', #4744, 1000.000000000000000 ) ;
#13467=DIRECTION ( 'NONE',  ( 1.000000000000000000, 0.000000000000000000, 1.300283923313630633E-47 ) ) ;
#13474=VERTEX_POINT ( 'NONE', #9215 ) ;
#13477=AXIS2_PLACEMENT_3D ( 'NONE', #26460, #1900, #29131 ) ;
#13480=DIRECTION ( 'NONE',  ( -0.000000000000000000, 1.000000000000000000, -0.000000000000000000 ) ) ;
#13481=CARTESIAN_POINT ( 'NONE',  ( 12.00000000000001066, -134.9999999999999716, 155.0000000000000000 ) ) ;
#13485=AXIS2_PLACEMENT_3D ( 'NONE', #25604, #22947, #28457 ) ;
#13486=FACE_BOUND ( 'NONE', #12294, .T. ) ;
#13487=CYLINDRICAL_SURFACE ( 'NONE', #14913, 7.999999999999979572 ) ;
#13489=FACE_OUTER_BOUND ( 'NONE', #2869, .T. ) ;
#13491=AXIS2_PLACEMENT_3D ( 'NONE', #3963, #10020, #31553 ) ;
#13493=EDGE_LOOP ( 'NONE', ( #10927, #31887, #25141, #12339 ) ) ;
#13495=EDGE_CURVE ( 'NONE', #21641, #143, #30402, .T. ) ;
#13498=EDGE_CURVE ( 'NONE', #15995, #10280, #27726, .T. ) ;
#13499=ORIENTED_EDGE ( 'NONE', *, *, #5372, .F. ) ;
#13500=CYLINDRICAL_SURFACE ( 'NONE', #17740, 7.999999999999979572 ) ;
#13504=ORIENTED_EDGE ( 'NONE', *, *, #1438, .F. ) ;
#13505=ORIENTED_EDGE ( 'NONE', *, *, #12554, .T. ) ;
#13506=VECTOR ( 'NONE', #16857, 1000.000000000000000 ) ;
#13512=AXIS2_PLACEMENT_3D ( 'NONE', #8925, #19627, #6235 ) ;
#13517=EDGE_CURVE ( 'NONE', #9925, #11163, #20948, .T. ) ;
#13518=VERTEX_POINT ( 'NONE', #10260 ) ;
#13519=EDGE_CURVE ( 'NONE', #18998, #13672, #9073, .T. ) ;
#13520=VERTEX_POINT ( 'NONE', #7227 ) ;
#13526=ORIENTED_EDGE ( 'NONE', *, *, #5604, .T. ) ;
#13527=CARTESIAN_POINT ( 'NONE',  ( -12.00000000000001066, 112.9999999999999574, 155.0000000000000000 ) ) ;
#13530=LINE ( 'NONE', #24366, #16588 ) ;
#13533=CARTESIAN_POINT ( 'NONE',  ( -418.0000000000000000, -105.0000000000000142, 107.9999999999999858 ) ) ;
#13535=DIRECTION ( 'NONE',  ( 1.000000000000000000, 3.469446951953834515E-18, 0.000000000000000000 ) ) ;
#13538=DIRECTION ( 'NONE',  ( 0.000000000000000000, 1.000000000000000000, 5.053935297177146739E-49 ) ) ;
#13540=EDGE_CURVE ( 'NONE', #763, #27942, #28781, .T. ) ;
#13547=DIRECTION ( 'NONE',  ( 1.000000000000000000, 0.000000000000000000, -1.232595164407831220E-32 ) ) ;
#13549=AXIS2_PLACEMENT_3D ( 'NONE', #16601, #6558, #9060 ) ;
#13554=ORIENTED_EDGE ( 'NONE', *, *, #32660, .F. ) ;
#13555=ORIENTED_EDGE ( 'NONE', *, *, #26917, .F. ) ;
#13557=CIRCLE ( 'NONE', #10143, 7.999999999999979572 ) ;
#13572=LINE ( 'NONE', #2179, #10858 ) ;
#13576=CARTESIAN_POINT ( 'NONE',  ( -418.0000000000000000, -104.9999999999999716, -187.0000000000000000 ) ) ;
#13577=CARTESIAN_POINT ( 'NONE',  ( -499.9999999999999432, 112.9999999999999574, -190.9999999999999716 ) ) ;
#13578=FACE_OUTER_BOUND ( 'NONE', #10190, .T. ) ;
#13583=EDGE_CURVE ( 'NONE', #14377, #7094, #5600, .T. ) ;
#13585=EDGE_CURVE ( 'NONE', #15904, #22409, #5254, .T. ) ;
#13589=CARTESIAN_POINT ( 'NONE',  ( -441.9999999999999432, -105.0000000000000142, -73.99999999999998579 ) ) ;
#13591=CYLINDRICAL_SURFACE ( 'NONE', #24232, 3.999999999999976019 ) ;
#13592=ORIENTED_EDGE ( 'NONE', *, *, #28076, .F. ) ;
#13597=VERTEX_POINT ( 'NONE', #29658 ) ;
#13598=DIRECTION ( 'NONE',  ( 0.000000000000000000, -1.000000000000000000, -2.465190328815662439E-32 ) ) ;
#13601=CARTESIAN_POINT ( 'NONE',  ( -418.0000000000000000, -105.0000000000000142, -101.9999999999999858 ) ) ;
#13603=CARTESIAN_POINT ( 'NONE',  ( 11.99999999999999645, 144.9999999999999716, -186.9999999999999716 ) ) ;
#13606=VERTEX_POINT ( 'NONE', #16146 ) ;
#13611=VERTEX_POINT ( 'NONE', #19336 ) ;
#13616=PLANE ( 'NONE',  #9955 ) ;
#13620=VECTOR ( 'NONE', #29488, 1000.000000000000000 ) ;
#13621=CARTESIAN_POINT ( 'NONE',  ( -12.00000000000001066, 124.9999999999999716, 155.0000000000000000 ) ) ;
#13624=CARTESIAN_POINT ( 'NONE',  ( -418.0000000000000000, -137.0000000000000000, -175.0000000000000000 ) ) ;
#13630=VERTEX_POINT ( 'NONE', #13814 ) ;
#13635=ORIENTED_EDGE ( 'NONE', *, *, #9437, .T. ) ;
#13638=ORIENTED_EDGE ( 'NONE', *, *, #17021, .T. ) ;
#13639=ORIENTED_EDGE ( 'NONE', *, *, #5961, .F. ) ;
#13640=CARTESIAN_POINT ( 'NONE',  ( -499.9999999999999432, -137.0000000000000000, -159.0000000000000000 ) ) ;
#13648=DIRECTION ( 'NONE',  ( -5.546364386991661285E-52, 0.000000000000000000, 1.000000000000000000 ) ) ;
#13650=DIRECTION ( 'NONE',  ( -1.000000000000000000, 0.000000000000000000, 0.000000000000000000 ) ) ;
#13652=DIRECTION ( 'NONE',  ( -1.000000000000000000, 0.000000000000000000, 0.000000000000000000 ) ) ;
#13654=ORIENTED_EDGE ( 'NONE', *, *, #31961, .T. ) ;
#13655=DIRECTION ( 'NONE',  ( 0.000000000000000000, 1.000000000000000000, 1.224646799147353207E-16 ) ) ;
#13659=CARTESIAN_POINT ( 'NONE',  ( -499.9999999999999432, -113.0000000000000000, -159.0000000000000000 ) ) ;
#13663=EDGE_CURVE ( 'NONE', #33397, #4380, #20171, .T. ) ;
#13664=CYLINDRICAL_SURFACE ( 'NONE', #6475, 3.999999999999976019 ) ;
#13665=AXIS2_PLACEMENT_3D ( 'NONE', #27949, #14797, #1427 ) ;
#13666=VERTEX_POINT ( 'NONE', #28524 ) ;
#13667=ADVANCED_FACE ( 'NONE', ( #20507 ), #34206, .F. ) ;
#13672=VERTEX_POINT ( 'NONE', #31021 ) ;
#13687=CIRCLE ( 'NONE', #2315, 7.999999999999979572 ) ;
#13688=LINE ( 'NONE', #13352, #32231 ) ;
#13690=AXIS2_PLACEMENT_3D ( 'NONE', #15448, #12783, #18482 ) ;
#13691=EDGE_CURVE ( 'NONE', #34601, #13338, #19320, .T. ) ;
#13692=CYLINDRICAL_SURFACE ( 'NONE', #26951, 7.999999999999979572 ) ;
#13695=ORIENTED_EDGE ( 'NONE', *, *, #15033, .F. ) ;
#13696=DIRECTION ( 'NONE',  ( 1.000000000000000000, 3.469446951953834515E-18, 0.000000000000000000 ) ) ;
#13701=ORIENTED_EDGE ( 'NONE', *, *, #19414, .F. ) ;
#13702=CARTESIAN_POINT ( 'NONE',  ( 15.99999999999998579, 75.55999999999990280, -177.7400000000000091 ) ) ;
#13704=VECTOR ( 'NONE', #18118, 1000.000000000000000 ) ;
#13708=CYLINDRICAL_SURFACE ( 'NONE', #12051, 3.999999999999976019 ) ;
#13712=EDGE_CURVE ( 'NONE', #4380, #24256, #30353, .T. ) ;
#13714=CYLINDRICAL_SURFACE ( 'NONE', #3120, 2.000000000000001776 ) ;
#13717=EDGE_CURVE ( 'NONE', #26511, #7371, #32379, .T. ) ;
#13722=ORIENTED_EDGE ( 'NONE', *, *, #19861, .F. ) ;
#13726=VECTOR ( 'NONE', #18889, 1000.000000000000000 ) ;
#13727=ORIENTED_EDGE ( 'NONE', *, *, #3932, .F. ) ;
#13729=AXIS2_PLACEMENT_3D ( 'NONE', #4447, #29204, #4797 ) ;
#13730=CARTESIAN_POINT ( 'NONE',  ( -414.0000000000000568, 113.0000000000000000, 154.9999999999999716 ) ) ;
#13734=DIRECTION ( 'NONE',  ( 0.000000000000000000, 0.000000000000000000, -1.000000000000000000 ) ) ;
#13736=ORIENTED_EDGE ( 'NONE', *, *, #2763, .F. ) ;
#13743=CARTESIAN_POINT ( 'NONE',  ( -430.0000000000000000, 114.9999999999999574, 113.9999999999999858 ) ) ;
#13745=AXIS2_PLACEMENT_3D ( 'NONE', #521, #166, #27384 ) ;
#13746=FACE_OUTER_BOUND ( 'NONE', #15572, .T. ) ;
#13747=CARTESIAN_POINT ( 'NONE',  ( -500.0000000000000000, -145.0000000000000000, 187.0000000000000000 ) ) ;
#13751=EDGE_CURVE ( 'NONE', #34323, #11236, #16858, .T. ) ;
#13755=CARTESIAN_POINT ( 'NONE',  ( -418.0000000000000000, -137.0000000000000000, 154.9999999999999716 ) ) ;
#13756=AXIS2_PLACEMENT_3D ( 'NONE', #26139, #28118, #34151 ) ;
#13757=DIRECTION ( 'NONE',  ( -1.300283923313630633E-47, 0.000000000000000000, -1.000000000000000000 ) ) ;
#13759=VECTOR ( 'NONE', #6690, 1000.000000000000000 ) ;
#13760=AXIS2_PLACEMENT_3D ( 'NONE', #4715, #18124, #4020 ) ;
#13762=AXIS2_PLACEMENT_3D ( 'NONE', #15821, #23809, #1739 ) ;
#13764=DIRECTION ( 'NONE',  ( -1.000000000000000000, 0.000000000000000000, -5.546364386991661285E-52 ) ) ;
#13766=FACE_OUTER_BOUND ( 'NONE', #1353, .T. ) ;
#13769=DIRECTION ( 'NONE',  ( 1.000000000000000000, 0.000000000000000000, 0.000000000000000000 ) ) ;
#13771=VERTEX_POINT ( 'NONE', #26718 ) ;
#13773=ORIENTED_EDGE ( 'NONE', *, *, #26319, .T. ) ;
#13778=CIRCLE ( 'NONE', #26268, 3.999999999999976019 ) ;
#13780=DIRECTION ( 'NONE',  ( 0.000000000000000000, 1.310824597558155437E-49, 1.000000000000000000 ) ) ;
#13781=AXIS2_PLACEMENT_3D ( 'NONE', #26963, #5582, #19318 ) ;
#13783=ORIENTED_EDGE ( 'NONE', *, *, #34069, .T. ) ;
#13784=VERTEX_POINT ( 'NONE', #12683 ) ;
#13786=DIRECTION ( 'NONE',  ( 0.000000000000000000, 1.131431318426415506E-52, 1.000000000000000000 ) ) ;
#13787=DIRECTION ( 'NONE',  ( 1.000000000000000000, 0.000000000000000000, 0.000000000000000000 ) ) ;
#13789=CARTESIAN_POINT ( 'NONE',  ( -12.00000000000001066, 134.9999999999999432, -186.9999999999999716 ) ) ;
#13791=CARTESIAN_POINT ( 'NONE',  ( -12.00000000000001066, 104.9999999999999858, -175.0000000000000284 ) ) ;
#13799=DIRECTION ( 'NONE',  ( -3.040835319149746090E-31, -1.000000000000000000, 0.000000000000000000 ) ) ;
#13800=ORIENTED_EDGE ( 'NONE', *, *, #924, .F. ) ;
#13801=CARTESIAN_POINT ( 'NONE',  ( -442.0000000000000000, 105.0000000000000142, -105.9999999999999574 ) ) ;
#13807=AXIS2_PLACEMENT_3D ( 'NONE', #24420, #18593, #10383 ) ;
#13813=CARTESIAN_POINT ( 'NONE',  ( 19.99999999999998224, 144.9999999999999147, 162.9999999999999716 ) ) ;
#13814=CARTESIAN_POINT ( 'NONE',  ( -418.0000000000000000, 109.0000000000000142, 154.9999999999999716 ) ) ;
#13815=EDGE_LOOP ( 'NONE', ( #15043, #16771, #7709, #16763 ) ) ;
#13817=DIRECTION ( 'NONE',  ( 0.000000000000000000, 0.000000000000000000, 1.000000000000000000 ) ) ;
#13821=AXIS2_PLACEMENT_3D ( 'NONE', #5020, #4658, #23374 ) ;
#13824=ORIENTED_EDGE ( 'NONE', *, *, #4157, .T. ) ;
#13825=ORIENTED_EDGE ( 'NONE', *, *, #2533, .F. ) ;
#13827=FACE_OUTER_BOUND ( 'NONE', #3984, .T. ) ;
#13830=CARTESIAN_POINT ( 'NONE',  ( -442.0000000000000000, -104.9999999999999858, -159.0000000000000000 ) ) ;
#13833=CIRCLE ( 'NONE', #22926, 7.999999999999979572 ) ;
#13835=AXIS2_PLACEMENT_3D ( 'NONE', #22817, #6242, #17144 ) ;
#13837=ORIENTED_EDGE ( 'NONE', *, *, #7817, .T. ) ;
#13841=ORIENTED_EDGE ( 'NONE', *, *, #8840, .F. ) ;
#13842=DIRECTION ( 'NONE',  ( -0.000000000000000000, 0.000000000000000000, 1.000000000000000000 ) ) ;
#13847=ORIENTED_EDGE ( 'NONE', *, *, #25788, .F. ) ;
#13848=CARTESIAN_POINT ( 'NONE',  ( -499.9999999999999432, 144.9999999999999716, -162.9999999999999716 ) ) ;
#13849=LINE ( 'NONE', #21676, #31555 ) ;
#13854=VECTOR ( 'NONE', #3285, 1000.000000000000000 ) ;
#13856=AXIS2_PLACEMENT_3D ( 'NONE', #8537, #30252, #5852 ) ;
#13859=CARTESIAN_POINT ( 'NONE',  ( -418.0000000000000000, 137.0000000000000000, -155.0000000000000000 ) ) ;
#13860=ADVANCED_FACE ( 'NONE', ( #15523 ), #31702, .F. ) ;
#13861=CYLINDRICAL_SURFACE ( 'NONE', #11855, 3.999999999999976019 ) ;
#13869=EDGE_CURVE ( 'NONE', #890, #1214, #17, .T. ) ;
#13871=AXIS2_PLACEMENT_3D ( 'NONE', #24303, #13467, #26989 ) ;
#13874=ORIENTED_EDGE ( 'NONE', *, *, #9780, .T. ) ;
#13883=CYLINDRICAL_SURFACE ( 'NONE', #27584, 3.999999999999976019 ) ;
#13884=ORIENTED_EDGE ( 'NONE', *, *, #31693, .T. ) ;
#13886=CIRCLE ( 'NONE', #33773, 3.999999999999976019 ) ;
#13888=VERTEX_POINT ( 'NONE', #9997 ) ;
#13890=CARTESIAN_POINT ( 'NONE',  ( -12.00000000000001066, 144.9999999999999147, 187.0000000000000000 ) ) ;
#13894=FACE_OUTER_BOUND ( 'NONE', #20257, .T. ) ;
#13895=DIRECTION ( 'NONE',  ( -1.000000000000000000, 0.000000000000000000, 0.000000000000000000 ) ) ;
#13896=CIRCLE ( 'NONE', #6486, 4.750000000000004441 ) ;
#13897=VERTEX_POINT ( 'NONE', #15354 ) ;
#13898=LINE ( 'NONE', #21724, #22779 ) ;
#13904=VECTOR ( 'NONE', #4492, 1000.000000000000000 ) ;
#13907=AXIS2_PLACEMENT_3D ( 'NONE', #3772, #22479, #19982 ) ;
#13910=( LENGTH_UNIT ( ) NAMED_UNIT ( * ) SI_UNIT ( .MILLI., .METRE. ) );
#13912=LINE ( 'NONE', #27602, #28102 ) ;
#13914=ORIENTED_EDGE ( 'NONE', *, *, #14840, .T. ) ;
#13919=DIRECTION ( 'NONE',  ( 0.000000000000000000, 0.000000000000000000, 1.000000000000000000 ) ) ;
#13927=DIRECTION ( 'NONE',  ( 1.000000000000000000, 0.000000000000000000, 0.000000000000000000 ) ) ;
#13931=LINE ( 'NONE', #19453, #25072 ) ;
#13932=EDGE_CURVE ( 'NONE', #15331, #15311, #1720, .T. ) ;
#13934=DIRECTION ( 'NONE',  ( 0.000000000000000000, 0.000000000000000000, -1.000000000000000000 ) ) ;
#13935=CARTESIAN_POINT ( 'NONE',  ( -349.0000000000000000, 134.9999999999999716, 109.9999999999999858 ) ) ;
#13937=CIRCLE ( 'NONE', #12804, 2.000000000000001776 ) ;
#13938=AXIS2_PLACEMENT_3D ( 'NONE', #12632, #31822, #12290 ) ;
#13939=DIRECTION ( 'NONE',  ( -0.000000000000000000, -1.000000000000000000, -0.000000000000000000 ) ) ;
#13941=DIRECTION ( 'NONE',  ( 0.000000000000000000, 5.053935297177146739E-49, 1.000000000000000000 ) ) ;
#13942=DIRECTION ( 'NONE',  ( 0.000000000000000000, -1.000000000000000000, 6.123233995736766036E-17 ) ) ;
#13945=EDGE_CURVE ( 'NONE', #2043, #19944, #19259, .T. ) ;
#13950=ORIENTED_EDGE ( 'NONE', *, *, #25340, .T. ) ;
#13958=DIRECTION ( 'NONE',  ( 0.000000000000000000, -1.000000000000000000, -5.145227585319922065E-49 ) ) ;
#13959=VECTOR ( 'NONE', #27525, 1000.000000000000000 ) ;
#13962=CARTESIAN_POINT ( 'NONE',  ( -449.9999999999999432, -105.0000000000000142, 162.9999999999999716 ) ) ;
#13963=ORIENTED_EDGE ( 'NONE', *, *, #20266, .F. ) ;
#13964=VERTEX_POINT ( 'NONE', #3212 ) ;
#13965=EDGE_CURVE ( 'NONE', #19763, #5382, #29746, .T. ) ;
#13966=VECTOR ( 'NONE', #9730, 1000.000000000000000 ) ;
#13972=EDGE_LOOP ( 'NONE', ( #33305, #21280, #32342, #31166 ) ) ;
#13974=CARTESIAN_POINT ( 'NONE',  ( -365.0000000000000000, 130.9999999999999716, 126.0000000000000000 ) ) ;
#13978=CARTESIAN_POINT ( 'NONE',  ( -414.0000000000000568, -105.0000000000000142, 187.0000000000000000 ) ) ;
#13980=ORIENTED_EDGE ( 'NONE', *, *, #7050, .T. ) ;
#13981=DIRECTION ( 'NONE',  ( 0.000000000000000000, 0.000000000000000000, -1.000000000000000000 ) ) ;
#13984=LINE ( 'NONE', #13454, #31091 ) ;
#13992=ORIENTED_EDGE ( 'NONE', *, *, #11112, .F. ) ;
#13994=DIRECTION ( 'NONE',  ( 0.000000000000000000, 1.131431318426415506E-52, 1.000000000000000000 ) ) ;
#13997=ORIENTED_EDGE ( 'NONE', *, *, #6734, .F. ) ;
#13999=DIRECTION ( 'NONE',  ( -1.000000000000000000, 0.000000000000000000, 0.000000000000000000 ) ) ;
#14000=VECTOR ( 'NONE', #16113, 1000.000000000000000 ) ;
#14004=ORIENTED_EDGE ( 'NONE', *, *, #11781, .T. ) ;
#14008=VECTOR ( 'NONE', #16969, 1000.000000000000000 ) ;
#14012=LINE ( 'NONE', #19187, #5510 ) ;
#14014=ORIENTED_EDGE ( 'NONE', *, *, #22595, .F. ) ;
#14017=DIRECTION ( 'NONE',  ( -0.000000000000000000, -1.000000000000000000, -0.000000000000000000 ) ) ;
#14021=DIRECTION ( 'NONE',  ( -0.000000000000000000, -0.000000000000000000, 1.000000000000000000 ) ) ;
#14023=CARTESIAN_POINT ( 'NONE',  ( -500.0000000000000000, -137.0000000000000000, 194.9999999999999716 ) ) ;
#14024=CARTESIAN_POINT ( 'NONE',  ( -12.00000000000001066, -109.0000000000000142, 174.9999999999999432 ) ) ;
#14025=ADVANCED_FACE ( 'NONE', ( #3560 ), #33822, .T. ) ;
#14027=CIRCLE ( 'NONE', #6026, 7.999999999999979572 ) ;
#14031=LINE ( 'NONE', #24867, #2558 ) ;
#14032=DIRECTION ( 'NONE',  ( 1.000000000000000000, 0.000000000000000000, 0.000000000000000000 ) ) ;
#14033=EDGE_CURVE ( 'NONE', #27516, #4507, #25451, .T. ) ;
#14034=VERTEX_POINT ( 'NONE', #12472 ) ;
#14037=VERTEX_POINT ( 'NONE', #3742 ) ;
#14038=AXIS2_PLACEMENT_3D ( 'NONE', #13417, #5549, #24250 ) ;
#14041=DIRECTION ( 'NONE',  ( 1.000000000000000000, 0.000000000000000000, 0.000000000000000000 ) ) ;
#14045=VERTEX_POINT ( 'NONE', #20128 ) ;
#14048=AXIS2_PLACEMENT_3D ( 'NONE', #24982, #32468, #24449 ) ;
#14050=CIRCLE ( 'NONE', #27098, 4.750000000000004441 ) ;
#14051=VECTOR ( 'NONE', #519, 1000.000000000000000 ) ;
#14052=CARTESIAN_POINT ( 'NONE',  ( -449.9999999999999432, -137.0000000000000000, -155.0000000000000000 ) ) ;
#14054=ORIENTED_EDGE ( 'NONE', *, *, #8263, .F. ) ;
#14055=CARTESIAN_POINT ( 'NONE',  ( -418.0000000000000000, -112.9999999999999858, -155.0000000000000000 ) ) ;
#14058=DIRECTION ( 'NONE',  ( 0.000000000000000000, 0.000000000000000000, 1.000000000000000000 ) ) ;
#14060=ORIENTED_EDGE ( 'NONE', *, *, #8464, .F. ) ;
#14071=AXIS2_PLACEMENT_3D ( 'NONE', #10966, #21813, #11324 ) ;
#14073=PLANE ( 'NONE',  #1981 ) ;
#14074=DIRECTION ( 'NONE',  ( -1.000000000000000000, 0.000000000000000000, 0.000000000000000000 ) ) ;
#14075=EDGE_CURVE ( 'NONE', #26932, #32711, #31159, .T. ) ;
#14076=VECTOR ( 'NONE', #20365, 1000.000000000000000 ) ;
#14078=VERTEX_POINT ( 'NONE', #9618 ) ;
#14079=ADVANCED_FACE ( 'NONE', ( #30801 ), #8909, .T. ) ;
#14081=EDGE_LOOP ( 'NONE', ( #21722, #12266, #6978, #5058 ) ) ;
#14082=VERTEX_POINT ( 'NONE', #19781 ) ;
#14086=CARTESIAN_POINT ( 'NONE',  ( -70.00000000000000000, 4.559999999999909015, -168.2400000000000091 ) ) ;
#14087=CARTESIAN_POINT ( 'NONE',  ( 19.99999999999998224, 134.9999999999998863, 162.9999999999999716 ) ) ;
#14089=EDGE_LOOP ( 'NONE', ( #29037, #13950, #1424, #6901, #3520, #22634, #627, #34893, #17127, #5067, #9999, #73, #30364, #22297, #15248, #15888 ) ) ;
#14093=LINE ( 'NONE', #6406, #8195 ) ;
#14095=AXIS2_PLACEMENT_3D ( 'NONE', #23021, #3785, #1475 ) ;
#14101=DIRECTION ( 'NONE',  ( 1.000000000000000000, 0.000000000000000000, 0.000000000000000000 ) ) ;
#14104=DIRECTION ( 'NONE',  ( 0.000000000000000000, 0.000000000000000000, -1.000000000000000000 ) ) ;
#14106=PLANE ( 'NONE',  #28783 ) ;
#14109=LINE ( 'NONE', #19108, #30539 ) ;
#14110=CYLINDRICAL_SURFACE ( 'NONE', #17159, 4.000000000000003553 ) ;
#14113=DIRECTION ( 'NONE',  ( 0.000000000000000000, -0.000000000000000000, -1.000000000000000000 ) ) ;
#14115=CARTESIAN_POINT ( 'NONE',  ( -12.00000000000001066, -124.9999999999999432, -158.9999999999999716 ) ) ;
#14117=DIRECTION ( 'NONE',  ( 1.000000000000000000, 0.000000000000000000, 0.000000000000000000 ) ) ;
#14121=ORIENTED_EDGE ( 'NONE', *, *, #9161, .T. ) ;
#14127=ORIENTED_EDGE ( 'NONE', *, *, #12636, .T. ) ;
#14129=EDGE_LOOP ( 'NONE', ( #9475, #18130, #20241, #10515, #16118, #33243, #10421, #13115 ) ) ;
#14130=ORIENTED_EDGE ( 'NONE', *, *, #576, .T. ) ;
#14131=CARTESIAN_POINT ( 'NONE',  ( -19.99999999999998934, 144.9999999999999147, 187.0000000000000000 ) ) ;
#14136=DIRECTION ( 'NONE',  ( 0.000000000000000000, 0.000000000000000000, -1.000000000000000000 ) ) ;
#14137=DIRECTION ( 'NONE',  ( 0.000000000000000000, 1.000000000000000000, 0.000000000000000000 ) ) ;
#14138=ORIENTED_EDGE ( 'NONE', *, *, #1938, .T. ) ;
#14139=EDGE_LOOP ( 'NONE', ( #25207, #20221, #6511, #12589 ) ) ;
#14140=DIRECTION ( 'NONE',  ( -1.848892746611746419E-32, -6.842277657836020854E-49, 1.000000000000000000 ) ) ;
#14142=EDGE_CURVE ( 'NONE', #19207, #1031, #28131, .T. ) ;
#14144=CIRCLE ( 'NONE', #20396, 4.000000000000003553 ) ;
#14146=FACE_OUTER_BOUND ( 'NONE', #30566, .T. ) ;
#14147=ORIENTED_EDGE ( 'NONE', *, *, #1199, .F. ) ;
#14149=DIRECTION ( 'NONE',  ( -0.000000000000000000, -1.000000000000000000, -0.000000000000000000 ) ) ;
#14151=ADVANCED_FACE ( 'NONE', ( #10307, #34884, #18172 ), #26148, .F. ) ;
#14152=CARTESIAN_POINT ( 'NONE',  ( -70.00000000000000000, 75.55999999999990280, 177.7400000000000091 ) ) ;
#14155=CARTESIAN_POINT ( 'NONE',  ( 0.000000000000000000, -55.00000000000000711, 155.0000000000000000 ) ) ;
#14156=DIRECTION ( 'NONE',  ( 1.232595164407830946E-32, 3.421138828918010427E-49, -1.000000000000000000 ) ) ;
#14166=EDGE_LOOP ( 'NONE', ( #10385, #13722, #28171, #16844 ) ) ;
#14167=EDGE_CURVE ( 'NONE', #28571, #18201, #12996, .T. ) ;
#14168=ADVANCED_FACE ( 'NONE', ( #7098 ), #13167, .T. ) ;
#14170=DIRECTION ( 'NONE',  ( -0.000000000000000000, 1.000000000000000000, -0.000000000000000000 ) ) ;
#14173=ORIENTED_EDGE ( 'NONE', *, *, #21552, .F. ) ;
#14175=EDGE_LOOP ( 'NONE', ( #23403, #13635, #4138, #6759 ) ) ;
#14178=EDGE_LOOP ( 'NONE', ( #3944, #14462, #5765, #15182 ) ) ;
#14181=LINE ( 'NONE', #8644, #6762 ) ;
#14184=CARTESIAN_POINT ( 'NONE',  ( -20.00000000000007461, 108.9999999999999858, 187.0000000000000000 ) ) ;
#14186=ORIENTED_EDGE ( 'NONE', *, *, #4130, .T. ) ;
#14187=LINE ( 'NONE', #9182, #16245 ) ;
#14191=LINE ( 'NONE', #35026, #6916 ) ;
#14196=CARTESIAN_POINT ( 'NONE',  ( -19.99999999999998934, 75.55999999999990280, -172.9900000000000091 ) ) ;
#14197=CARTESIAN_POINT ( 'NONE',  ( -12.00000000000001066, 124.9999999999999716, 155.0000000000000000 ) ) ;
#14198=ORIENTED_EDGE ( 'NONE', *, *, #6848, .T. ) ;
#14208=CARTESIAN_POINT ( 'NONE',  ( -499.9999999999999432, 108.9999999999999858, -162.9999999999999716 ) ) ;
#14211=DIRECTION ( 'NONE',  ( -0.000000000000000000, -1.000000000000000000, -0.000000000000000000 ) ) ;
#14212=LINE ( 'NONE', #3507, #7691 ) ;
#14213=DIRECTION ( 'NONE',  ( 0.000000000000000000, -5.145227585319922065E-49, -1.000000000000000000 ) ) ;
#14217=CARTESIAN_POINT ( 'NONE',  ( -449.9999999999999432, -104.9999999999999858, -187.0000000000000000 ) ) ;
#14218=EDGE_CURVE ( 'NONE', #9057, #34809, #8686, .T. ) ;
#14222=CARTESIAN_POINT ( 'NONE',  ( -410.0000000000000568, 105.0000000000000000, -77.99999999999997158 ) ) ;
#14225=VERTEX_POINT ( 'NONE', #16546 ) ;
#14230=( LENGTH_UNIT ( ) NAMED_UNIT ( * ) SI_UNIT ( .MILLI., .METRE. ) );
#14233=ADVANCED_FACE ( 'NONE', ( #2990 ), #12085, .T. ) ;
#14241=DIRECTION ( 'NONE',  ( 1.000000000000000000, 0.000000000000000000, -1.232595164407831220E-32 ) ) ;
#14243=ORIENTED_EDGE ( 'NONE', *, *, #32694, .T. ) ;
#14246=CARTESIAN_POINT ( 'NONE',  ( 15.99999999999998579, 75.55999999999990280, 172.9900000000000091 ) ) ;
#14251=CARTESIAN_POINT ( 'NONE',  ( -499.9999999999999432, 112.9999999999999574, -155.0000000000000000 ) ) ;
#14252=CARTESIAN_POINT ( 'NONE',  ( -499.9999999999999432, 140.9999999999999716, 162.9999999999999716 ) ) ;
#14254=CARTESIAN_POINT ( 'NONE',  ( -12.00000000000001066, -124.9999999999999432, -154.9999999999999716 ) ) ;
#14255=VERTEX_POINT ( 'NONE', #30756 ) ;
#14259=ORIENTED_EDGE ( 'NONE', *, *, #7247, .F. ) ;
#14266=VERTEX_POINT ( 'NONE', #23113 ) ;
#14267=LINE ( 'NONE', #24752, #9952 ) ;
#14273=FACE_OUTER_BOUND ( 'NONE', #9522, .T. ) ;
#14274=AXIS2_PLACEMENT_3D ( 'NONE', #6458, #33522, #33881 ) ;
#14278=VECTOR ( 'NONE', #2235, 1000.000000000000000 ) ;
#14280=DIRECTION ( 'NONE',  ( 0.000000000000000000, 0.000000000000000000, 1.000000000000000000 ) ) ;
#14284=PLANE ( 'NONE',  #29999 ) ;
#14285=CARTESIAN_POINT ( 'NONE',  ( 11.99999999999999645, 134.9999999999999432, -194.9999999999999432 ) ) ;
#14286=FACE_OUTER_BOUND ( 'NONE', #7732, .T. ) ;
#14289=VECTOR ( 'NONE', #24272, 1000.000000000000000 ) ;
#14292=EDGE_CURVE ( 'NONE', #19981, #6277, #20091, .T. ) ;
#14294=FACE_OUTER_BOUND ( 'NONE', #33235, .T. ) ;
#14295=LINE ( 'NONE', #33666, #9990 ) ;
#14296=UNCERTAINTY_MEASURE_WITH_UNIT (LENGTH_MEASURE( 1.000000000000000082E-05 ), #32654, 'distance_accuracy_value', 'NONE');
#14297=CARTESIAN_POINT ( 'NONE',  ( -418.0000000000000000, -124.9999999999999858, -69.99999999999998579 ) ) ;
#14298=ORIENTED_EDGE ( 'NONE', *, *, #33045, .F. ) ;
#14299=LINE ( 'NONE', #9296, #16770 ) ;
#14301=ORIENTED_EDGE ( 'NONE', *, *, #26914, .F. ) ;
#14305=VECTOR ( 'NONE', #1675, 1000.000000000000000 ) ;
#14306=VECTOR ( 'NONE', #26002, 1000.000000000000000 ) ;
#14314=CIRCLE ( 'NONE', #17166, 7.999999999999979572 ) ;
#14316=ORIENTED_EDGE ( 'NONE', *, *, #34113, .T. ) ;
#14320=ORIENTED_EDGE ( 'NONE', *, *, #20259, .F. ) ;
#14321=LINE ( 'NONE', #30142, #23649 ) ;
#14323=ADVANCED_FACE ( 'NONE', ( #31283 ), #27904, .T. ) ;
#14327=LINE ( 'NONE', #27655, #27345 ) ;
#14329=VECTOR ( 'NONE', #14825, 1000.000000000000000 ) ;
#14331=VECTOR ( 'NONE', #17054, 1000.000000000000000 ) ;
#14332=EDGE_CURVE ( 'NONE', #7246, #11377, #28455, .T. ) ;
#14333=EDGE_CURVE ( 'NONE', #15331, #6935, #3866, .T. ) ;
#14335=ORIENTED_EDGE ( 'NONE', *, *, #2326, .F. ) ;
#14336=AXIS2_PLACEMENT_3D ( 'NONE', #19030, #24686, #27020 ) ;
#14338=AXIS2_PLACEMENT_3D ( 'NONE', #22426, #27934, #30962 ) ;
#14342=( NAMED_UNIT ( * ) SI_UNIT ( $, .STERADIAN. ) SOLID_ANGLE_UNIT ( ) );
#14344=ORIENTED_EDGE ( 'NONE', *, *, #13945, .F. ) ;
#14355=CIRCLE ( 'NONE', #30231, 3.999999999999976019 ) ;
#14358=EDGE_LOOP ( 'NONE', ( #17648, #28040, #11682, #3368, #30721, #28579, #24619, #944 ) ) ;
#14360=EDGE_LOOP ( 'NONE', ( #8618, #8519, #16762, #10067 ) ) ;
#14361=VERTEX_POINT ( 'NONE', #14929 ) ;
#14365=CARTESIAN_POINT ( 'NONE',  ( -361.0000000000000000, -125.0000000000000284, 185.0000000000000000 ) ) ;
#14367=ORIENTED_EDGE ( 'NONE', *, *, #14858, .F. ) ;
#14371=LINE ( 'NONE', #2475, #19284 ) ;
#14377=VERTEX_POINT ( 'NONE', #29132 ) ;
#14380=AXIS2_PLACEMENT_3D ( 'NONE', #34602, #31909, #9396 ) ;
#14381=CARTESIAN_POINT ( 'NONE',  ( -445.9999999999999432, 105.0000000000000000, 132.0000000000000000 ) ) ;
#14384=CIRCLE ( 'NONE', #5803, 3.999999999999976019 ) ;
#14386=PLANE ( 'NONE',  #29731 ) ;
#14389=DIRECTION ( 'NONE',  ( 0.000000000000000000, -6.123233995736766036E-17, -1.000000000000000000 ) ) ;
#14391=EDGE_CURVE ( 'NONE', #27733, #30526, #7233, .T. ) ;
#14392=ORIENTED_EDGE ( 'NONE', *, *, #25648, .F. ) ;
#14397=ORIENTED_EDGE ( 'NONE', *, *, #21753, .T. ) ;
#14402=EDGE_LOOP ( 'NONE', ( #9232, #19740, #32688, #20649, #17512, #9647, #5293, #31679 ) ) ;
#14404=EDGE_CURVE ( 'NONE', #19234, #17537, #26640, .T. ) ;
#14406=DIRECTION ( 'NONE',  ( 0.000000000000000000, 0.000000000000000000, -1.000000000000000000 ) ) ;
#14412=CIRCLE ( 'NONE', #14963, 4.000000000000003553 ) ;
#14413=ORIENTED_EDGE ( 'NONE', *, *, #33568, .F. ) ;
#14421=CARTESIAN_POINT ( 'NONE',  ( -361.0000000000000000, -135.0000000000000000, 126.0000000000000000 ) ) ;
#14423=ORIENTED_EDGE ( 'NONE', *, *, #23237, .T. ) ;
#14429=CARTESIAN_POINT ( 'NONE',  ( -500.0000000000000000, 144.9999999999999716, -155.0000000000000000 ) ) ;
#14430=LINE ( 'NONE', #1069, #9305 ) ;
#14433=CIRCLE ( 'NONE', #31453, 7.999999999999979572 ) ;
#14436=FACE_OUTER_BOUND ( 'NONE', #7182, .T. ) ;
#14438=ORIENTED_EDGE ( 'NONE', *, *, #2668, .T. ) ;
#14439=ADVANCED_FACE ( 'NONE', ( #9921 ), #2253, .T. ) ;
#14440=ADVANCED_FACE ( 'NONE', ( #23627 ), #4215, .T. ) ;
#14446=DIRECTION ( 'NONE',  ( -3.469446951953832974E-18, -1.000000000000000000, -7.888609052210116302E-31 ) ) ;
#14447=VECTOR ( 'NONE', #5476, 1000.000000000000000 ) ;
#14452=CARTESIAN_POINT ( 'NONE',  ( 11.99999999999995559, -134.9999999999999716, -162.9999999999999432 ) ) ;
#14454=AXIS2_PLACEMENT_3D ( 'NONE', #14821, #9473, #11809 ) ;
#14456=ORIENTED_EDGE ( 'NONE', *, *, #11954, .T. ) ;
#14460=DIRECTION ( 'NONE',  ( -0.000000000000000000, 2.465190328815661892E-32, 1.000000000000000000 ) ) ;
#14461=DIRECTION ( 'NONE',  ( 0.000000000000000000, 1.000000000000000000, 5.145227585319922065E-49 ) ) ;
#14462=ORIENTED_EDGE ( 'NONE', *, *, #33877, .T. ) ;
#14467=DIRECTION ( 'NONE',  ( -3.040835319149746528E-31, -1.000000000000000000, 0.000000000000000000 ) ) ;
#14470=DIRECTION ( 'NONE',  ( -0.000000000000000000, -0.000000000000000000, 1.000000000000000000 ) ) ;
#14474=ORIENTED_EDGE ( 'NONE', *, *, #30089, .T. ) ;
#14479=ORIENTED_EDGE ( 'NONE', *, *, #12404, .T. ) ;
#14480=EDGE_CURVE ( 'NONE', #14078, #5880, #21306, .T. ) ;
#14483=AXIS2_PLACEMENT_3D ( 'NONE', #31857, #23178, #1975 ) ;
#14484=EDGE_CURVE ( 'NONE', #10828, #8663, #12437, .T. ) ;
#14490=ORIENTED_EDGE ( 'NONE', *, *, #15158, .F. ) ;
#14491=CARTESIAN_POINT ( 'NONE',  ( -499.9999999999999432, -113.0000000000000000, -187.0000000000000000 ) ) ;
#14494=ORIENTED_EDGE ( 'NONE', *, *, #6508, .F. ) ;
#14497=ORIENTED_EDGE ( 'NONE', *, *, #16050, .T. ) ;
#14502=DIRECTION ( 'NONE',  ( -1.000000000000000000, 0.000000000000000000, 0.000000000000000000 ) ) ;
#14503=CARTESIAN_POINT ( 'NONE',  ( -355.0000000000000000, -119.0000000000000000, 113.9999999999999858 ) ) ;
#14507=VECTOR ( 'NONE', #497, 1000.000000000000000 ) ;
#14508=VECTOR ( 'NONE', #17806, 1000.000000000000000 ) ;
#14510=ORIENTED_EDGE ( 'NONE', *, *, #26034, .F. ) ;
#14513=DIRECTION ( 'NONE',  ( 0.000000000000000000, 0.000000000000000000, -1.000000000000000000 ) ) ;
#14515=DIRECTION ( 'NONE',  ( 1.000000000000000000, 3.469446951953834515E-18, 0.000000000000000000 ) ) ;
#14519=CARTESIAN_POINT ( 'NONE',  ( -449.9999999999999432, -105.0000000000000142, 162.9999999999999716 ) ) ;
#14521=DIRECTION ( 'NONE',  ( 1.000000000000000000, -0.000000000000000000, -0.000000000000000000 ) ) ;
#14523=CIRCLE ( 'NONE', #34961, 7.999999999999952038 ) ;
#14524=ORIENTED_EDGE ( 'NONE', *, *, #32480, .T. ) ;
#14526=DIRECTION ( 'NONE',  ( -0.000000000000000000, 1.000000000000000000, -0.000000000000000000 ) ) ;
#14529=ORIENTED_EDGE ( 'NONE', *, *, #23966, .F. ) ;
#14530=ORIENTED_EDGE ( 'NONE', *, *, #7983, .F. ) ;
#14532=EDGE_CURVE ( 'NONE', #17865, #30730, #33579, .T. ) ;
#14534=ORIENTED_EDGE ( 'NONE', *, *, #6812, .T. ) ;
#14535=DIRECTION ( 'NONE',  ( 0.000000000000000000, 1.000000000000000000, 1.224646799147353207E-16 ) ) ;
#14540=ADVANCED_FACE ( 'NONE', ( #20781 ), #20954, .F. ) ;
#14542=DIRECTION ( 'NONE',  ( 0.000000000000000000, 0.000000000000000000, 1.000000000000000000 ) ) ;
#14547=LINE ( 'NONE', #17923, #31145 ) ;
#14548=DIRECTION ( 'NONE',  ( 0.000000000000000000, 2.309213040847544338E-50, 1.000000000000000000 ) ) ;
#14549=CARTESIAN_POINT ( 'NONE',  ( -361.0000000000000000, -125.0000000000000284, 183.0000000000000000 ) ) ;
#14550=DIRECTION ( 'NONE',  ( 0.000000000000000000, -1.000000000000000000, 3.374343856708137958E-53 ) ) ;
#14554=EDGE_LOOP ( 'NONE', ( #33413, #18696, #7348, #19012 ) ) ;
#14556=CARTESIAN_POINT ( 'NONE',  ( -418.0000000000000000, -137.0000000000000000, -175.0000000000000000 ) ) ;
#14557=DIRECTION ( 'NONE',  ( 0.000000000000000000, 1.000000000000000000, 1.224646799147353207E-16 ) ) ;
#14559=ORIENTED_EDGE ( 'NONE', *, *, #9714, .F. ) ;
#14560=FACE_OUTER_BOUND ( 'NONE', #1285, .T. ) ;
#14568=CARTESIAN_POINT ( 'NONE',  ( -418.0000000000000000, -141.0000000000000000, 154.9999999999999716 ) ) ;
#14569=FACE_OUTER_BOUND ( 'NONE', #7449, .T. ) ;
#14570=ADVANCED_FACE ( 'NONE', ( #27332 ), #26995, .F. ) ;
#14572=VECTOR ( 'NONE', #20567, 1000.000000000000000 ) ;
#14576=FACE_OUTER_BOUND ( 'NONE', #15124, .T. ) ;
#14577=VERTEX_POINT ( 'NONE', #473 ) ;
#14578=VECTOR ( 'NONE', #29945, 1000.000000000000000 ) ;
#14579=FACE_OUTER_BOUND ( 'NONE', #14402, .T. ) ;
#14580=DIRECTION ( 'NONE',  ( -0.000000000000000000, -0.000000000000000000, -1.000000000000000000 ) ) ;
#14582=CARTESIAN_POINT ( 'NONE',  ( -349.0000000000000000, -125.0000000000000284, 128.0000000000000000 ) ) ;
#14586=VERTEX_POINT ( 'NONE', #27515 ) ;
#14587=LINE ( 'NONE', #28273, #14051 ) ;
#14589=EDGE_CURVE ( 'NONE', #10753, #31620, #23343, .T. ) ;
#14591=VECTOR ( 'NONE', #17570, 1000.000000000000000 ) ;
#14592=DIRECTION ( 'NONE',  ( -1.000000000000000000, -3.040835319149746528E-31, -1.232595164407830946E-32 ) ) ;
#14594=VERTEX_POINT ( 'NONE', #8117 ) ;
#14596=DIRECTION ( 'NONE',  ( 0.000000000000000000, 0.000000000000000000, -1.000000000000000000 ) ) ;
#14597=EDGE_LOOP ( 'NONE', ( #13727, #13800, #17251, #4219 ) ) ;
#14605=VECTOR ( 'NONE', #27962, 1000.000000000000000 ) ;
#14606=LINE ( 'NONE', #8532, #23147 ) ;
#14608=DIRECTION ( 'NONE',  ( 0.000000000000000000, 1.000000000000000000, 0.000000000000000000 ) ) ;
#14613=CARTESIAN_POINT ( 'NONE',  ( 15.99999999999998579, -124.9999999999999432, -186.9999999999999716 ) ) ;
#14614=DIRECTION ( 'NONE',  ( 0.000000000000000000, -2.309213040847544338E-50, -1.000000000000000000 ) ) ;
#14615=CARTESIAN_POINT ( 'NONE',  ( 15.99999999999998579, 112.9999999999999574, 155.0000000000000000 ) ) ;
#14616=( NAMED_UNIT ( * ) SI_UNIT ( $, .STERADIAN. ) SOLID_ANGLE_UNIT ( ) );
#14623=ORIENTED_EDGE ( 'NONE', *, *, #12742, .T. ) ;
#14626=LINE ( 'NONE', #14086, #11281 ) ;
#14628=CARTESIAN_POINT ( 'NONE',  ( 19.99999999999998934, 124.9999999999999716, 162.9999999999999716 ) ) ;
#14635=VERTEX_POINT ( 'NONE', #11161 ) ;
#14638=LINE ( 'NONE', #17132, #34588 ) ;
#14641=ORIENTED_EDGE ( 'NONE', *, *, #5856, .T. ) ;
#14643=DIRECTION ( 'NONE',  ( 0.000000000000000000, 0.000000000000000000, -1.000000000000000000 ) ) ;
#14648=CIRCLE ( 'NONE', #5509, 4.750000000000004441 ) ;
#14651=DIRECTION ( 'NONE',  ( -1.300283923313630633E-47, 0.000000000000000000, -1.000000000000000000 ) ) ;
#14662=ORIENTED_EDGE ( 'NONE', *, *, #7050, .F. ) ;
#14667=CARTESIAN_POINT ( 'NONE',  ( -20.00000000000007461, 136.9999999999999432, 187.0000000000000000 ) ) ;
#14668=ORIENTED_EDGE ( 'NONE', *, *, #21846, .T. ) ;
#14673=AXIS2_PLACEMENT_3D ( 'NONE', #21930, #8567, #30285 ) ;
#14682=EDGE_CURVE ( 'NONE', #18383, #24429, #20502, .T. ) ;
#14687=ADVANCED_FACE ( 'NONE', ( #24135 ), #22359, .T. ) ;
#14688=FACE_OUTER_BOUND ( 'NONE', #34977, .T. ) ;
#14692=CARTESIAN_POINT ( 'NONE',  ( -15.99999999999998579, 144.9999999999999716, -162.9999999999999147 ) ) ;
#14696=CARTESIAN_POINT ( 'NONE',  ( 11.99999999999999645, 144.9999999999999716, -194.9999999999999432 ) ) ;
#14699=DIRECTION ( 'NONE',  ( 1.000000000000000000, 0.000000000000000000, -1.848892746611746966E-32 ) ) ;
#14703=LINE ( 'NONE', #30873, #15421 ) ;
#14704=LINE ( 'NONE', #17719, #3201 ) ;
#14716=CARTESIAN_POINT ( 'NONE',  ( -12.00000000000001066, 144.9999999999999716, 162.9999999999999716 ) ) ;
#14719=CARTESIAN_POINT ( 'NONE',  ( -11.99999999999998224, -145.0000000000000000, 162.9999999999999716 ) ) ;
#14720=CARTESIAN_POINT ( 'NONE',  ( 11.99999999999999645, -124.9999999999999432, -162.9999999999999432 ) ) ;
#14722=ORIENTED_EDGE ( 'NONE', *, *, #22508, .T. ) ;
#14727=EDGE_CURVE ( 'NONE', #1001, #14361, #19700, .T. ) ;
#14729=CARTESIAN_POINT ( 'NONE',  ( -363.0000000000000000, -125.0000000000000284, 168.9999999999999716 ) ) ;
#14731=ADVANCED_FACE ( 'NONE', ( #30895 ), #28228, .F. ) ;
#14732=DIRECTION ( 'NONE',  ( 1.000000000000000000, -0.000000000000000000, -0.000000000000000000 ) ) ;
#14733=ORIENTED_EDGE ( 'NONE', *, *, #5837, .T. ) ;
#14734=ADVANCED_FACE ( 'NONE', ( #3825 ), #1171, .T. ) ;
#14736=CARTESIAN_POINT ( 'NONE',  ( -418.0000000000000000, -105.0000000000000142, -69.99999999999998579 ) ) ;
#14738=CARTESIAN_POINT ( 'NONE',  ( -499.9999999999999432, 112.9999999999999574, 190.9999999999999716 ) ) ;
#14740=DIRECTION ( 'NONE',  ( 0.000000000000000000, 1.000000000000000000, 5.053935297177146739E-49 ) ) ;
#14741=ORIENTED_EDGE ( 'NONE', *, *, #17734, .T. ) ;
#14745=ORIENTED_EDGE ( 'NONE', *, *, #28297, .F. ) ;
#14750=CIRCLE ( 'NONE', #9065, 8.000000000000007105 ) ;
#14756=CARTESIAN_POINT ( 'NONE',  ( -12.00000000000001066, -145.0000000000000000, 190.9999999999999716 ) ) ;
#14757=DIRECTION ( 'NONE',  ( -3.040835319149746090E-31, -1.000000000000000000, 0.000000000000000000 ) ) ;
#14758=CARTESIAN_POINT ( 'NONE',  ( -418.0000000000000000, -125.0000000000000000, 100.0000000000000000 ) ) ;
#14760=VERTEX_POINT ( 'NONE', #14184 ) ;
#14764=DIRECTION ( 'NONE',  ( 0.000000000000000000, 1.310824597558155437E-49, 1.000000000000000000 ) ) ;
#14765=AXIS2_PLACEMENT_3D ( 'NONE', #9135, #20010, #30855 ) ;
#14766=CARTESIAN_POINT ( 'NONE',  ( 19.99999999999990763, -134.9999999999999716, -186.9999999999999716 ) ) ;
#14767=ORIENTED_EDGE ( 'NONE', *, *, #7701, .F. ) ;
#14768=CYLINDRICAL_SURFACE ( 'NONE', #21418, 7.999999999999979572 ) ;
#14769=CARTESIAN_POINT ( 'NONE',  ( -442.0000000000000000, 113.0000000000000000, -155.0000000000000000 ) ) ;
#14770=ORIENTED_EDGE ( 'NONE', *, *, #5835, .T. ) ;
#14775=ORIENTED_EDGE ( 'NONE', *, *, #6964, .F. ) ;
#14780=VERTEX_POINT ( 'NONE', #14365 ) ;
#14783=PLANE ( 'NONE',  #210 ) ;
#14785=LINE ( 'NONE', #1240, #32463 ) ;
#14789=ADVANCED_FACE ( 'NONE', ( #11506 ), #11872, .F. ) ;
#14790=VECTOR ( 'NONE', #33836, 1000.000000000000000 ) ;
#14791=ORIENTED_EDGE ( 'NONE', *, *, #21057, .F. ) ;
#14797=DIRECTION ( 'NONE',  ( 0.000000000000000000, 2.309213040847544338E-50, 1.000000000000000000 ) ) ;
#14801=CARTESIAN_POINT ( 'NONE',  ( -12.00000000000001066, 124.9999999999999716, 155.0000000000000000 ) ) ;
#14802=DIRECTION ( 'NONE',  ( 0.000000000000000000, 1.131431318426415506E-52, 1.000000000000000000 ) ) ;
#14803=ORIENTED_EDGE ( 'NONE', *, *, #28290, .F. ) ;
#14805=DIRECTION ( 'NONE',  ( 0.000000000000000000, 0.000000000000000000, 1.000000000000000000 ) ) ;
#14806=DIRECTION ( 'NONE',  ( 0.000000000000000000, 1.131431318426415506E-52, 1.000000000000000000 ) ) ;
#14808=ORIENTED_EDGE ( 'NONE', *, *, #28887, .F. ) ;
#14809=LINE ( 'NONE', #22462, #18568 ) ;
#14810=DIRECTION ( 'NONE',  ( -1.300283923313630633E-47, 0.000000000000000000, -1.000000000000000000 ) ) ;
#14811=EDGE_CURVE ( 'NONE', #16642, #11839, #1000, .T. ) ;
#14812=DIRECTION ( 'NONE',  ( 1.000000000000000000, 0.000000000000000000, 0.000000000000000000 ) ) ;
#14814=EDGE_LOOP ( 'NONE', ( #11326, #21262, #27490, #32789 ) ) ;
#14821=CARTESIAN_POINT ( 'NONE',  ( -418.0000000000000000, -141.0000000000000000, -175.0000000000000000 ) ) ;
#14823=ORIENTED_EDGE ( 'NONE', *, *, #20624, .F. ) ;
#14824=CARTESIAN_POINT ( 'NONE',  ( 19.99999999999998934, -32.99999999999997158, 155.0000000000000000 ) ) ;
#14825=DIRECTION ( 'NONE',  ( 0.000000000000000000, 1.000000000000000000, 0.000000000000000000 ) ) ;
#14827=ORIENTED_EDGE ( 'NONE', *, *, #27651, .F. ) ;
#14828=ORIENTED_EDGE ( 'NONE', *, *, #34559, .F. ) ;
#14829=EDGE_CURVE ( 'NONE', #15936, #11473, #31753, .T. ) ;
#14832=ADVANCED_FACE ( 'NONE', ( #7191 ), #28745, .F. ) ;
#14835=VECTOR ( 'NONE', #6785, 1000.000000000000000 ) ;
#14836=VERTEX_POINT ( 'NONE', #10054 ) ;
#14839=CARTESIAN_POINT ( 'NONE',  ( -361.0000000000000000, -125.0000000000000284, 113.9999999999999858 ) ) ;
#14840=EDGE_CURVE ( 'NONE', #8592, #8166, #14855, .T. ) ;
#14844=LINE ( 'NONE', #15014, #24870 ) ;
#14845=DIRECTION ( 'NONE',  ( -1.000000000000000000, 0.000000000000000000, 0.000000000000000000 ) ) ;
#14846=ORIENTED_EDGE ( 'NONE', *, *, #21804, .F. ) ;
#14849=AXIS2_PLACEMENT_3D ( 'NONE', #31087, #25732, #1358 ) ;
#14851=CARTESIAN_POINT ( 'NONE',  ( -500.0000000000000000, 144.9999999999999716, 155.0000000000000000 ) ) ;
#14852=CARTESIAN_POINT ( 'NONE',  ( -410.0000000000000568, -137.0000000000000000, -175.0000000000000000 ) ) ;
#14854=VERTEX_POINT ( 'NONE', #20741 ) ;
#14855=CIRCLE ( 'NONE', #4018, 3.999999999999982681 ) ;
#14856=FACE_OUTER_BOUND ( 'NONE', #8103, .T. ) ;
#14858=EDGE_CURVE ( 'NONE', #6669, #6498, #16554, .T. ) ;
#14868=LINE ( 'NONE', #25701, #25199 ) ;
#14869=VECTOR ( 'NONE', #18524, 1000.000000000000000 ) ;
#14873=CARTESIAN_POINT ( 'NONE',  ( -12.00000000000001066, -56.99999999999997868, -154.9999999999999716 ) ) ;
#14875=CARTESIAN_POINT ( 'NONE',  ( -12.00000000000001066, 134.9999999999999432, -162.9999999999999432 ) ) ;
#14877=ORIENTED_EDGE ( 'NONE', *, *, #27509, .F. ) ;
#14879=EDGE_CURVE ( 'NONE', #16498, #842, #7537, .T. ) ;
#14880=ADVANCED_FACE ( 'NONE', ( #26241 ), #34259, .F. ) ;
#14881=VERTEX_POINT ( 'NONE', #9539 ) ;
#14883=VERTEX_POINT ( 'NONE', #20400 ) ;
#14888=CARTESIAN_POINT ( 'NONE',  ( -12.00000000000006573, -145.0000000000000000, -186.9999999999999716 ) ) ;
#14893=VECTOR ( 'NONE', #19903, 1000.000000000000000 ) ;
#14895=LINE ( 'NONE', #12049, #9521 ) ;
#14902=VERTEX_POINT ( 'NONE', #6841 ) ;
#14906=ORIENTED_EDGE ( 'NONE', *, *, #5193, .F. ) ;
#14908=DIRECTION ( 'NONE',  ( 1.000000000000000000, 0.000000000000000000, 0.000000000000000000 ) ) ;
#14909=EDGE_LOOP ( 'NONE', ( #13736, #14530, #29265, #5929, #6794 ) ) ;
#14911=LINE ( 'NONE', #10077, #33590 ) ;
#14913=AXIS2_PLACEMENT_3D ( 'NONE', #5459, #21664, #10988 ) ;
#14914=EDGE_LOOP ( 'NONE', ( #1111, #17602, #9069, #6959 ) ) ;
#14915=AXIS2_PLACEMENT_3D ( 'NONE', #26657, #23815, #7252 ) ;
#14918=AXIS2_PLACEMENT_3D ( 'NONE', #24330, #9358, #4939 ) ;
#14924=ADVANCED_FACE ( 'NONE', ( #15577 ), #15063, .T. ) ;
#14926=CARTESIAN_POINT ( 'NONE',  ( -363.0000000000000000, 124.9999999999999432, 181.0000000000000000 ) ) ;
#14928=LINE ( 'NONE', #34120, #17925 ) ;
#14929=CARTESIAN_POINT ( 'NONE',  ( -430.0000000000000000, 130.9999999999999716, 111.9999999999999858 ) ) ;
#14932=ORIENTED_EDGE ( 'NONE', *, *, #16893, .F. ) ;
#14934=CLOSED_SHELL ( 'NONE', ( #459, #18211, #34663, #24891, #18979, #33868, #14233, #10043, #22463, #16450, #21768, #21738, #33073, #14968, #14731, #6704, #34226, #24929 ) ) ;
#14937=CARTESIAN_POINT ( 'NONE',  ( -349.0000000000000000, 134.9999999999999716, 113.9999999999999858 ) ) ;
#14942=VECTOR ( 'NONE', #26259, 1000.000000000000000 ) ;
#14949=VERTEX_POINT ( 'NONE', #23758 ) ;
#14951=CARTESIAN_POINT ( 'NONE',  ( -442.0000000000000000, -125.0000000000000000, 155.0000000000000000 ) ) ;
#14952=DIRECTION ( 'NONE',  ( 0.000000000000000000, 0.000000000000000000, 1.000000000000000000 ) ) ;
#14954=UNCERTAINTY_MEASURE_WITH_UNIT (LENGTH_MEASURE( 1.000000000000000082E-05 ), #11939, 'distance_accuracy_value', 'NONE');
#14956=DIRECTION ( 'NONE',  ( -0.000000000000000000, 1.000000000000000000, -0.000000000000000000 ) ) ;
#14957=ADVANCED_FACE ( 'NONE', ( #34615 ), #10225, .F. ) ;
#14960=CIRCLE ( 'NONE', #2988, 7.999999999999979572 ) ;
#14963=AXIS2_PLACEMENT_3D ( 'NONE', #5022, #25880, #23730 ) ;
#14964=ADVANCED_FACE ( 'NONE', ( #10762 ), #29971, .T. ) ;
#14965=ORIENTED_EDGE ( 'NONE', *, *, #7247, .T. ) ;
#14968=ADVANCED_FACE ( 'NONE', ( #18607 ), #29452, .T. ) ;
#14975=ADVANCED_FACE ( 'NONE', ( #32280 ), #23913, .F. ) ;
#14978=LINE ( 'NONE', #561, #22088 ) ;
#14982=CARTESIAN_POINT ( 'NONE',  ( 12.00000000000001066, -32.99999999999997158, -175.0000000000000000 ) ) ;
#14986=AXIS2_PLACEMENT_3D ( 'NONE', #22199, #25027, #10821 ) ;
#14987=AXIS2_PLACEMENT_3D ( 'NONE', #12493, #2310, #21892 ) ;
#14988=ORIENTED_EDGE ( 'NONE', *, *, #31444, .F. ) ;
#14990=CARTESIAN_POINT ( 'NONE',  ( 12.00000000000003908, -60.99999999999996447, -154.9999999999999716 ) ) ;
#14994=LINE ( 'NONE', #22296, #20686 ) ;
#14999=ORIENTED_EDGE ( 'NONE', *, *, #6923, .F. ) ;
#15001=ORIENTED_EDGE ( 'NONE', *, *, #8238, .T. ) ;
#15007=ADVANCED_FACE ( 'NONE', ( #29794 ), #5046, .T. ) ;
#15009=EDGE_LOOP ( 'NONE', ( #722, #8253, #1591, #20967 ) ) ;
#15011=VERTEX_POINT ( 'NONE', #5399 ) ;
#15012=CARTESIAN_POINT ( 'NONE',  ( -20.00000000000004619, -105.0000000000000000, -162.9999999999999716 ) ) ;
#15013=ORIENTED_EDGE ( 'NONE', *, *, #8634, .T. ) ;
#15014=CARTESIAN_POINT ( 'NONE',  ( -430.0000000000000000, -131.0000000000000000, 128.0000000000000000 ) ) ;
#15015=CARTESIAN_POINT ( 'NONE',  ( -410.0000000000000568, -105.0000000000000142, 107.9999999999999574 ) ) ;
#15020=LINE ( 'NONE', #14851, #34642 ) ;
#15022=EDGE_CURVE ( 'NONE', #8951, #19693, #32806, .T. ) ;
#15023=CARTESIAN_POINT ( 'NONE',  ( -418.0000000000000000, 137.0000000000000000, 154.9999999999999716 ) ) ;
#15024=ORIENTED_EDGE ( 'NONE', *, *, #4157, .F. ) ;
#15025=DIRECTION ( 'NONE',  ( 1.000000000000000000, 0.000000000000000000, 0.000000000000000000 ) ) ;
#15026=CARTESIAN_POINT ( 'NONE',  ( -499.9999999999999432, 112.9999999999999574, 159.0000000000000000 ) ) ;
#15030=VECTOR ( 'NONE', #30809, 1000.000000000000000 ) ;
#15033=EDGE_CURVE ( 'NONE', #7332, #27667, #10284, .T. ) ;
#15035=ADVANCED_FACE ( 'NONE', ( #27119, #2734 ), #24432, .T. ) ;
#15036=DIRECTION ( 'NONE',  ( 0.000000000000000000, 1.310824597558155437E-49, 1.000000000000000000 ) ) ;
#15037=CARTESIAN_POINT ( 'NONE',  ( -349.0000000000000000, -125.0000000000000284, 164.9999999999999716 ) ) ;
#15038=LINE ( 'NONE', #1836, #8199 ) ;
#15041=AXIS2_PLACEMENT_3D ( 'NONE', #4062, #15653, #20459 ) ;
#15043=ORIENTED_EDGE ( 'NONE', *, *, #817, .F. ) ;
#15045=LINE ( 'NONE', #4666, #25715 ) ;
#15047=VECTOR ( 'NONE', #20992, 1000.000000000000000 ) ;
#15048=EDGE_CURVE ( 'NONE', #34687, #9057, #34160, .T. ) ;
#15049=EDGE_LOOP ( 'NONE', ( #26845, #16334, #1948, #24745 ) ) ;
#15051=ORIENTED_EDGE ( 'NONE', *, *, #34559, .T. ) ;
#15057=ORIENTED_EDGE ( 'NONE', *, *, #4882, .T. ) ;
#15060=CARTESIAN_POINT ( 'NONE',  ( -430.0000000000000000, 130.9999999999999716, 113.9999999999999858 ) ) ;
#15061=AXIS2_PLACEMENT_3D ( 'NONE', #26051, #18234, #1665 ) ;
#15063=PLANE ( 'NONE',  #9725 ) ;
#15070=CARTESIAN_POINT ( 'NONE',  ( 19.99999999999998934, -55.00000000000000711, 162.9999999999999716 ) ) ;
#15073=LINE ( 'NONE', #12926, #9044 ) ;
#15074=VERTEX_POINT ( 'NONE', #8777 ) ;
#15077=EDGE_CURVE ( 'NONE', #3477, #28571, #25144, .T. ) ;
#15081=AXIS2_PLACEMENT_3D ( 'NONE', #15142, #33645, #3563 ) ;
#15082=DIRECTION ( 'NONE',  ( -0.000000000000000000, 1.000000000000000000, -0.000000000000000000 ) ) ;
#15085=DIRECTION ( 'NONE',  ( 0.000000000000000000, 2.309213040847544338E-50, 1.000000000000000000 ) ) ;
#15086=AXIS2_PLACEMENT_3D ( 'NONE', #14937, #25771, #9229 ) ;
#15088=AXIS2_PLACEMENT_3D ( 'NONE', #21190, #23688, #26527 ) ;
#15089=VERTEX_POINT ( 'NONE', #30678 ) ;
#15090=AXIS2_PLACEMENT_3D ( 'NONE', #10869, #13547, #16407 ) ;
#15091=DIRECTION ( 'NONE',  ( 0.000000000000000000, -1.000000000000000000, 0.000000000000000000 ) ) ;
#15092=DIRECTION ( 'NONE',  ( 0.000000000000000000, -0.000000000000000000, 1.000000000000000000 ) ) ;
#15093=ORIENTED_EDGE ( 'NONE', *, *, #18470, .F. ) ;
#15096=ORIENTED_EDGE ( 'NONE', *, *, #6338, .T. ) ;
#15097=CARTESIAN_POINT ( 'NONE',  ( -414.0000000000000568, -112.9999999999999858, 155.0000000000000000 ) ) ;
#15098=CARTESIAN_POINT ( 'NONE',  ( -11.99999999999998224, -134.9999999999999716, 162.9999999999999716 ) ) ;
#15099=CIRCLE ( 'NONE', #29319, 3.999999999999976019 ) ;
#15102=CARTESIAN_POINT ( 'NONE',  ( 19.99999999999998224, 134.9999999999998863, 187.0000000000000000 ) ) ;
#15103=VERTEX_POINT ( 'NONE', #16824 ) ;
#15105=EDGE_LOOP ( 'NONE', ( #16076, #8245, #6526, #11588, #13884, #967, #18844, #26370 ) ) ;
#15109=CIRCLE ( 'NONE', #5979, 7.999999999999979572 ) ;
#15110=CARTESIAN_POINT ( 'NONE',  ( -349.0000000000000000, -135.0000000000000000, 130.0000000000000000 ) ) ;
#15112=CARTESIAN_POINT ( 'NONE',  ( -20.00000000000007461, 112.9999999999999574, 187.0000000000000000 ) ) ;
#15114=FACE_OUTER_BOUND ( 'NONE', #29294, .T. ) ;
#15118=ADVANCED_FACE ( 'NONE', ( #6629, #17529, #31032 ), #430, .F. ) ;
#15122=EDGE_CURVE ( 'NONE', #29489, #11417, #6449, .T. ) ;
#15123=CARTESIAN_POINT ( 'NONE',  ( -418.0000000000000000, -105.0000000000000142, -101.9999999999999858 ) ) ;
#15124=EDGE_LOOP ( 'NONE', ( #33335, #15349, #24122, #6485 ) ) ;
#15133=ORIENTED_EDGE ( 'NONE', *, *, #24986, .T. ) ;
#15141=VERTEX_POINT ( 'NONE', #8600 ) ;
#15142=CARTESIAN_POINT ( 'NONE',  ( 11.99999999999999645, 124.9999999999999716, 190.9999999999999716 ) ) ;
#15146=CARTESIAN_POINT ( 'NONE',  ( -499.9999999999999432, -113.0000000000000000, -190.9999999999999716 ) ) ;
#15147=DIRECTION ( 'NONE',  ( 1.000000000000000000, 0.000000000000000000, 1.300283923313630633E-47 ) ) ;
#15148=VERTEX_POINT ( 'NONE', #13962 ) ;
#15150=DIRECTION ( 'NONE',  ( 1.000000000000000000, 0.000000000000000000, 0.000000000000000000 ) ) ;
#15153=EDGE_CURVE ( 'NONE', #11831, #15331, #24968, .T. ) ;
#15158=EDGE_CURVE ( 'NONE', #34740, #4151, #596, .T. ) ;
#15161=EDGE_CURVE ( 'NONE', #763, #25411, #33513, .T. ) ;
#15164=LINE ( 'NONE', #12845, #14306 ) ;
#15165=DIRECTION ( 'NONE',  ( 0.000000000000000000, -1.000000000000000000, 0.000000000000000000 ) ) ;
#15167=DIRECTION ( 'NONE',  ( -1.000000000000000000, 0.000000000000000000, 0.000000000000000000 ) ) ;
#15171=DIRECTION ( 'NONE',  ( 1.000000000000000000, 0.000000000000000000, 0.000000000000000000 ) ) ;
#15174=EDGE_CURVE ( 'NONE', #18838, #14780, #17351, .T. ) ;
#15182=ORIENTED_EDGE ( 'NONE', *, *, #15886, .T. ) ;
#15186=CARTESIAN_POINT ( 'NONE',  ( -442.0000000000000000, -105.0000000000000142, -101.9999999999999858 ) ) ;
#15188=ORIENTED_EDGE ( 'NONE', *, *, #27429, .T. ) ;
#15189=ORIENTED_EDGE ( 'NONE', *, *, #17735, .F. ) ;
#15193=CARTESIAN_POINT ( 'NONE',  ( -445.9999999999999432, 137.0000000000000000, 154.9999999999999716 ) ) ;
#15194=DIRECTION ( 'NONE',  ( -0.000000000000000000, -0.000000000000000000, -1.000000000000000000 ) ) ;
#15197=VECTOR ( 'NONE', #2006, 1000.000000000000000 ) ;
#15199=FACE_OUTER_BOUND ( 'NONE', #10019, .T. ) ;
#15200=CARTESIAN_POINT ( 'NONE',  ( -449.9999999999999432, 124.9999999999999432, -162.9999999999999716 ) ) ;
#15204=CARTESIAN_POINT ( 'NONE',  ( -430.0000000000000000, 118.9999999999999858, 128.0000000000000000 ) ) ;
#15212=ADVANCED_FACE ( 'NONE', ( #9129 ), #23710, .T. ) ;
#15213=AXIS2_PLACEMENT_3D ( 'NONE', #22181, #296, #19522 ) ;
#15214=CARTESIAN_POINT ( 'NONE',  ( -499.9999999999999432, 108.9999999999999858, 162.9999999999999716 ) ) ;
#15215=ORIENTED_EDGE ( 'NONE', *, *, #11720, .F. ) ;
#15217=DIRECTION ( 'NONE',  ( 0.000000000000000000, 0.000000000000000000, -1.000000000000000000 ) ) ;
#15218=DIRECTION ( 'NONE',  ( 0.000000000000000000, 0.000000000000000000, -1.000000000000000000 ) ) ;
#15222=DIRECTION ( 'NONE',  ( -2.154935995002245207E-17, -0.000000000000000000, -1.000000000000000000 ) ) ;
#15229=ORIENTED_EDGE ( 'NONE', *, *, #23966, .T. ) ;
#15232=AXIS2_PLACEMENT_3D ( 'NONE', #22144, #19308, #13787 ) ;
#15237=ORIENTED_EDGE ( 'NONE', *, *, #12805, .T. ) ;
#15239=DIRECTION ( 'NONE',  ( 1.000000000000000000, 0.000000000000000000, 0.000000000000000000 ) ) ;
#15241=DIRECTION ( 'NONE',  ( -0.000000000000000000, -1.000000000000000000, -0.000000000000000000 ) ) ;
#15242=DIRECTION ( 'NONE',  ( -0.000000000000000000, -1.000000000000000000, -0.000000000000000000 ) ) ;
#15243=DIRECTION ( 'NONE',  ( -0.000000000000000000, -5.053935297177146739E-49, -1.000000000000000000 ) ) ;
#15248=ORIENTED_EDGE ( 'NONE', *, *, #4516, .T. ) ;
#15249=CARTESIAN_POINT ( 'NONE',  ( -349.0000000000000000, 134.9999999999999716, 126.0000000000000000 ) ) ;
#15250=CARTESIAN_POINT ( 'NONE',  ( -12.00000000000001066, -32.99999999999997158, 154.9999999999999716 ) ) ;
#15253=CIRCLE ( 'NONE', #18658, 4.750000000000004441 ) ;
#15255=EDGE_CURVE ( 'NONE', #7431, #30469, #15363, .T. ) ;
#15260=DIRECTION ( 'NONE',  ( 0.000000000000000000, 1.000000000000000000, 0.000000000000000000 ) ) ;
#15262=ADVANCED_FACE ( 'NONE', ( #28701, #9494 ), #20865, .T. ) ;
#15266=CARTESIAN_POINT ( 'NONE',  ( 15.99999999999998579, -32.99999999999997158, 154.9999999999999716 ) ) ;
#15267=ORIENTED_EDGE ( 'NONE', *, *, #2834, .F. ) ;
#15274=ADVANCED_FACE ( 'NONE', ( #29042, #23357, #18389 ), #3953, .F. ) ;
#15279=DIRECTION ( 'NONE',  ( 0.000000000000000000, -1.310824597558155437E-49, -1.000000000000000000 ) ) ;
#15281=ORIENTED_EDGE ( 'NONE', *, *, #11001, .F. ) ;
#15282=ORIENTED_EDGE ( 'NONE', *, *, #3948, .T. ) ;
#15290=ADVANCED_FACE ( 'NONE', ( #31202 ), #12695, .T. ) ;
#15298=VECTOR ( 'NONE', #33923, 1000.000000000000000 ) ;
#15305=DIRECTION ( 'NONE',  ( 0.000000000000000000, -1.000000000000000000, -2.465190328815662439E-32 ) ) ;
#15306=EDGE_CURVE ( 'NONE', #10280, #10318, #7469, .T. ) ;
#15311=VERTEX_POINT ( 'NONE', #15015 ) ;
#15312=EDGE_CURVE ( 'NONE', #16142, #29708, #12344, .T. ) ;
#15314=DIRECTION ( 'NONE',  ( 0.000000000000000000, 0.000000000000000000, 1.000000000000000000 ) ) ;
#15321=CARTESIAN_POINT ( 'NONE',  ( -414.0000000000000568, -137.0000000000000000, -175.0000000000000000 ) ) ;
#15326=ORIENTED_EDGE ( 'NONE', *, *, #2275, .F. ) ;
#15328=EDGE_LOOP ( 'NONE', ( #5345, #12864, #160, #16732 ) ) ;
#15329=DIRECTION ( 'NONE',  ( 1.000000000000000000, 0.000000000000000000, 1.300283923313630633E-47 ) ) ;
#15331=VERTEX_POINT ( 'NONE', #5488 ) ;
#15333=CARTESIAN_POINT ( 'NONE',  ( -12.00000000000001066, 124.9999999999999716, 155.0000000000000000 ) ) ;
#15335=ORIENTED_EDGE ( 'NONE', *, *, #2533, .T. ) ;
#15340=CARTESIAN_POINT ( 'NONE',  ( -19.99999999999998934, 112.9999999999999574, -175.0000000000000284 ) ) ;
#15342=CARTESIAN_POINT ( 'NONE',  ( 19.99999999999998934, -115.0000000000000000, 154.9999999999999716 ) ) ;
#15346=ORIENTED_EDGE ( 'NONE', *, *, #16350, .F. ) ;
#15349=ORIENTED_EDGE ( 'NONE', *, *, #14333, .T. ) ;
#15350=ORIENTED_EDGE ( 'NONE', *, *, #4198, .F. ) ;
#15351=EDGE_CURVE ( 'NONE', #32651, #32967, #5184, .T. ) ;
#15353=EDGE_CURVE ( 'NONE', #14577, #10753, #26552, .T. ) ;
#15354=CARTESIAN_POINT ( 'NONE',  ( -19.99999999999998934, -112.9999999999999858, -155.0000000000000284 ) ) ;
#15358=VERTEX_POINT ( 'NONE', #10356 ) ;
#15359=EDGE_CURVE ( 'NONE', #1031, #19038, #14314, .T. ) ;
#15363=LINE ( 'NONE', #1816, #9195 ) ;
#15364=ORIENTED_EDGE ( 'NONE', *, *, #33541, .T. ) ;
#15365=ORIENTED_EDGE ( 'NONE', *, *, #18428, .T. ) ;
#15370=DIRECTION ( 'NONE',  ( 0.000000000000000000, 0.000000000000000000, -1.000000000000000000 ) ) ;
#15373=VERTEX_POINT ( 'NONE', #3352 ) ;
#15375=DIRECTION ( 'NONE',  ( 1.000000000000000000, 0.000000000000000000, 0.000000000000000000 ) ) ;
#15383=CARTESIAN_POINT ( 'NONE',  ( 0.000000000000000000, -55.00000000000000711, 0.000000000000000000 ) ) ;
#15385=ORIENTED_EDGE ( 'NONE', *, *, #21259, .T. ) ;
#15386=LINE ( 'NONE', #18410, #8738 ) ;
#15389=ORIENTED_EDGE ( 'NONE', *, *, #6463, .F. ) ;
#15390=AXIS2_PLACEMENT_3D ( 'NONE', #29144, #12611, #10105 ) ;
#15396=EDGE_LOOP ( 'NONE', ( #28573, #31485, #22169, #20732 ) ) ;
#15397=ORIENTED_EDGE ( 'NONE', *, *, #29850, .F. ) ;
#15399=CARTESIAN_POINT ( 'NONE',  ( -442.0000000000000000, -124.9999999999999716, 139.9999999999999716 ) ) ;
#15403=DIRECTION ( 'NONE',  ( 0.000000000000000000, 0.000000000000000000, 1.000000000000000000 ) ) ;
#15405=VERTEX_POINT ( 'NONE', #19568 ) ;
#15413=CARTESIAN_POINT ( 'NONE',  ( 11.99999999999999822, -64.99999999999997158, 154.9999999999999716 ) ) ;
#15414=ORIENTED_EDGE ( 'NONE', *, *, #8140, .T. ) ;
#15419=ORIENTED_EDGE ( 'NONE', *, *, #15905, .F. ) ;
#15421=VECTOR ( 'NONE', #30160, 1000.000000000000000 ) ;
#15423=PLANE ( 'NONE',  #20043 ) ;
#15424=CARTESIAN_POINT ( 'NONE',  ( 19.99999999999998934, -124.9999999999999432, -154.9999999999999716 ) ) ;
#15426=CARTESIAN_POINT ( 'NONE',  ( 11.99999999999999645, 144.9999999999999716, 194.9999999999999716 ) ) ;
#15427=ORIENTED_EDGE ( 'NONE', *, *, #16093, .T. ) ;
#15436=ORIENTED_EDGE ( 'NONE', *, *, #27651, .T. ) ;
#15445=DIRECTION ( 'NONE',  ( 0.000000000000000000, 0.000000000000000000, -1.000000000000000000 ) ) ;
#15447=CARTESIAN_POINT ( 'NONE',  ( -500.0000000000000000, -113.0000000000000000, 159.0000000000000000 ) ) ;
#15448=CARTESIAN_POINT ( 'NONE',  ( -499.9999999999999432, 112.9999999999999574, -187.0000000000000000 ) ) ;
#15450=ORIENTED_EDGE ( 'NONE', *, *, #32176, .F. ) ;
#15456=AXIS2_PLACEMENT_3D ( 'NONE', #33604, #28446, #25590 ) ;
#15458=CARTESIAN_POINT ( 'NONE',  ( 11.99999999999999645, -145.0000000000000000, 174.9999999999999432 ) ) ;
#15463=CARTESIAN_POINT ( 'NONE',  ( -365.0000000000000000, -119.0000000000000000, 113.9999999999999858 ) ) ;
#15466=VECTOR ( 'NONE', #19205, 1000.000000000000000 ) ;
#15468=ORIENTED_EDGE ( 'NONE', *, *, #10734, .T. ) ;
#15476=EDGE_CURVE ( 'NONE', #16412, #24248, #27213, .T. ) ;
#15477=DIRECTION ( 'NONE',  ( -0.000000000000000000, 1.000000000000000000, -0.000000000000000000 ) ) ;
#15479=EDGE_CURVE ( 'NONE', #32751, #18201, #25236, .T. ) ;
#15482=CARTESIAN_POINT ( 'NONE',  ( 12.00000000000001066, -134.9999999999999716, 194.9999999999999716 ) ) ;
#15483=ADVANCED_FACE ( 'NONE', ( #9227 ), #1396, .T. ) ;
#15489=DIRECTION ( 'NONE',  ( 0.000000000000000000, 0.000000000000000000, -1.000000000000000000 ) ) ;
#15491=ADVANCED_FACE ( 'NONE', ( #6723, #25951 ), #1046, .T. ) ;
#15492=ORIENTED_EDGE ( 'NONE', *, *, #1248, .T. ) ;
#15495=CARTESIAN_POINT ( 'NONE',  ( -365.0000000000000000, 130.9999999999999716, 126.0000000000000000 ) ) ;
#15496=ORIENTED_EDGE ( 'NONE', *, *, #23991, .F. ) ;
#15497=VERTEX_POINT ( 'NONE', #30595 ) ;
#15501=DIRECTION ( 'NONE',  ( -1.000000000000000000, 0.000000000000000000, 0.000000000000000000 ) ) ;
#15504=ORIENTED_EDGE ( 'NONE', *, *, #27559, .F. ) ;
#15508=EDGE_CURVE ( 'NONE', #17362, #32005, #6186, .T. ) ;
#15511=LINE ( 'NONE', #15340, #33858 ) ;
#15512=EDGE_CURVE ( 'NONE', #11201, #7081, #20097, .T. ) ;
#15514=VECTOR ( 'NONE', #16271, 1000.000000000000000 ) ;
#15521=ORIENTED_EDGE ( 'NONE', *, *, #19745, .F. ) ;
#15523=FACE_OUTER_BOUND ( 'NONE', #11724, .T. ) ;
#15528=DIRECTION ( 'NONE',  ( 0.000000000000000000, 0.000000000000000000, 1.000000000000000000 ) ) ;
#15531=CARTESIAN_POINT ( 'NONE',  ( 11.99999999999999645, 140.9999999999999716, -155.0000000000000000 ) ) ;
#15532=VECTOR ( 'NONE', #6160, 1000.000000000000000 ) ;
#15537=VECTOR ( 'NONE', #32952, 1000.000000000000000 ) ;
#15538=CARTESIAN_POINT ( 'NONE',  ( -500.0000000000000000, -137.0000000000000000, 190.9999999999999716 ) ) ;
#15541=LINE ( 'NONE', #18579, #27331 ) ;
#15544=DIRECTION ( 'NONE',  ( 0.000000000000000000, 0.000000000000000000, -1.000000000000000000 ) ) ;
#15545=CARTESIAN_POINT ( 'NONE',  ( -499.9999999999999432, -113.0000000000000000, -159.0000000000000000 ) ) ;
#15549=CARTESIAN_POINT ( 'NONE',  ( 15.99999999999998579, -55.00000000000000711, -154.9999999999999716 ) ) ;
#15551=ADVANCED_FACE ( 'NONE', ( #33788 ), #30762, .F. ) ;
#15554=EDGE_CURVE ( 'NONE', #12516, #32323, #3524, .T. ) ;
#15556=CARTESIAN_POINT ( 'NONE',  ( -365.0000000000000000, 130.9999999999999716, 111.9999999999999858 ) ) ;
#15566=DIRECTION ( 'NONE',  ( -1.000000000000000000, 0.000000000000000000, 0.000000000000000000 ) ) ;
#15571=DIRECTION ( 'NONE',  ( 0.000000000000000000, -1.000000000000000000, 3.374343856708137958E-53 ) ) ;
#15572=EDGE_LOOP ( 'NONE', ( #21737, #545, #5211, #955 ) ) ;
#15575=CIRCLE ( 'NONE', #28630, 3.999999999999976019 ) ;
#15576=DIRECTION ( 'NONE',  ( 0.000000000000000000, 0.000000000000000000, 1.000000000000000000 ) ) ;
#15577=FACE_OUTER_BOUND ( 'NONE', #22262, .T. ) ;
#15581=CARTESIAN_POINT ( 'NONE',  ( -12.00000000000001066, 144.9999999999999716, 155.0000000000000000 ) ) ;
#15584=DIRECTION ( 'NONE',  ( 1.000000000000000000, 0.000000000000000000, 0.000000000000000000 ) ) ;
#15585=UNCERTAINTY_MEASURE_WITH_UNIT (LENGTH_MEASURE( 1.000000000000000082E-05 ), #5257, 'distance_accuracy_value', 'NONE');
#15586=VERTEX_POINT ( 'NONE', #12443 ) ;
#15588=ORIENTED_EDGE ( 'NONE', *, *, #28908, .T. ) ;
#15589=CARTESIAN_POINT ( 'NONE',  ( -345.0000000000000000, -125.0000000000000284, 168.9999999999999716 ) ) ;
#15593=ORIENTED_EDGE ( 'NONE', *, *, #24746, .F. ) ;
#15600=ORIENTED_EDGE ( 'NONE', *, *, #17732, .F. ) ;
#15601=CARTESIAN_POINT ( 'NONE',  ( -15.99999999999998579, 124.9999999999999716, 162.9999999999999716 ) ) ;
#15604=ORIENTED_EDGE ( 'NONE', *, *, #13932, .T. ) ;
#15608=DIRECTION ( 'NONE',  ( 0.000000000000000000, 1.000000000000000000, -3.374343856708137958E-53 ) ) ;
#15609=VECTOR ( 'NONE', #22923, 1000.000000000000000 ) ;
#15613=LINE ( 'NONE', #9904, #11118 ) ;
#15616=EDGE_LOOP ( 'NONE', ( #6084, #17766, #29454, #13639 ) ) ;
#15625=LINE ( 'NONE', #27156, #23544 ) ;
#15626=CARTESIAN_POINT ( 'NONE',  ( -418.0000000000000000, -137.0000000000000000, 154.9999999999999716 ) ) ;
#15628=DIRECTION ( 'NONE',  ( -1.000000000000000000, 0.000000000000000000, -5.546364386991661285E-52 ) ) ;
#15630=ORIENTED_EDGE ( 'NONE', *, *, #18810, .F. ) ;
#15633=DIRECTION ( 'NONE',  ( 1.000000000000000000, 0.000000000000000000, 0.000000000000000000 ) ) ;
#15637=DIRECTION ( 'NONE',  ( 0.000000000000000000, 1.000000000000000000, 0.000000000000000000 ) ) ;
#15638=CARTESIAN_POINT ( 'NONE',  ( 19.99999999999998934, 136.9999999999999716, -175.0000000000000284 ) ) ;
#15643=DIRECTION ( 'NONE',  ( 1.300283923313630633E-47, 0.000000000000000000, 1.000000000000000000 ) ) ;
#15644=ORIENTED_EDGE ( 'NONE', *, *, #14811, .F. ) ;
#15645=FACE_OUTER_BOUND ( 'NONE', #5392, .T. ) ;
#15647=VECTOR ( 'NONE', #14389, 1000.000000000000000 ) ;
#15648=VECTOR ( 'NONE', #1072, 1000.000000000000000 ) ;
#15652=EDGE_CURVE ( 'NONE', #5999, #27971, #20613, .T. ) ;
#15653=DIRECTION ( 'NONE',  ( 0.000000000000000000, -1.224646799147353207E-16, 1.000000000000000000 ) ) ;
#15655=EDGE_LOOP ( 'NONE', ( #18276, #27368, #10128, #8705, #24856, #21344, #11918, #33224 ) ) ;
#15658=CARTESIAN_POINT ( 'NONE',  ( -20.00000000000007461, 136.9999999999999432, -187.0000000000000000 ) ) ;
#15661=ORIENTED_EDGE ( 'NONE', *, *, #6303, .F. ) ;
#15665=VECTOR ( 'NONE', #29106, 1000.000000000000000 ) ;
#15667=AXIS2_PLACEMENT_3D ( 'NONE', #16340, #29506, #5452 ) ;
#15674=AXIS2_PLACEMENT_3D ( 'NONE', #17034, #14535, #22714 ) ;
#15676=AXIS2_PLACEMENT_3D ( 'NONE', #10948, #32604, #27453 ) ;
#15678=ADVANCED_FACE ( 'NONE', ( #12790 ), #21314, .T. ) ;
#15679=CIRCLE ( 'NONE', #20226, 3.999999999999976019 ) ;
#15683=VERTEX_POINT ( 'NONE', #26648 ) ;
#15686=ORIENTED_EDGE ( 'NONE', *, *, #1128, .F. ) ;
#15695=CARTESIAN_POINT ( 'NONE',  ( -499.9999999999999432, -141.0000000000000000, -187.0000000000000000 ) ) ;
#15697=FACE_OUTER_BOUND ( 'NONE', #31319, .T. ) ;
#15701=CARTESIAN_POINT ( 'NONE',  ( -442.0000000000000000, 105.0000000000000000, 132.0000000000000000 ) ) ;
#15702=DIRECTION ( 'NONE',  ( 5.546364386991661285E-52, 0.000000000000000000, 1.000000000000000000 ) ) ;
#15705=ORIENTED_EDGE ( 'NONE', *, *, #19604, .F. ) ;
#15707=EDGE_LOOP ( 'NONE', ( #27196, #7397, #3147, #18453, #31974, #26827, #30177, #19880 ) ) ;
#15708=VERTEX_POINT ( 'NONE', #13133 ) ;
#15713=VERTEX_POINT ( 'NONE', #2092 ) ;
#15716=EDGE_CURVE ( 'NONE', #1290, #11374, #26822, .T. ) ;
#15721=CARTESIAN_POINT ( 'NONE',  ( 11.99999999999999645, -55.00000000000002132, 162.9999999999999716 ) ) ;
#15724=CARTESIAN_POINT ( 'NONE',  ( -500.0000000000000000, -113.0000000000000000, 162.9999999999999716 ) ) ;
#15732=DIRECTION ( 'NONE',  ( -0.000000000000000000, -1.000000000000000000, -0.000000000000000000 ) ) ;
#15741=AXIS2_PLACEMENT_3D ( 'NONE', #22979, #1437, #33834 ) ;
#15742=CARTESIAN_POINT ( 'NONE',  ( -19.99999999999998934, -56.99999999999997868, -154.9999999999999716 ) ) ;
#15746=LINE ( 'NONE', #23897, #20837 ) ;
#15748=EDGE_LOOP ( 'NONE', ( #23447, #26196 ) ) ;
#15749=DIRECTION ( 'NONE',  ( 0.000000000000000000, -1.224646799147353207E-16, 1.000000000000000000 ) ) ;
#15752=VERTEX_POINT ( 'NONE', #34308 ) ;
#15753=ORIENTED_EDGE ( 'NONE', *, *, #25356, .F. ) ;
#15755=ORIENTED_EDGE ( 'NONE', *, *, #16191, .T. ) ;
#15756=ORIENTED_EDGE ( 'NONE', *, *, #6337, .T. ) ;
#15757=DIRECTION ( 'NONE',  ( 0.000000000000000000, 1.000000000000000000, 1.224646799147353207E-16 ) ) ;
#15759=EDGE_CURVE ( 'NONE', #181, #21502, #31632, .T. ) ;
#15762=EDGE_CURVE ( 'NONE', #9264, #26418, #14191, .T. ) ;
#15763=DIRECTION ( 'NONE',  ( 1.000000000000000000, 3.040835319149746090E-31, 1.232595164407830946E-32 ) ) ;
#15769=DIRECTION ( 'NONE',  ( 1.000000000000000000, 0.000000000000000000, -1.232595164407831220E-32 ) ) ;
#15772=DIRECTION ( 'NONE',  ( 0.000000000000000000, 0.000000000000000000, -1.000000000000000000 ) ) ;
#15774=LINE ( 'NONE', #26254, #7095 ) ;
#15775=PLANE ( 'NONE',  #19294 ) ;
#15777=VECTOR ( 'NONE', #32494, 1000.000000000000000 ) ;
#15778=PLANE ( 'NONE',  #30997 ) ;
#15780=PLANE ( 'NONE',  #34514 ) ;
#15781=VERTEX_POINT ( 'NONE', #5451 ) ;
#15784=CARTESIAN_POINT ( 'NONE',  ( -442.0000000000000000, -104.9999999999999716, -187.0000000000000000 ) ) ;
#15785=ORIENTED_EDGE ( 'NONE', *, *, #9863, .T. ) ;
#15787=CARTESIAN_POINT ( 'NONE',  ( -449.9999999999999432, -125.0000000000000000, -101.9999999999999858 ) ) ;
#15789=CYLINDRICAL_SURFACE ( 'NONE', #32438, 3.999999999999976019 ) ;
#15790=VECTOR ( 'NONE', #7774, 1000.000000000000000 ) ;
#15793=ORIENTED_EDGE ( 'NONE', *, *, #8259, .T. ) ;
#15801=ORIENTED_EDGE ( 'NONE', *, *, #14167, .F. ) ;
#15806=CARTESIAN_POINT ( 'NONE',  ( -449.9999999999999432, -112.9999999999999858, -174.9999999999999716 ) ) ;
#15811=EDGE_LOOP ( 'NONE', ( #9670, #24743, #18620, #31310, #19298, #33459, #14497, #20940 ) ) ;
#15813=ORIENTED_EDGE ( 'NONE', *, *, #18741, .F. ) ;
#15815=EDGE_CURVE ( 'NONE', #14078, #2690, #1245, .T. ) ;
#15818=CIRCLE ( 'NONE', #20350, 4.000000000000003553 ) ;
#15821=CARTESIAN_POINT ( 'NONE',  ( -70.00000000000000000, 4.559999999999908127, 172.9900000000000091 ) ) ;
#15824=CARTESIAN_POINT ( 'NONE',  ( -19.99999999999998934, -134.9999999999999716, 162.9999999999999716 ) ) ;
#15825=EDGE_CURVE ( 'NONE', #17242, #32490, #6837, .T. ) ;
#15828=CARTESIAN_POINT ( 'NONE',  ( -499.9999999999999432, 112.9999999999999574, -194.9999999999999716 ) ) ;
#15830=CARTESIAN_POINT ( 'NONE',  ( -12.00000000000001243, 134.9999999999998863, 194.9999999999999716 ) ) ;
#15834=VECTOR ( 'NONE', #27820, 1000.000000000000000 ) ;
#15837=CARTESIAN_POINT ( 'NONE',  ( -19.99999999999998934, 124.9999999999999716, 162.9999999999999716 ) ) ;
#15838=DIRECTION ( 'NONE',  ( 0.000000000000000000, -1.131431318426415506E-52, -1.000000000000000000 ) ) ;
#15840=VECTOR ( 'NONE', #4254, 1000.000000000000000 ) ;
#15845=ORIENTED_EDGE ( 'NONE', *, *, #26917, .T. ) ;
#15849=CARTESIAN_POINT ( 'NONE',  ( -12.00000000000001066, -56.99999999999997868, -175.0000000000000000 ) ) ;
#15850=CARTESIAN_POINT ( 'NONE',  ( -410.0000000000000568, -137.0000000000000000, -175.0000000000000000 ) ) ;
#15853=EDGE_CURVE ( 'NONE', #11201, #12516, #5205, .T. ) ;
#15854=FACE_OUTER_BOUND ( 'NONE', #7076, .T. ) ;
#15856=CIRCLE ( 'NONE', #11295, 7.999999999999979572 ) ;
#15858=CARTESIAN_POINT ( 'NONE',  ( -12.00000000000001066, 136.9999999999999716, 155.0000000000000000 ) ) ;
#15869=STYLED_ITEM('',(#35254),#10172);
#15870=CARTESIAN_POINT ( 'NONE',  ( -20.00000000000007461, -109.0000000000000142, -162.9999999999999716 ) ) ;
#15882=CARTESIAN_POINT ( 'NONE',  ( -365.0000000000000000, 116.9999999999999858, 126.0000000000000000 ) ) ;
#15884=CARTESIAN_POINT ( 'NONE',  ( -19.99999999999998934, 144.9999999999999716, -162.9999999999999147 ) ) ;
#15886=EDGE_CURVE ( 'NONE', #29470, #8179, #2956, .T. ) ;
#15888=ORIENTED_EDGE ( 'NONE', *, *, #3646, .T. ) ;
#15894=VECTOR ( 'NONE', #11504, 1000.000000000000000 ) ;
#15897=ORIENTED_EDGE ( 'NONE', *, *, #20276, .T. ) ;
#15898=DIRECTION ( 'NONE',  ( -3.469446951953832974E-18, -1.000000000000000000, -7.888609052210116302E-31 ) ) ;
#15902=CARTESIAN_POINT ( 'NONE',  ( 11.99999999999999645, 134.9999999999998863, 187.0000000000000000 ) ) ;
#15904=VERTEX_POINT ( 'NONE', #21489 ) ;
#15905=EDGE_CURVE ( 'NONE', #24475, #26754, #7950, .T. ) ;
#15907=CARTESIAN_POINT ( 'NONE',  ( -12.00000000000001066, 104.9999999999999858, -155.0000000000000000 ) ) ;
#15908=LINE ( 'NONE', #32246, #28882 ) ;
#15912=EDGE_LOOP ( 'NONE', ( #8155, #33149, #24011, #22276 ) ) ;
#15913=LINE ( 'NONE', #29589, #35089 ) ;
#15914=PLANE ( 'NONE',  #898 ) ;
#15915=DIRECTION ( 'NONE',  ( 1.000000000000000000, 0.000000000000000000, 0.000000000000000000 ) ) ;
#15922=LINE ( 'NONE', #24068, #11631 ) ;
#15923=ORIENTED_EDGE ( 'NONE', *, *, #2646, .T. ) ;
#15924=CARTESIAN_POINT ( 'NONE',  ( -355.0000000000000000, -119.0000000000000000, 126.0000000000000000 ) ) ;
#15925=LINE ( 'NONE', #27102, #13230 ) ;
#15926=DIRECTION ( 'NONE',  ( 0.000000000000000000, -6.123233995736766036E-17, -1.000000000000000000 ) ) ;
#15927=ADVANCED_FACE ( 'NONE', ( #1178 ), #6325, .F. ) ;
#15929=EDGE_CURVE ( 'NONE', #16123, #31755, #30727, .T. ) ;
#15930=EDGE_CURVE ( 'NONE', #31987, #4626, #5131, .T. ) ;
#15931=ORIENTED_EDGE ( 'NONE', *, *, #34474, .T. ) ;
#15934=VERTEX_POINT ( 'NONE', #28052 ) ;
#15936=VERTEX_POINT ( 'NONE', #25018 ) ;
#15939=EDGE_LOOP ( 'NONE', ( #118, #31664, #2771, #4168 ) ) ;
#15940=LINE ( 'NONE', #8246, #8218 ) ;
#15943=ORIENTED_EDGE ( 'NONE', *, *, #5837, .F. ) ;
#15950=LINE ( 'NONE', #21089, #28706 ) ;
#15952=ORIENTED_EDGE ( 'NONE', *, *, #26292, .T. ) ;
#15953=DIRECTION ( 'NONE',  ( 0.000000000000000000, -0.000000000000000000, 1.000000000000000000 ) ) ;
#15955=CYLINDRICAL_SURFACE ( 'NONE', #8932, 7.999999999999986677 ) ;
#15958=ORIENTED_EDGE ( 'NONE', *, *, #17021, .F. ) ;
#15962=CARTESIAN_POINT ( 'NONE',  ( -19.99999999999998934, 134.9999999999999432, -186.9999999999999716 ) ) ;
#15965=EDGE_LOOP ( 'NONE', ( #25370, #5817, #10126, #12329 ) ) ;
#15968=ORIENTED_EDGE ( 'NONE', *, *, #1055, .F. ) ;
#15969=AXIS2_PLACEMENT_3D ( 'NONE', #31798, #7406, #2778 ) ;
#15973=ORIENTED_EDGE ( 'NONE', *, *, #3603, .T. ) ;
#15977=VECTOR ( 'NONE', #23364, 1000.000000000000000 ) ;
#15979=ORIENTED_EDGE ( 'NONE', *, *, #25205, .F. ) ;
#15982=ORIENTED_EDGE ( 'NONE', *, *, #13540, .F. ) ;
#15993=CARTESIAN_POINT ( 'NONE',  ( -410.0000000000000568, 137.0000000000000000, 154.9999999999999716 ) ) ;
#15995=VERTEX_POINT ( 'NONE', #3662 ) ;
#16000=FACE_OUTER_BOUND ( 'NONE', #5485, .T. ) ;
#16001=ADVANCED_FACE ( 'NONE', ( #27870 ), #17228, .T. ) ;
#16002=VECTOR ( 'NONE', #3004, 1000.000000000000000 ) ;
#16004=LINE ( 'NONE', #26842, #14893 ) ;
#16005=AXIS2_PLACEMENT_3D ( 'NONE', #10075, #10250, #1373 ) ;
#16006=FACE_BOUND ( 'NONE', #17913, .T. ) ;
#16008=CARTESIAN_POINT ( 'NONE',  ( -11.99999999999998224, -145.0000000000000000, 155.0000000000000000 ) ) ;
#16014=AXIS2_PLACEMENT_3D ( 'NONE', #34, #13225, #2868 ) ;
#16015=VERTEX_POINT ( 'NONE', #20059 ) ;
#16023=CYLINDRICAL_SURFACE ( 'NONE', #16913, 8.000000000000007105 ) ;
#16026=CIRCLE ( 'NONE', #23400, 3.999999999999948042 ) ;
#16027=ORIENTED_EDGE ( 'NONE', *, *, #4049, .F. ) ;
#16030=AXIS2_PLACEMENT_3D ( 'NONE', #28948, #17598, #26101 ) ;
#16031=ORIENTED_EDGE ( 'NONE', *, *, #2205, .T. ) ;
#16032=AXIS2_PLACEMENT_3D ( 'NONE', #11857, #11318, #19510 ) ;
#16034=DIRECTION ( 'NONE',  ( 0.000000000000000000, 0.000000000000000000, -1.000000000000000000 ) ) ;
#16041=DIRECTION ( 'NONE',  ( 0.000000000000000000, 0.000000000000000000, 1.000000000000000000 ) ) ;
#16050=EDGE_CURVE ( 'NONE', #19987, #21251, #16550, .T. ) ;
#16051=EDGE_CURVE ( 'NONE', #23168, #32120, #1190, .T. ) ;
#16057=CARTESIAN_POINT ( 'NONE',  ( -365.0000000000000000, -114.9999999999999858, 113.9999999999999858 ) ) ;
#16060=ORIENTED_EDGE ( 'NONE', *, *, #1243, .T. ) ;
#16062=EDGE_CURVE ( 'NONE', #31793, #8977, #17697, .T. ) ;
#16063=CARTESIAN_POINT ( 'NONE',  ( -12.00000000000001066, -105.0000000000000142, 174.9999999999999432 ) ) ;
#16065=VERTEX_POINT ( 'NONE', #9882 ) ;
#16066=LINE ( 'NONE', #31706, #16226 ) ;
#16067=( NAMED_UNIT ( * ) PLANE_ANGLE_UNIT ( ) SI_UNIT ( $, .RADIAN. ) );
#16068=CARTESIAN_POINT ( 'NONE',  ( -499.9999999999999432, -105.0000000000000142, -187.0000000000000000 ) ) ;
#16069=ORIENTED_EDGE ( 'NONE', *, *, #32870, .F. ) ;
#16074=CARTESIAN_POINT ( 'NONE',  ( 19.99999999999998934, 136.9999999999999716, 155.0000000000000000 ) ) ;
#16076=ORIENTED_EDGE ( 'NONE', *, *, #4972, .T. ) ;
#16078=FACE_BOUND ( 'NONE', #12463, .T. ) ;
#16080=DIRECTION ( 'NONE',  ( 1.000000000000000000, -0.000000000000000000, -0.000000000000000000 ) ) ;
#16081=AXIS2_PLACEMENT_3D ( 'NONE', #1234, #30780, #6906 ) ;
#16084=CARTESIAN_POINT ( 'NONE',  ( -19.99999999999998934, -145.0000000000000000, -162.9999999999999432 ) ) ;
#16085=DIRECTION ( 'NONE',  ( 0.000000000000000000, 2.309213040847544338E-50, 1.000000000000000000 ) ) ;
#16089=ORIENTED_EDGE ( 'NONE', *, *, #15351, .T. ) ;
#16090=CARTESIAN_POINT ( 'NONE',  ( -445.9999999999999432, -104.9999999999999716, -187.0000000000000000 ) ) ;
#16092=FACE_OUTER_BOUND ( 'NONE', #20750, .T. ) ;
#16093=EDGE_CURVE ( 'NONE', #2574, #23168, #4692, .T. ) ;
#16097=CARTESIAN_POINT ( 'NONE',  ( -12.00000000000006573, -145.0000000000000000, -194.9999999999999432 ) ) ;
#16100=VECTOR ( 'NONE', #14908, 1000.000000000000000 ) ;
#16101=VECTOR ( 'NONE', #27412, 1000.000000000000000 ) ;
#16102=VECTOR ( 'NONE', #23044, 1000.000000000000000 ) ;
#16108=EDGE_CURVE ( 'NONE', #29515, #30502, #29023, .T. ) ;
#16110=CARTESIAN_POINT ( 'NONE',  ( -12.00000000000001066, -112.9999999999999858, 174.9999999999999432 ) ) ;
#16112=ORIENTED_EDGE ( 'NONE', *, *, #11590, .T. ) ;
#16113=DIRECTION ( 'NONE',  ( 0.000000000000000000, 1.000000000000000000, -3.421138828918010427E-49 ) ) ;
#16114=CARTESIAN_POINT ( 'NONE',  ( -418.0000000000000568, 104.9999999999999858, -155.0000000000000000 ) ) ;
#16118=ORIENTED_EDGE ( 'NONE', *, *, #5135, .F. ) ;
#16119=EDGE_CURVE ( 'NONE', #9803, #8292, #13687, .T. ) ;
#16121=CIRCLE ( 'NONE', #13821, 8.000000000000007105 ) ;
#16122=FACE_OUTER_BOUND ( 'NONE', #25800, .T. ) ;
#16123=VERTEX_POINT ( 'NONE', #4354 ) ;
#16124=DIRECTION ( 'NONE',  ( 1.000000000000000000, 3.469446951953834515E-18, 0.000000000000000000 ) ) ;
#16127=CARTESIAN_POINT ( 'NONE',  ( -445.9999999999999432, 105.0000000000000142, 107.9999999999999858 ) ) ;
#16134=VERTEX_POINT ( 'NONE', #31593 ) ;
#16135=CARTESIAN_POINT ( 'NONE',  ( -70.00000000000000000, 75.55999999999990280, 168.2400000000000091 ) ) ;
#16138=ORIENTED_EDGE ( 'NONE', *, *, #18289, .F. ) ;
#16140=LINE ( 'NONE', #5594, #30209 ) ;
#16142=VERTEX_POINT ( 'NONE', #15413 ) ;
#16143=VECTOR ( 'NONE', #3164, 1000.000000000000000 ) ;
#16144=ORIENTED_EDGE ( 'NONE', *, *, #15077, .F. ) ;
#16145=CARTESIAN_POINT ( 'NONE',  ( -20.00000000000007461, 108.9999999999999858, -187.0000000000000000 ) ) ;
#16146=CARTESIAN_POINT ( 'NONE',  ( 12.00000000000001066, 104.9999999999999858, 155.0000000000000000 ) ) ;
#16152=DIRECTION ( 'NONE',  ( -1.000000000000000000, 0.000000000000000000, 1.848892746611746966E-32 ) ) ;
#16153=EDGE_LOOP ( 'NONE', ( #24360, #10247, #15705, #5906 ) ) ;
#16154=ORIENTED_EDGE ( 'NONE', *, *, #17416, .T. ) ;
#16155=AXIS2_PLACEMENT_3D ( 'NONE', #31142, #17984, #14952 ) ;
#16157=ORIENTED_EDGE ( 'NONE', *, *, #20566, .F. ) ;
#16158=DIRECTION ( 'NONE',  ( 0.000000000000000000, 0.000000000000000000, -1.000000000000000000 ) ) ;
#16160=DIRECTION ( 'NONE',  ( -3.040835319149746090E-31, -1.000000000000000000, 0.000000000000000000 ) ) ;
#16161=ADVANCED_FACE ( 'NONE', ( #23589 ), #10062, .F. ) ;
#16165=CARTESIAN_POINT ( 'NONE',  ( -349.0000000000000000, 124.9999999999999432, 183.0000000000000000 ) ) ;
#16167=EDGE_LOOP ( 'NONE', ( #29325, #10992, #33731, #5598 ) ) ;
#16172=CIRCLE ( 'NONE', #248, 3.999999999999976019 ) ;
#16173=EDGE_CURVE ( 'NONE', #2443, #7332, #32116, .T. ) ;
#16174=DIRECTION ( 'NONE',  ( 1.000000000000000000, 0.000000000000000000, 0.000000000000000000 ) ) ;
#16179=ORIENTED_EDGE ( 'NONE', *, *, #26034, .T. ) ;
#16182=VECTOR ( 'NONE', #20500, 1000.000000000000000 ) ;
#16184=DIRECTION ( 'NONE',  ( 0.000000000000000000, 0.000000000000000000, 1.000000000000000000 ) ) ;
#16185=DIRECTION ( 'NONE',  ( 0.000000000000000000, 0.000000000000000000, -1.000000000000000000 ) ) ;
#16187=ORIENTED_EDGE ( 'NONE', *, *, #4357, .F. ) ;
#16188=ORIENTED_EDGE ( 'NONE', *, *, #14033, .T. ) ;
#16191=EDGE_CURVE ( 'NONE', #14883, #6316, #31312, .T. ) ;
#16192=ORIENTED_EDGE ( 'NONE', *, *, #4198, .T. ) ;
#16193=DIRECTION ( 'NONE',  ( -1.000000000000000000, 0.000000000000000000, 1.232595164407831220E-32 ) ) ;
#16199=ORIENTED_EDGE ( 'NONE', *, *, #27408, .T. ) ;
#16201=VECTOR ( 'NONE', #25420, 1000.000000000000000 ) ;
#16202=EDGE_CURVE ( 'NONE', #13771, #7322, #21074, .T. ) ;
#16205=ADVANCED_FACE ( 'NONE', ( #1865 ), #2048, .T. ) ;
#16215=CARTESIAN_POINT ( 'NONE',  ( -349.0000000000000000, -125.0000000000000284, 181.0000000000000000 ) ) ;
#16216=DIRECTION ( 'NONE',  ( 1.000000000000000000, 0.000000000000000000, 0.000000000000000000 ) ) ;
#16217=EDGE_LOOP ( 'NONE', ( #14259, #34617, #25995, #3887, #20465, #22510, #14510, #17171 ) ) ;
#16218=ORIENTED_EDGE ( 'NONE', *, *, #24293, .T. ) ;
#16220=CARTESIAN_POINT ( 'NONE',  ( -500.0000000000000000, -145.0000000000000000, -155.0000000000000000 ) ) ;
#16221=VERTEX_POINT ( 'NONE', #21087 ) ;
#16222=CARTESIAN_POINT ( 'NONE',  ( 19.99999999999998934, 4.559999999999908127, 172.9900000000000091 ) ) ;
#16224=CARTESIAN_POINT ( 'NONE',  ( 11.99999999999999645, -124.9999999999999432, -194.9999999999999432 ) ) ;
#16225=CARTESIAN_POINT ( 'NONE',  ( -15.99999999999998579, -32.99999999999997158, 154.9999999999999716 ) ) ;
#16226=VECTOR ( 'NONE', #10719, 1000.000000000000000 ) ;
#16233=VECTOR ( 'NONE', #16532, 1000.000000000000000 ) ;
#16235=VERTEX_POINT ( 'NONE', #7547 ) ;
#16240=EDGE_CURVE ( 'NONE', #7312, #493, #18438, .T. ) ;
#16243=CARTESIAN_POINT ( 'NONE',  ( -418.0000000000000000, -145.0000000000000000, 155.0000000000000000 ) ) ;
#16245=VECTOR ( 'NONE', #8827, 1000.000000000000000 ) ;
#16246=ADVANCED_FACE ( 'NONE', ( #34984 ), #19311, .T. ) ;
#16247=DIRECTION ( 'NONE',  ( 0.000000000000000000, -1.000000000000000000, -5.053935297177146739E-49 ) ) ;
#16248=VERTEX_POINT ( 'NONE', #21617 ) ;
#16251=DIRECTION ( 'NONE',  ( -0.000000000000000000, 1.000000000000000000, -0.000000000000000000 ) ) ;
#16253=VECTOR ( 'NONE', #21446, 1000.000000000000000 ) ;
#16257=VERTEX_POINT ( 'NONE', #2741 ) ;
#16258=FACE_BOUND ( 'NONE', #15748, .T. ) ;
#16259=LINE ( 'NONE', #24409, #27054 ) ;
#16261=VECTOR ( 'NONE', #5024, 1000.000000000000000 ) ;
#16262=CARTESIAN_POINT ( 'NONE',  ( -418.0000000000000000, -109.0000000000000142, -174.9999999999999716 ) ) ;
#16271=DIRECTION ( 'NONE',  ( 0.000000000000000000, 0.000000000000000000, 1.000000000000000000 ) ) ;
#16272=CARTESIAN_POINT ( 'NONE',  ( 15.99999999999998579, -115.0000000000000000, -155.0000000000000284 ) ) ;
#16284=CIRCLE ( 'NONE', #26482, 3.999999999999976019 ) ;
#16286=DIRECTION ( 'NONE',  ( 0.000000000000000000, 2.309213040847544338E-50, 1.000000000000000000 ) ) ;
#16289=ORIENTED_EDGE ( 'NONE', *, *, #8899, .F. ) ;
#16296=ORIENTED_EDGE ( 'NONE', *, *, #32344, .T. ) ;
#16300=EDGE_CURVE ( 'NONE', #19582, #8355, #13440, .T. ) ;
#16302=ORIENTED_EDGE ( 'NONE', *, *, #10376, .F. ) ;
#16304=DIRECTION ( 'NONE',  ( 1.000000000000000000, 0.000000000000000000, -1.232595164407831220E-32 ) ) ;
#16306=LINE ( 'NONE', #16478, #34867 ) ;
#16311=DIRECTION ( 'NONE',  ( 1.000000000000000000, -0.000000000000000000, -0.000000000000000000 ) ) ;
#16314=MECHANICAL_DESIGN_GEOMETRIC_PRESENTATION_REPRESENTATION('',(#7178),#31631);
#16315=ADVANCED_FACE ( 'NONE', ( #22470 ), #19141, .F. ) ;
#16317=DIRECTION ( 'NONE',  ( 0.000000000000000000, 0.000000000000000000, -1.000000000000000000 ) ) ;
#16319=CIRCLE ( 'NONE', #10051, 3.999999999999976019 ) ;
#16322=VECTOR ( 'NONE', #32904, 1000.000000000000000 ) ;
#16328=ORIENTED_EDGE ( 'NONE', *, *, #1546, .F. ) ;
#16329=PLANE ( 'NONE',  #12766 ) ;
#16330=CARTESIAN_POINT ( 'NONE',  ( 15.99999999999998579, 75.55999999999990280, 177.7400000000000091 ) ) ;
#16334=ORIENTED_EDGE ( 'NONE', *, *, #8334, .T. ) ;
#16336=CARTESIAN_POINT ( 'NONE',  ( -19.99999999999998934, 75.55999999999990280, -177.7400000000000091 ) ) ;
#16338=CARTESIAN_POINT ( 'NONE',  ( -410.0000000000000568, 105.0000000000000142, 107.9999999999999858 ) ) ;
#16339=DIRECTION ( 'NONE',  ( 0.000000000000000000, 0.000000000000000000, -1.000000000000000000 ) ) ;
#16340=CARTESIAN_POINT ( 'NONE',  ( 11.99999999999999645, -115.0000000000000000, 162.9999999999999716 ) ) ;
#16349=DIRECTION ( 'NONE',  ( 0.000000000000000000, -2.309213040847544338E-50, -1.000000000000000000 ) ) ;
#16350=EDGE_CURVE ( 'NONE', #842, #15934, #19391, .T. ) ;
#16352=VERTEX_POINT ( 'NONE', #27480 ) ;
#16353=AXIS2_PLACEMENT_3D ( 'NONE', #13576, #24408, #24237 ) ;
#16355=DIRECTION ( 'NONE',  ( 0.000000000000000000, 0.000000000000000000, -1.000000000000000000 ) ) ;
#16356=ORIENTED_EDGE ( 'NONE', *, *, #34112, .F. ) ;
#16358=DIRECTION ( 'NONE',  ( -0.000000000000000000, -1.000000000000000000, -0.000000000000000000 ) ) ;
#16368=AXIS2_PLACEMENT_3D ( 'NONE', #203, #23917, #19266 ) ;
#16371=ORIENTED_EDGE ( 'NONE', *, *, #17468, .T. ) ;
#16372=DIRECTION ( 'NONE',  ( 0.000000000000000000, 0.000000000000000000, -1.000000000000000000 ) ) ;
#16373=EDGE_CURVE ( 'NONE', #21039, #20858, #6107, .T. ) ;
#16374=FACE_OUTER_BOUND ( 'NONE', #34841, .T. ) ;
#16375=AXIS2_PLACEMENT_3D ( 'NONE', #27202, #16193, #34691 ) ;
#16376=CIRCLE ( 'NONE', #1020, 3.999999999999982681 ) ;
#16384=DIRECTION ( 'NONE',  ( -1.000000000000000000, 0.000000000000000000, 0.000000000000000000 ) ) ;
#16390=DIRECTION ( 'NONE',  ( -1.000000000000000000, 0.000000000000000000, 0.000000000000000000 ) ) ;
#16393=CYLINDRICAL_SURFACE ( 'NONE', #33047, 4.000000000000003553 ) ;
#16395=ORIENTED_EDGE ( 'NONE', *, *, #31183, .T. ) ;
#16398=DIRECTION ( 'NONE',  ( 0.000000000000000000, 0.000000000000000000, 1.000000000000000000 ) ) ;
#16403=CARTESIAN_POINT ( 'NONE',  ( 15.99999999999998579, -115.0000000000000142, 162.9999999999999716 ) ) ;
#16404=AXIS2_PLACEMENT_3D ( 'NONE', #5323, #13365, #27400 ) ;
#16405=VECTOR ( 'NONE', #17482, 1000.000000000000000 ) ;
#16407=DIRECTION ( 'NONE',  ( 0.000000000000000000, 0.000000000000000000, -1.000000000000000000 ) ) ;
#16408=DIRECTION ( 'NONE',  ( 0.000000000000000000, 1.000000000000000000, -3.374343856708137958E-53 ) ) ;
#16409=CIRCLE ( 'NONE', #26065, 8.000000000000007105 ) ;
#16412=VERTEX_POINT ( 'NONE', #30513 ) ;
#16419=SHAPE_DEFINITION_REPRESENTATION ( #11796, #47 ) ;
#16424=DIRECTION ( 'NONE',  ( 0.000000000000000000, 1.000000000000000000, 0.000000000000000000 ) ) ;
#16432=ORIENTED_EDGE ( 'NONE', *, *, #15122, .F. ) ;
#16435=FACE_OUTER_BOUND ( 'NONE', #35051, .T. ) ;
#16436=DIRECTION ( 'NONE',  ( -0.000000000000000000, 0.000000000000000000, 1.000000000000000000 ) ) ;
#16440=DIRECTION ( 'NONE',  ( 1.000000000000000000, 0.000000000000000000, 0.000000000000000000 ) ) ;
#16442=AXIS2_PLACEMENT_3D ( 'NONE', #17926, #6849, #28751 ) ;
#16444=VERTEX_POINT ( 'NONE', #22852 ) ;
#16446=CARTESIAN_POINT ( 'NONE',  ( -12.00000000000001066, -28.99999999999999645, 155.0000000000000000 ) ) ;
#16449=AXIS2_PLACEMENT_3D ( 'NONE', #15060, #10800, #32493 ) ;
#16450=ADVANCED_FACE ( 'NONE', ( #3615 ), #5928, .T. ) ;
#16453=EDGE_CURVE ( 'NONE', #28489, #24869, #12184, .T. ) ;
#16454=VERTEX_POINT ( 'NONE', #33168 ) ;
#16457=LINE ( 'NONE', #32275, #8205 ) ;
#16458=ORIENTED_EDGE ( 'NONE', *, *, #16564, .F. ) ;
#16462=AXIS2_PLACEMENT_3D ( 'NONE', #26773, #18784, #2387 ) ;
#16463=PLANE ( 'NONE',  #2720 ) ;
#16465=ORIENTED_EDGE ( 'NONE', *, *, #2644, .T. ) ;
#16466=ORIENTED_EDGE ( 'NONE', *, *, #4803, .T. ) ;
#16467=PLANE ( 'NONE',  #12288 ) ;
#16471=EDGE_LOOP ( 'NONE', ( #27776, #10490, #20105, #18180 ) ) ;
#16472=MECHANICAL_DESIGN_GEOMETRIC_PRESENTATION_REPRESENTATION('',(#30077),#2799);
#16473=LINE ( 'NONE', #13791, #11141 ) ;
#16478=CARTESIAN_POINT ( 'NONE',  ( -442.0000000000000000, 141.0000000000000000, -155.0000000000000000 ) ) ;
#16479=VECTOR ( 'NONE', #8860, 1000.000000000000000 ) ;
#16480=DIRECTION ( 'NONE',  ( 0.000000000000000000, 0.000000000000000000, -1.000000000000000000 ) ) ;
#16485=LINE ( 'NONE', #13801, #10294 ) ;
#16489=CIRCLE ( 'NONE', #24331, 4.000000000000003553 ) ;
#16493=ADVANCED_FACE ( 'NONE', ( #33882 ), #25154, .T. ) ;
#16496=EDGE_CURVE ( 'NONE', #13672, #30715, #14327, .T. ) ;
#16497=ADVANCED_FACE ( 'NONE', ( #22504, #14146 ), #783, .T. ) ;
#16498=VERTEX_POINT ( 'NONE', #11653 ) ;
#16502=ORIENTED_EDGE ( 'NONE', *, *, #22, .F. ) ;
#16512=DIRECTION ( 'NONE',  ( 0.000000000000000000, 0.000000000000000000, -1.000000000000000000 ) ) ;
#16519=ORIENTED_EDGE ( 'NONE', *, *, #19745, .T. ) ;
#16520=DIRECTION ( 'NONE',  ( 0.000000000000000000, 0.000000000000000000, -1.000000000000000000 ) ) ;
#16522=CARTESIAN_POINT ( 'NONE',  ( -414.0000000000000568, 105.0000000000000142, 187.0000000000000000 ) ) ;
#16529=AXIS2_PLACEMENT_3D ( 'NONE', #18997, #24840, #21648 ) ;
#16531=CARTESIAN_POINT ( 'NONE',  ( -70.00000000000000000, 75.55999999999990280, -168.2400000000000091 ) ) ;
#16532=DIRECTION ( 'NONE',  ( 0.000000000000000000, 1.000000000000000000, -3.374343856708137958E-53 ) ) ;
#16535=ORIENTED_EDGE ( 'NONE', *, *, #240, .T. ) ;
#16545=DIRECTION ( 'NONE',  ( -1.232595164407830946E-32, -3.421138828918010427E-49, 1.000000000000000000 ) ) ;
#16546=CARTESIAN_POINT ( 'NONE',  ( -499.9999999999999432, -141.0000000000000000, -162.9999999999999716 ) ) ;
#16547=VERTEX_POINT ( 'NONE', #34403 ) ;
#16549=ORIENTED_EDGE ( 'NONE', *, *, #10492, .F. ) ;
#16550=CIRCLE ( 'NONE', #25619, 8.000000000000007105 ) ;
#16551=CYLINDRICAL_SURFACE ( 'NONE', #20306, 4.000000000000003553 ) ;
#16554=CIRCLE ( 'NONE', #19394, 7.999999999999979572 ) ;
#16557=ORIENTED_EDGE ( 'NONE', *, *, #68, .F. ) ;
#16558=DIRECTION ( 'NONE',  ( 0.000000000000000000, 0.000000000000000000, -1.000000000000000000 ) ) ;
#16560=ADVANCED_FACE ( 'NONE', ( #34579 ), #12522, .T. ) ;
#16564=EDGE_CURVE ( 'NONE', #30135, #24825, #5733, .T. ) ;
#16568=VECTOR ( 'NONE', #27260, 1000.000000000000000 ) ;
#16569=CIRCLE ( 'NONE', #26216, 7.999999999999979572 ) ;
#16570=CIRCLE ( 'NONE', #25638, 7.999999999999979572 ) ;
#16573=FACE_OUTER_BOUND ( 'NONE', #32992, .T. ) ;
#16576=DIRECTION ( 'NONE',  ( -0.000000000000000000, 1.000000000000000000, -0.000000000000000000 ) ) ;
#16578=CARTESIAN_POINT ( 'NONE',  ( -500.0000000000000000, -113.0000000000000000, 187.0000000000000000 ) ) ;
#16580=DIRECTION ( 'NONE',  ( 0.000000000000000000, 1.131431318426415506E-52, 1.000000000000000000 ) ) ;
#16582=EDGE_LOOP ( 'NONE', ( #32092, #18664, #21997, #2248 ) ) ;
#16587=ORIENTED_EDGE ( 'NONE', *, *, #19110, .F. ) ;
#16588=VECTOR ( 'NONE', #19060, 1000.000000000000000 ) ;
#16591=AXIS2_PLACEMENT_3D ( 'NONE', #9568, #18285, #12421 ) ;
#16595=CARTESIAN_POINT ( 'NONE',  ( -445.9999999999999432, -137.0000000000000000, -175.0000000000000000 ) ) ;
#16596=DIRECTION ( 'NONE',  ( -1.000000000000000000, 0.000000000000000000, -0.000000000000000000 ) ) ;
#16597=CARTESIAN_POINT ( 'NONE',  ( -500.0000000000000000, -113.0000000000000000, 190.9999999999999716 ) ) ;
#16601=CARTESIAN_POINT ( 'NONE',  ( 11.99999999999999645, 134.9999999999998863, 162.9999999999999716 ) ) ;
#16602=EDGE_CURVE ( 'NONE', #6498, #1469, #7153, .T. ) ;
#16603=CARTESIAN_POINT ( 'NONE',  ( -499.9999999999999432, -141.0000000000000000, -187.0000000000000000 ) ) ;
#16605=FACE_OUTER_BOUND ( 'NONE', #30912, .T. ) ;
#16618=PLANE ( 'NONE',  #10503 ) ;
#16620=VECTOR ( 'NONE', #12618, 1000.000000000000000 ) ;
#16631=CYLINDRICAL_SURFACE ( 'NONE', #34930, 7.999999999999992895 ) ;
#16636=AXIS2_PLACEMENT_3D ( 'NONE', #33241, #17067, #32522 ) ;
#16641=CIRCLE ( 'NONE', #9257, 2.000000000000001776 ) ;
#16642=VERTEX_POINT ( 'NONE', #18222 ) ;
#16645=EDGE_CURVE ( 'NONE', #13606, #32956, #33602, .T. ) ;
#16647=DIRECTION ( 'NONE',  ( 0.000000000000000000, 0.000000000000000000, 1.000000000000000000 ) ) ;
#16648=ORIENTED_EDGE ( 'NONE', *, *, #7608, .F. ) ;
#16649=EDGE_CURVE ( 'NONE', #30837, #17242, #17878, .T. ) ;
#16650=CARTESIAN_POINT ( 'NONE',  ( -12.00000000000001066, -145.0000000000000000, 162.9999999999999716 ) ) ;
#16654=DIRECTION ( 'NONE',  ( 1.000000000000000000, 0.000000000000000000, 0.000000000000000000 ) ) ;
#16655=CARTESIAN_POINT ( 'NONE',  ( 11.99999999999999645, 104.9999999999999858, -155.0000000000000000 ) ) ;
#16658=ORIENTED_EDGE ( 'NONE', *, *, #27703, .T. ) ;
#16662=( NAMED_UNIT ( * ) PLANE_ANGLE_UNIT ( ) SI_UNIT ( $, .RADIAN. ) );
#16664=VECTOR ( 'NONE', #12807, 1000.000000000000000 ) ;
#16666=AXIS2_PLACEMENT_3D ( 'NONE', #11097, #25126, #22300 ) ;
#16667=AXIS2_PLACEMENT_3D ( 'NONE', #7922, #19321, #32991 ) ;
#16668=CARTESIAN_POINT ( 'NONE',  ( 11.99999999999999645, -124.9999999999999432, -186.9999999999999716 ) ) ;
#16669=CARTESIAN_POINT ( 'NONE',  ( -12.00000000000001066, -124.9999999999999432, -186.9999999999999716 ) ) ;
#16673=LINE ( 'NONE', #5599, #13506 ) ;
#16676=ORIENTED_EDGE ( 'NONE', *, *, #30089, .F. ) ;
#16681=EDGE_LOOP ( 'NONE', ( #27465, #34153, #14745, #3462 ) ) ;
#16683=EDGE_CURVE ( 'NONE', #29789, #7256, #29587, .T. ) ;
#16684=DIRECTION ( 'NONE',  ( -1.000000000000000000, 0.000000000000000000, 0.000000000000000000 ) ) ;
#16690=LINE ( 'NONE', #2957, #13959 ) ;
#16691=AXIS2_PLACEMENT_3D ( 'NONE', #23937, #31946, #4709 ) ;
#16692=CARTESIAN_POINT ( 'NONE',  ( -442.0000000000000000, 124.9999999999999432, -159.0000000000000000 ) ) ;
#16694=LINE ( 'NONE', #34856, #30056 ) ;
#16695=EDGE_LOOP ( 'NONE', ( #30626, #12827, #11616, #5779, #9876, #23620, #19553, #9633 ) ) ;
#16699=LINE ( 'NONE', #24673, #10958 ) ;
#16702=CARTESIAN_POINT ( 'NONE',  ( -499.9999999999999432, -137.0000000000000000, -155.0000000000000000 ) ) ;
#16703=VERTEX_POINT ( 'NONE', #7868 ) ;
#16711=DIRECTION ( 'NONE',  ( -0.000000000000000000, -0.000000000000000000, -1.000000000000000000 ) ) ;
#16712=CARTESIAN_POINT ( 'NONE',  ( -12.00000000000001066, -124.9999999999999432, -154.9999999999999716 ) ) ;
#16717=VECTOR ( 'NONE', #5504, 1000.000000000000000 ) ;
#16718=DIRECTION ( 'NONE',  ( -1.000000000000000000, 0.000000000000000000, -5.546364386991661285E-52 ) ) ;
#16719=ORIENTED_EDGE ( 'NONE', *, *, #5797, .T. ) ;
#16721=( LENGTH_UNIT ( ) NAMED_UNIT ( * ) SI_UNIT ( .MILLI., .METRE. ) );
#16722=CARTESIAN_POINT ( 'NONE',  ( -442.0000000000000000, 137.0000000000000000, 154.9999999999999716 ) ) ;
#16726=ORIENTED_EDGE ( 'NONE', *, *, #24817, .T. ) ;
#16732=ORIENTED_EDGE ( 'NONE', *, *, #21307, .T. ) ;
#16733=ORIENTED_EDGE ( 'NONE', *, *, #15930, .F. ) ;
#16735=ORIENTED_EDGE ( 'NONE', *, *, #3989, .F. ) ;
#16736=DIRECTION ( 'NONE',  ( -1.000000000000000000, -3.469446951953834515E-18, 0.000000000000000000 ) ) ;
#16743=ADVANCED_FACE ( 'NONE', ( #16605 ), #27439, .F. ) ;
#16744=VECTOR ( 'NONE', #1331, 1000.000000000000000 ) ;
#16746=VERTEX_POINT ( 'NONE', #13743 ) ;
#16760=VECTOR ( 'NONE', #23668, 1000.000000000000000 ) ;
#16761=EDGE_CURVE ( 'NONE', #23261, #5794, #21661, .T. ) ;
#16762=ORIENTED_EDGE ( 'NONE', *, *, #24709, .T. ) ;
#16763=ORIENTED_EDGE ( 'NONE', *, *, #12854, .T. ) ;
#16766=AXIS2_PLACEMENT_3D ( 'NONE', #34415, #6996, #25881 ) ;
#16770=VECTOR ( 'NONE', #12156, 1000.000000000000000 ) ;
#16771=ORIENTED_EDGE ( 'NONE', *, *, #29776, .T. ) ;
#16773=DIRECTION ( 'NONE',  ( 0.000000000000000000, 0.000000000000000000, 1.000000000000000000 ) ) ;
#16778=DIRECTION ( 'NONE',  ( 1.232595164407830946E-32, 7.496237820289040735E-63, -1.000000000000000000 ) ) ;
#16779=ORIENTED_EDGE ( 'NONE', *, *, #5639, .T. ) ;
#16784=CYLINDRICAL_SURFACE ( 'NONE', #17851, 3.999999999999948042 ) ;
#16790=EDGE_CURVE ( 'NONE', #34661, #890, #24576, .T. ) ;
#16793=CIRCLE ( 'NONE', #27561, 4.750000000000004441 ) ;
#16795=EDGE_CURVE ( 'NONE', #13175, #31799, #30646, .T. ) ;
#16796=AXIS2_PLACEMENT_3D ( 'NONE', #30902, #28236, #25552 ) ;
#16797=CARTESIAN_POINT ( 'NONE',  ( 15.99999999999998579, 4.559999999999908127, 172.9900000000000091 ) ) ;
#16799=DIRECTION ( 'NONE',  ( -1.000000000000000000, 0.000000000000000000, 0.000000000000000000 ) ) ;
#16800=VECTOR ( 'NONE', #30571, 1000.000000000000000 ) ;
#16801=AXIS2_PLACEMENT_3D ( 'NONE', #23651, #15305, #25969 ) ;
#16803=EDGE_LOOP ( 'NONE', ( #9995, #25248, #14320, #19490 ) ) ;
#16806=AXIS2_PLACEMENT_3D ( 'NONE', #15383, #23377, #28554 ) ;
#16807=ORIENTED_EDGE ( 'NONE', *, *, #22419, .F. ) ;
#16810=ADVANCED_FACE ( 'NONE', ( #19798 ), #16784, .F. ) ;
#16811=ADVANCED_FACE ( 'NONE', ( #11965 ), #27966, .F. ) ;
#16812=VECTOR ( 'NONE', #2257, 1000.000000000000000 ) ;
#16816=ORIENTED_EDGE ( 'NONE', *, *, #27429, .F. ) ;
#16817=EDGE_LOOP ( 'NONE', ( #21915, #7425, #22519, #21542, #6755, #14808, #1811, #1608, #25410, #29479, #1765, #9271, #20505, #6127, #32271, #22484 ) ) ;
#16822=ORIENTED_EDGE ( 'NONE', *, *, #22506, .T. ) ;
#16824=CARTESIAN_POINT ( 'NONE',  ( -499.9999999999999432, 140.9999999999999716, -187.0000000000000000 ) ) ;
#16826=ORIENTED_EDGE ( 'NONE', *, *, #17909, .F. ) ;
#16837=ORIENTED_EDGE ( 'NONE', *, *, #29387, .F. ) ;
#16841=CARTESIAN_POINT ( 'NONE',  ( -12.00000000000001066, -145.0000000000000000, 155.0000000000000000 ) ) ;
#16844=ORIENTED_EDGE ( 'NONE', *, *, #4115, .T. ) ;
#16847=CYLINDRICAL_SURFACE ( 'NONE', #10040, 7.999999999999952038 ) ;
#16849=FACE_OUTER_BOUND ( 'NONE', #6885, .T. ) ;
#16850=CARTESIAN_POINT ( 'NONE',  ( -12.00000000000001066, 134.9999999999998863, 162.9999999999999716 ) ) ;
#16852=EDGE_CURVE ( 'NONE', #12415, #13518, #6462, .T. ) ;
#16857=DIRECTION ( 'NONE',  ( -1.232595164407830946E-32, -3.421138828918010427E-49, 1.000000000000000000 ) ) ;
#16858=LINE ( 'NONE', #27682, #29572 ) ;
#16859=ORIENTED_EDGE ( 'NONE', *, *, #32824, .T. ) ;
#16860=EDGE_LOOP ( 'NONE', ( #5465, #10940, #21218, #774, #30282, #29527, #8500, #988 ) ) ;
#16871=AXIS2_PLACEMENT_3D ( 'NONE', #14556, #25203, #33398 ) ;
#16872=DIRECTION ( 'NONE',  ( 0.000000000000000000, 1.310824597558155437E-49, 1.000000000000000000 ) ) ;
#16875=CARTESIAN_POINT ( 'NONE',  ( -430.0000000000000000, -131.0000000000000000, 128.0000000000000000 ) ) ;
#16877=ORIENTED_EDGE ( 'NONE', *, *, #8308, .F. ) ;
#16879=DIRECTION ( 'NONE',  ( 0.000000000000000000, 0.000000000000000000, -1.000000000000000000 ) ) ;
#16880=DIRECTION ( 'NONE',  ( -1.000000000000000000, 0.000000000000000000, 0.000000000000000000 ) ) ;
#16882=EDGE_LOOP ( 'NONE', ( #29155, #12686, #12169, #18671 ) ) ;
#16885=CARTESIAN_POINT ( 'NONE',  ( -345.0000000000000000, 134.9999999999999716, 125.9999999999999716 ) ) ;
#16887=AXIS2_PLACEMENT_3D ( 'NONE', #23715, #24049, #7863 ) ;
#16888=ORIENTED_EDGE ( 'NONE', *, *, #27157, .F. ) ;
#16889=EDGE_CURVE ( 'NONE', #5434, #8847, #15575, .T. ) ;
#16891=DIRECTION ( 'NONE',  ( -1.232595164407830946E-32, -7.496237820289040735E-63, 1.000000000000000000 ) ) ;
#16892=CARTESIAN_POINT ( 'NONE',  ( -12.00000000000001066, 144.9999999999999147, 162.9999999999999716 ) ) ;
#16893=EDGE_CURVE ( 'NONE', #1848, #11811, #33125, .T. ) ;
#16897=DIRECTION ( 'NONE',  ( 2.891205793294675368E-16, 7.888609052210118054E-31, 1.000000000000000000 ) ) ;
#16899=ORIENTED_EDGE ( 'NONE', *, *, #29932, .T. ) ;
#16902=CARTESIAN_POINT ( 'NONE',  ( -500.0000000000000000, -113.0000000000000000, 194.9999999999999716 ) ) ;
#16904=EDGE_LOOP ( 'NONE', ( #26092, #24375, #11162, #34115, #34868, #10063, #6185, #30578 ) ) ;
#16905=ORIENTED_EDGE ( 'NONE', *, *, #9383, .F. ) ;
#16906=EDGE_LOOP ( 'NONE', ( #5492, #17815, #529, #30226 ) ) ;
#16909=MECHANICAL_DESIGN_GEOMETRIC_PRESENTATION_REPRESENTATION('',(#32229),#22585);
#16910=EDGE_CURVE ( 'NONE', #13666, #6940, #10836, .T. ) ;
#16912=VECTOR ( 'NONE', #9754, 1000.000000000000000 ) ;
#16913=AXIS2_PLACEMENT_3D ( 'NONE', #27038, #32542, #7984 ) ;
#16914=CARTESIAN_POINT ( 'NONE',  ( -499.9999999999999432, 112.9999999999999574, 194.9999999999999716 ) ) ;
#16915=ORIENTED_EDGE ( 'NONE', *, *, #7701, .T. ) ;
#16924=CIRCLE ( 'NONE', #13477, 3.999999999999976019 ) ;
#16927=CARTESIAN_POINT ( 'NONE',  ( -442.0000000000000000, 105.0000000000000142, -101.9999999999999858 ) ) ;
#16929=CARTESIAN_POINT ( 'NONE',  ( -430.0000000000000000, -135.0000000000000000, 126.0000000000000000 ) ) ;
#16933=LINE ( 'NONE', #27761, #15648 ) ;
#16937=AXIS2_PLACEMENT_3D ( 'NONE', #32421, #8216, #26561 ) ;
#16942=EDGE_CURVE ( 'NONE', #30178, #22409, #2810, .T. ) ;
#16943=ORIENTED_EDGE ( 'NONE', *, *, #19313, .T. ) ;
#16945=EDGE_CURVE ( 'NONE', #33601, #14361, #30052, .T. ) ;
#16946=VECTOR ( 'NONE', #7066, 1000.000000000000000 ) ;
#16952=ORIENTED_EDGE ( 'NONE', *, *, #16978, .T. ) ;
#16953=CARTESIAN_POINT ( 'NONE',  ( -442.0000000000000000, 105.0000000000000142, 194.9999999999999716 ) ) ;
#16955=LINE ( 'NONE', #11243, #1402 ) ;
#16957=VECTOR ( 'NONE', #11114, 1000.000000000000000 ) ;
#16959=EDGE_LOOP ( 'NONE', ( #11926, #5663, #5841, #1420, #1330, #26149, #11261, #1274 ) ) ;
#16960=LINE ( 'NONE', #19440, #6614 ) ;
#16961=DIRECTION ( 'NONE',  ( -0.000000000000000000, -0.000000000000000000, 1.000000000000000000 ) ) ;
#16965=ORIENTED_EDGE ( 'NONE', *, *, #7535, .T. ) ;
#16967=VECTOR ( 'NONE', #5888, 1000.000000000000000 ) ;
#16969=DIRECTION ( 'NONE',  ( -1.000000000000000000, 0.000000000000000000, -1.300283923313630633E-47 ) ) ;
#16973=DIRECTION ( 'NONE',  ( 0.000000000000000000, 2.309213040847544338E-50, 1.000000000000000000 ) ) ;
#16976=LINE ( 'NONE', #11622, #6495 ) ;
#16977=FACE_OUTER_BOUND ( 'NONE', #3024, .T. ) ;
#16978=EDGE_CURVE ( 'NONE', #22599, #33196, #24694, .T. ) ;
#16979=FACE_OUTER_BOUND ( 'NONE', #32046, .T. ) ;
#16980=ORIENTED_EDGE ( 'NONE', *, *, #30914, .F. ) ;
#16982=PLANE ( 'NONE',  #27946 ) ;
#16986=AXIS2_PLACEMENT_3D ( 'NONE', #29177, #4772, #6756 ) ;
#16990=ORIENTED_EDGE ( 'NONE', *, *, #6943, .F. ) ;
#16991=CARTESIAN_POINT ( 'NONE',  ( -20.00000000000007461, 136.9999999999999432, 159.0000000000000000 ) ) ;
#16994=DIRECTION ( 'NONE',  ( 0.000000000000000000, 1.000000000000000000, 1.224646799147353207E-16 ) ) ;
#16995=VECTOR ( 'NONE', #5700, 1000.000000000000000 ) ;
#16999=DIRECTION ( 'NONE',  ( 1.000000000000000000, 0.000000000000000000, 0.000000000000000000 ) ) ;
#17000=ORIENTED_EDGE ( 'NONE', *, *, #7655, .T. ) ;
#17002=FACE_BOUND ( 'NONE', #20680, .T. ) ;
#17003=CARTESIAN_POINT ( 'NONE',  ( -349.0000000000000000, 124.9999999999999432, 185.0000000000000000 ) ) ;
#17005=PLANE ( 'NONE',  #26 ) ;
#17008=ORIENTED_EDGE ( 'NONE', *, *, #2470, .F. ) ;
#17013=CARTESIAN_POINT ( 'NONE',  ( -361.0000000000000000, -125.0000000000000284, 166.9999999999999716 ) ) ;
#17021=EDGE_CURVE ( 'NONE', #10430, #18467, #9324, .T. ) ;
#17022=CARTESIAN_POINT ( 'NONE',  ( -499.9999999999999432, 112.9999999999999574, 155.0000000000000000 ) ) ;
#17024=LINE ( 'NONE', #14519, #16744 ) ;
#17026=DIRECTION ( 'NONE',  ( -1.000000000000000000, -3.469446951953834515E-18, 0.000000000000000000 ) ) ;
#17028=STYLED_ITEM('',(#35254),#12482);
#17033=EDGE_LOOP ( 'NONE', ( #34509, #25946, #16905, #2833 ) ) ;
#17034=CARTESIAN_POINT ( 'NONE',  ( -12.00000000000001066, 144.9999999999999716, -186.9999999999999716 ) ) ;
#17037=CARTESIAN_POINT ( 'NONE',  ( -365.0000000000000000, -125.0000000000000284, 113.9999999999999858 ) ) ;
#17040=DIRECTION ( 'NONE',  ( -3.040835319149746528E-31, -1.000000000000000000, 0.000000000000000000 ) ) ;
#17043=ORIENTED_EDGE ( 'NONE', *, *, #21303, .T. ) ;
#17049=AXIS2_PLACEMENT_3D ( 'NONE', #13974, #24807, #3965 ) ;
#17053=LINE ( 'NONE', #22195, #4829 ) ;
#17054=DIRECTION ( 'NONE',  ( 1.000000000000000000, -0.000000000000000000, -0.000000000000000000 ) ) ;
#17055=ADVANCED_FACE ( 'NONE', ( #13342 ), #35053, .T. ) ;
#17056=CARTESIAN_POINT ( 'NONE',  ( -414.0000000000000568, -104.9999999999999716, -187.0000000000000000 ) ) ;
#17065=CARTESIAN_POINT ( 'NONE',  ( -499.9999999999999432, 112.9999999999999574, 187.0000000000000000 ) ) ;
#17066=CYLINDRICAL_SURFACE ( 'NONE', #17950, 3.999999999999976019 ) ;
#17067=DIRECTION ( 'NONE',  ( -0.000000000000000000, 0.000000000000000000, -1.000000000000000000 ) ) ;
#17073=PLANE ( 'NONE',  #18406 ) ;
#17075=CARTESIAN_POINT ( 'NONE',  ( -499.9999999999999432, 136.9999999999999432, 187.0000000000000000 ) ) ;
#17081=CARTESIAN_POINT ( 'NONE',  ( -12.00000000000001243, 134.9999999999999432, -154.9999999999999716 ) ) ;
#17088=ORIENTED_EDGE ( 'NONE', *, *, #3252, .T. ) ;
#17090=LINE ( 'NONE', #27923, #25997 ) ;
#17095=DIRECTION ( 'NONE',  ( -1.232595164407831220E-32, 3.421138828918010427E-49, -1.000000000000000000 ) ) ;
#17096=ADVANCED_FACE ( 'NONE', ( #8683 ), #17073, .T. ) ;
#17098=EDGE_LOOP ( 'NONE', ( #29510, #22224, #12832, #34686 ) ) ;
#17100=DIRECTION ( 'NONE',  ( 0.000000000000000000, 0.000000000000000000, -1.000000000000000000 ) ) ;
#17106=DIRECTION ( 'NONE',  ( 0.000000000000000000, 1.000000000000000000, -1.310824597558155437E-49 ) ) ;
#17108=ORIENTED_EDGE ( 'NONE', *, *, #5755, .T. ) ;
#17109=ORIENTED_EDGE ( 'NONE', *, *, #26179, .F. ) ;
#17117=DIRECTION ( 'NONE',  ( 0.000000000000000000, 1.000000000000000000, 5.145227585319922065E-49 ) ) ;
#17120=DIRECTION ( 'NONE',  ( 5.546364386991661285E-52, 0.000000000000000000, 1.000000000000000000 ) ) ;
#17121=CARTESIAN_POINT ( 'NONE',  ( -414.0000000000000568, 137.0000000000000000, -155.0000000000000000 ) ) ;
#17123=CARTESIAN_POINT ( 'NONE',  ( -12.00000000000001066, 108.9999999999999858, -155.0000000000000000 ) ) ;
#17125=VECTOR ( 'NONE', #32592, 1000.000000000000000 ) ;
#17127=ORIENTED_EDGE ( 'NONE', *, *, #1938, .F. ) ;
#17129=VECTOR ( 'NONE', #7747, 1000.000000000000000 ) ;
#17131=EDGE_CURVE ( 'NONE', #12639, #30526, #24874, .T. ) ;
#17132=CARTESIAN_POINT ( 'NONE',  ( -449.9999999999999432, 105.0000000000000142, -175.0000000000000000 ) ) ;
#17133=CARTESIAN_POINT ( 'NONE',  ( -70.00000000000000000, 75.55999999999990280, 172.9900000000000091 ) ) ;
#17140=ADVANCED_FACE ( 'NONE', ( #1035, #14579 ), #6357, .T. ) ;
#17144=DIRECTION ( 'NONE',  ( -1.000000000000000000, 0.000000000000000000, -0.000000000000000000 ) ) ;
#17156=EDGE_LOOP ( 'NONE', ( #10956, #34209, #20511, #3750 ) ) ;
#17159=AXIS2_PLACEMENT_3D ( 'NONE', #24941, #10562, #21413 ) ;
#17160=VERTEX_POINT ( 'NONE', #33059 ) ;
#17161=VERTEX_POINT ( 'NONE', #11366 ) ;
#17162=FACE_OUTER_BOUND ( 'NONE', #15396, .T. ) ;
#17163=ORIENTED_EDGE ( 'NONE', *, *, #3240, .F. ) ;
#17164=VERTEX_POINT ( 'NONE', #27550 ) ;
#17165=LINE ( 'NONE', #28528, #6541 ) ;
#17166=AXIS2_PLACEMENT_3D ( 'NONE', #15721, #2171, #19393 ) ;
#17171=ORIENTED_EDGE ( 'NONE', *, *, #17332, .F. ) ;
#17175=CARTESIAN_POINT ( 'NONE',  ( 19.99999999999998224, -115.0000000000000000, -158.9999999999999716 ) ) ;
#17178=ORIENTED_EDGE ( 'NONE', *, *, #13965, .T. ) ;
#17179=AXIS2_PLACEMENT_3D ( 'NONE', #29563, #7476, #29390 ) ;
#17180=FACE_OUTER_BOUND ( 'NONE', #20263, .T. ) ;
#17184=CIRCLE ( 'NONE', #14336, 3.999999999999989786 ) ;
#17192=DIRECTION ( 'NONE',  ( -0.000000000000000000, -1.000000000000000000, -0.000000000000000000 ) ) ;
#17194=EDGE_CURVE ( 'NONE', #10950, #10851, #1349, .T. ) ;
#17196=EDGE_LOOP ( 'NONE', ( #1699, #23789, #19322, #4296 ) ) ;
#17197=PLANE ( 'NONE',  #9338 ) ;
#17198=CYLINDRICAL_SURFACE ( 'NONE', #27338, 2.000000000000001776 ) ;
#17199=CARTESIAN_POINT ( 'NONE',  ( -499.9999999999999432, -137.0000000000000000, -162.9999999999999716 ) ) ;
#17200=ORIENTED_EDGE ( 'NONE', *, *, #24178, .T. ) ;
#17204=CARTESIAN_POINT ( 'NONE',  ( -347.0000000000000000, -135.0000000000000000, 126.0000000000000000 ) ) ;
#17205=ORIENTED_EDGE ( 'NONE', *, *, #17194, .T. ) ;
#17207=ADVANCED_FACE ( 'NONE', ( #510 ), #338, .T. ) ;
#17208=VECTOR ( 'NONE', #24868, 1000.000000000000000 ) ;
#17213=ORIENTED_EDGE ( 'NONE', *, *, #3165, .T. ) ;
#17215=DIRECTION ( 'NONE',  ( -1.300283923313630633E-47, 0.000000000000000000, -1.000000000000000000 ) ) ;
#17222=EDGE_LOOP ( 'NONE', ( #2418, #14054, #16733, #9951 ) ) ;
#17225=CARTESIAN_POINT ( 'NONE',  ( -365.0000000000000000, -119.0000000000000000, 113.9999999999999858 ) ) ;
#17226=EDGE_CURVE ( 'NONE', #23064, #17161, #25779, .T. ) ;
#17227=DIRECTION ( 'NONE',  ( 0.000000000000000000, 0.000000000000000000, -1.000000000000000000 ) ) ;
#17228=CYLINDRICAL_SURFACE ( 'NONE', #13139, 7.999999999999979572 ) ;
#17230=CARTESIAN_POINT ( 'NONE',  ( -499.9999999999999432, 108.9999999999999858, -187.0000000000000000 ) ) ;
#17231=ORIENTED_EDGE ( 'NONE', *, *, #32856, .T. ) ;
#17232=CARTESIAN_POINT ( 'NONE',  ( -12.00000000000001066, -60.99999999999997158, -175.0000000000000000 ) ) ;
#17239=ADVANCED_FACE ( 'NONE', ( #6711 ), #1558, .F. ) ;
#17241=CARTESIAN_POINT ( 'NONE',  ( -449.9999999999999432, 104.9999999999999858, -162.9999999999999716 ) ) ;
#17242=VERTEX_POINT ( 'NONE', #15097 ) ;
#17244=EDGE_LOOP ( 'NONE', ( #31236, #3442, #24962, #31614 ) ) ;
#17245=PLANE ( 'NONE',  #6346 ) ;
#17246=CARTESIAN_POINT ( 'NONE',  ( -500.0000000000000000, -113.0000000000000000, -155.0000000000000000 ) ) ;
#17251=ORIENTED_EDGE ( 'NONE', *, *, #6404, .F. ) ;
#17252=CARTESIAN_POINT ( 'NONE',  ( -500.0000000000000000, 136.9999999999999432, -155.0000000000000000 ) ) ;
#17253=EDGE_CURVE ( 'NONE', #33693, #2489, #16172, .T. ) ;
#17255=CARTESIAN_POINT ( 'NONE',  ( -12.00000000000001066, -112.9999999999999858, -155.0000000000000284 ) ) ;
#17257=VECTOR ( 'NONE', #9717, 1000.000000000000000 ) ;
#17261=VERTEX_POINT ( 'NONE', #4029 ) ;
#17263=VECTOR ( 'NONE', #28380, 1000.000000000000000 ) ;
#17267=CARTESIAN_POINT ( 'NONE',  ( -500.0000000000000000, -137.0000000000000000, 162.9999999999999716 ) ) ;
#17269=ORIENTED_EDGE ( 'NONE', *, *, #6856, .T. ) ;
#17272=ORIENTED_EDGE ( 'NONE', *, *, #32043, .T. ) ;
#17273=EDGE_CURVE ( 'NONE', #33070, #35069, #23279, .T. ) ;
#17275=LINE ( 'NONE', #11925, #4054 ) ;
#17279=CARTESIAN_POINT ( 'NONE',  ( 11.99999999999999645, 108.9999999999999858, 155.0000000000000000 ) ) ;
#17282=CARTESIAN_POINT ( 'NONE',  ( 11.99999999999999645, -145.0000000000000000, -162.9999999999999432 ) ) ;
#17283=LINE ( 'NONE', #3372, #28619 ) ;
#17288=DIRECTION ( 'NONE',  ( -3.469446951953832974E-18, -1.000000000000000000, -7.888609052210116302E-31 ) ) ;
#17289=ADVANCED_FACE ( 'NONE', ( #9915 ), #25577, .T. ) ;
#17290=DIRECTION ( 'NONE',  ( -0.000000000000000000, 0.000000000000000000, 1.000000000000000000 ) ) ;
#17291=VERTEX_POINT ( 'NONE', #25759 ) ;
#17294=ORIENTED_EDGE ( 'NONE', *, *, #19414, .T. ) ;
#17299=EDGE_CURVE ( 'NONE', #726, #8847, #12598, .T. ) ;
#17302=ORIENTED_EDGE ( 'NONE', *, *, #31968, .F. ) ;
#17303=CARTESIAN_POINT ( 'NONE',  ( -442.0000000000000000, 141.0000000000000000, -175.0000000000000000 ) ) ;
#17307=DIRECTION ( 'NONE',  ( -0.000000000000000000, 1.000000000000000000, -0.000000000000000000 ) ) ;
#17309=VECTOR ( 'NONE', #3063, 1000.000000000000000 ) ;
#17312=AXIS2_PLACEMENT_3D ( 'NONE', #35042, #2628, #2798 ) ;
#17313=CARTESIAN_POINT ( 'NONE',  ( -410.0000000000000568, 113.0000000000000000, -155.0000000000000000 ) ) ;
#17314=CYLINDRICAL_SURFACE ( 'NONE', #32363, 3.999999999999948042 ) ;
#17315=CARTESIAN_POINT ( 'NONE',  ( -418.0000000000000000, 104.9999999999999858, -175.0000000000000000 ) ) ;
#17316=CARTESIAN_POINT ( 'NONE',  ( -418.0000000000000000, -124.9999999999999858, -77.99999999999997158 ) ) ;
#17317=ORIENTED_EDGE ( 'NONE', *, *, #10577, .F. ) ;
#17320=ORIENTED_EDGE ( 'NONE', *, *, #10037, .F. ) ;
#17322=CARTESIAN_POINT ( 'NONE',  ( -347.0000000000000000, -125.0000000000000284, 168.9999999999999716 ) ) ;
#17324=CARTESIAN_POINT ( 'NONE',  ( -12.00000000000001066, -124.9999999999999432, -154.9999999999999716 ) ) ;
#17325=CARTESIAN_POINT ( 'NONE',  ( 11.99999999999999645, 134.9999999999999432, -194.9999999999999432 ) ) ;
#17327=DIRECTION ( 'NONE',  ( 2.891205793294675368E-16, 0.000000000000000000, -1.000000000000000000 ) ) ;
#17331=VECTOR ( 'NONE', #15769, 1000.000000000000000 ) ;
#17332=EDGE_CURVE ( 'NONE', #11445, #1780, #13778, .T. ) ;
#17334=ORIENTED_EDGE ( 'NONE', *, *, #17689, .T. ) ;
#17340=EDGE_CURVE ( 'NONE', #23628, #35, #28611, .T. ) ;
#17342=ORIENTED_EDGE ( 'NONE', *, *, #9790, .T. ) ;
#17343=CARTESIAN_POINT ( 'NONE',  ( -442.0000000000000000, -109.0000000000000142, -155.0000000000000000 ) ) ;
#17347=CARTESIAN_POINT ( 'NONE',  ( 11.99999999999999645, 144.9999999999999716, 155.0000000000000000 ) ) ;
#17348=CIRCLE ( 'NONE', #13348, 3.999999999999948042 ) ;
#17349=ORIENTED_EDGE ( 'NONE', *, *, #17797, .F. ) ;
#17350=DIRECTION ( 'NONE',  ( -3.469446951953832974E-18, -1.000000000000000000, -7.888609052210116302E-31 ) ) ;
#17351=LINE ( 'NONE', #33343, #18309 ) ;
#17356=AXIS2_PLACEMENT_3D ( 'NONE', #19226, #24886, #5659 ) ;
#17358=DIRECTION ( 'NONE',  ( 0.000000000000000000, 0.000000000000000000, -1.000000000000000000 ) ) ;
#17359=LINE ( 'NONE', #10811, #1728 ) ;
#17362=VERTEX_POINT ( 'NONE', #18596 ) ;
#17363=PLANE ( 'NONE',  #5423 ) ;
#17364=AXIS2_PLACEMENT_3D ( 'NONE', #27536, #31853, #18364 ) ;
#17365=CIRCLE ( 'NONE', #10535, 4.750000000000004441 ) ;
#17366=PLANE ( 'NONE',  #32917 ) ;
#17367=ORIENTED_EDGE ( 'NONE', *, *, #32344, .F. ) ;
#17369=AXIS2_PLACEMENT_3D ( 'NONE', #6882, #9407, #4214 ) ;
#17370=FACE_OUTER_BOUND ( 'NONE', #24683, .T. ) ;
#17371=CARTESIAN_POINT ( 'NONE',  ( -414.0000000000000568, -112.9999999999999858, -155.0000000000000000 ) ) ;
#17374=CARTESIAN_POINT ( 'NONE',  ( -12.00000000000001066, -64.99999999999997158, -154.9999999999999716 ) ) ;
#17376=VERTEX_POINT ( 'NONE', #14926 ) ;
#17377=CARTESIAN_POINT ( 'NONE',  ( -19.99999999999998934, 112.9999999999999574, -155.0000000000000000 ) ) ;
#17378=CARTESIAN_POINT ( 'NONE',  ( -12.00000000000003908, -134.9999999999999716, -194.9999999999999432 ) ) ;
#17380=AXIS2_PLACEMENT_3D ( 'NONE', #14839, #28696, #9490 ) ;
#17382=DIRECTION ( 'NONE',  ( 0.000000000000000000, 6.123233995736766036E-17, 1.000000000000000000 ) ) ;
#17384=ORIENTED_EDGE ( 'NONE', *, *, #5480, .T. ) ;
#17386=EDGE_CURVE ( 'NONE', #31534, #16134, #18938, .T. ) ;
#17387=AXIS2_PLACEMENT_3D ( 'NONE', #17246, #8674, #11718 ) ;
#17388=VECTOR ( 'NONE', #6488, 1000.000000000000000 ) ;
#17389=ORIENTED_EDGE ( 'NONE', *, *, #19936, .F. ) ;
#17392=ORIENTED_EDGE ( 'NONE', *, *, #10487, .T. ) ;
#17393=ADVANCED_FACE ( 'NONE', ( #23108 ), #16329, .T. ) ;
#17394=CARTESIAN_POINT ( 'NONE',  ( -499.9999999999999432, -113.0000000000000000, -155.0000000000000000 ) ) ;
#17395=CLOSED_SHELL ( 'NONE', ( #15927, #34029, #21377, #32004, #25151, #29491, #20971, #30392, #5562, #6657, #24997, #8307, #20820, #27883, #15678, #30473, #21980, #14151, #8269, #656, #32649, #28967, #28307, #21969, #32578, #14025, #14975, #23242, #28890, #13860, #35013, #23309, #20730, #30979, #15290, #10079, #32519, #4839, #2808, #19593, #8630, #26565, #2591, #21644, #19943, #31121, #19581, #8249, #1201, #5685, #34578, #25801, #12587, #15274, #14734, #24200, #15118, #30173, #23378, #26341, #24764, #7403, #28335, #20880, #3768, #17055, #32825, #33248, #30366, #24599, #26625, #25383, #12841, #16161, #3801, #10231, #19950, #27827, #6411, #39, #34555, #12541, #18541, #5249, #25235, #28918, #3118, #34155, #34286, #16497, #15212, #165, #17207, #29880, #31526, #28856, #13667, #32348, #5652, #27388, #17466, #25089 ) ) ;
#17396=ADVANCED_FACE ( 'NONE', ( #5256 ), #26458, .T. ) ;
#17399=DIRECTION ( 'NONE',  ( 1.000000000000000000, -3.540705920434608777E-32, 2.891205793294675368E-16 ) ) ;
#17400=EDGE_CURVE ( 'NONE', #14255, #24525, #15625, .T. ) ;
#17403=VERTEX_POINT ( 'NONE', #13640 ) ;
#17405=DIRECTION ( 'NONE',  ( 1.000000000000000000, 0.000000000000000000, -1.232595164407831220E-32 ) ) ;
#17407=DIRECTION ( 'NONE',  ( 1.000000000000000000, -0.000000000000000000, -0.000000000000000000 ) ) ;
#17409=VECTOR ( 'NONE', #9787, 1000.000000000000000 ) ;
#17410=DIRECTION ( 'NONE',  ( 1.000000000000000000, 0.000000000000000000, 0.000000000000000000 ) ) ;
#17415=PLANE ( 'NONE',  #1802 ) ;
#17416=EDGE_CURVE ( 'NONE', #33601, #19123, #29792, .T. ) ;
#17420=FACE_OUTER_BOUND ( 'NONE', #5923, .T. ) ;
#17421=EDGE_LOOP ( 'NONE', ( #973, #19497, #11942, #15188 ) ) ;
#17422=CARTESIAN_POINT ( 'NONE',  ( -500.0000000000000000, -137.0000000000000000, 155.0000000000000000 ) ) ;
#17427=VERTEX_POINT ( 'NONE', #29490 ) ;
#17439=DIRECTION ( 'NONE',  ( 0.000000000000000000, -1.224646799147353207E-16, 1.000000000000000000 ) ) ;
#17440=CARTESIAN_POINT ( 'NONE',  ( -499.9999999999999432, 112.9999999999999574, 162.9999999999999716 ) ) ;
#17441=EDGE_CURVE ( 'NONE', #34959, #26754, #7042, .T. ) ;
#17444=EDGE_LOOP ( 'NONE', ( #15419, #518, #7966, #21082, #15024, #28910, #28496, #9315, #3735, #20905, #3819, #20402, #18353, #30920, #24445, #27932 ) ) ;
#17445=ORIENTED_EDGE ( 'NONE', *, *, #29088, .T. ) ;
#17449=LINE ( 'NONE', #3874, #30974 ) ;
#17451=EDGE_LOOP ( 'NONE', ( #10048, #29165, #16289, #11038 ) ) ;
#17453=DIRECTION ( 'NONE',  ( 0.000000000000000000, 1.000000000000000000, 5.145227585319922065E-49 ) ) ;
#17461=CARTESIAN_POINT ( 'NONE',  ( -19.99999999999998934, 136.9999999999999716, -175.0000000000000284 ) ) ;
#17463=CIRCLE ( 'NONE', #33331, 7.999999999999979572 ) ;
#17466=ADVANCED_FACE ( 'NONE', ( #13121 ), #2079, .F. ) ;
#17467=CARTESIAN_POINT ( 'NONE',  ( -442.0000000000000000, 104.9999999999999858, -162.9999999999999716 ) ) ;
#17468=EDGE_CURVE ( 'NONE', #8951, #32109, #2597, .T. ) ;
#17475=ORIENTED_EDGE ( 'NONE', *, *, #24145, .T. ) ;
#17481=VECTOR ( 'NONE', #12840, 1000.000000000000000 ) ;
#17482=DIRECTION ( 'NONE',  ( -0.000000000000000000, 1.000000000000000000, -0.000000000000000000 ) ) ;
#17483=VECTOR ( 'NONE', #16390, 1000.000000000000000 ) ;
#17485=ORIENTED_EDGE ( 'NONE', *, *, #33581, .T. ) ;
#17486=CARTESIAN_POINT ( 'NONE',  ( -430.0000000000000000, -131.0000000000000000, 113.9999999999999858 ) ) ;
#17488=DIRECTION ( 'NONE',  ( 1.000000000000000000, 0.000000000000000000, 0.000000000000000000 ) ) ;
#17490=EDGE_LOOP ( 'NONE', ( #33824, #27165, #31441, #2246 ) ) ;
#17491=VERTEX_POINT ( 'NONE', #8471 ) ;
#17498=CARTESIAN_POINT ( 'NONE',  ( -355.0000000000000000, 130.9999999999999716, 113.9999999999999858 ) ) ;
#17502=FACE_BOUND ( 'NONE', #30186, .T. ) ;
#17504=ADVANCED_FACE ( 'NONE', ( #6310, #19339 ), #30716, .T. ) ;
#17505=DIRECTION ( 'NONE',  ( 1.000000000000000000, 0.000000000000000000, 5.546364386991661285E-52 ) ) ;
#17512=ORIENTED_EDGE ( 'NONE', *, *, #31300, .T. ) ;
#17517=ORIENTED_EDGE ( 'NONE', *, *, #4972, .F. ) ;
#17520=DIRECTION ( 'NONE',  ( 0.000000000000000000, 0.000000000000000000, -1.000000000000000000 ) ) ;
#17521=ORIENTED_EDGE ( 'NONE', *, *, #24615, .F. ) ;
#17528=LINE ( 'NONE', #20004, #15834 ) ;
#17529=FACE_BOUND ( 'NONE', #23802, .T. ) ;
#17534=DIRECTION ( 'NONE',  ( -1.000000000000000000, 0.000000000000000000, 0.000000000000000000 ) ) ;
#17535=CARTESIAN_POINT ( 'NONE',  ( 11.99999999999999645, 124.9999999999999716, 155.0000000000000000 ) ) ;
#17537=VERTEX_POINT ( 'NONE', #32843 ) ;
#17538=CARTESIAN_POINT ( 'NONE',  ( -20.00000000000007461, 104.9999999999999858, 162.9999999999999716 ) ) ;
#17539=DIRECTION ( 'NONE',  ( 0.000000000000000000, 0.000000000000000000, -1.000000000000000000 ) ) ;
#17542=DIRECTION ( 'NONE',  ( 1.300283923313630633E-47, 0.000000000000000000, 1.000000000000000000 ) ) ;
#17544=EDGE_CURVE ( 'NONE', #10934, #16746, #19172, .T. ) ;
#17545=DIRECTION ( 'NONE',  ( 0.000000000000000000, -1.000000000000000000, 6.123233995736766036E-17 ) ) ;
#17546=CARTESIAN_POINT ( 'NONE',  ( -442.0000000000000000, -125.0000000000000000, 159.0000000000000000 ) ) ;
#17551=CARTESIAN_POINT ( 'NONE',  ( -15.99999999999998579, -145.0000000000000000, -162.9999999999999432 ) ) ;
#17555=CARTESIAN_POINT ( 'NONE',  ( -449.9999999999999432, -125.0000000000000000, 162.9999999999999716 ) ) ;
#17562=ORIENTED_EDGE ( 'NONE', *, *, #17468, .F. ) ;
#17564=ORIENTED_EDGE ( 'NONE', *, *, #18230, .F. ) ;
#17565=EDGE_LOOP ( 'NONE', ( #20929, #24541, #17334, #3653 ) ) ;
#17570=DIRECTION ( 'NONE',  ( -0.000000000000000000, 1.000000000000000000, -0.000000000000000000 ) ) ;
#17576=DIRECTION ( 'NONE',  ( 0.000000000000000000, 0.000000000000000000, 1.000000000000000000 ) ) ;
#17577=CARTESIAN_POINT ( 'NONE',  ( -19.99999999999998934, 124.9999999999999716, 187.0000000000000000 ) ) ;
#17579=DIRECTION ( 'NONE',  ( 0.000000000000000000, 1.131431318426415506E-52, 1.000000000000000000 ) ) ;
#17580=LINE ( 'NONE', #28416, #22704 ) ;
#17581=ORIENTED_EDGE ( 'NONE', *, *, #3208, .F. ) ;
#17582=CARTESIAN_POINT ( 'NONE',  ( -12.00000000000001066, -112.9999999999999858, 174.9999999999999432 ) ) ;
#17583=DIRECTION ( 'NONE',  ( 0.000000000000000000, 0.000000000000000000, -1.000000000000000000 ) ) ;
#17584=EDGE_CURVE ( 'NONE', #11839, #34323, #26944, .T. ) ;
#17586=FACE_OUTER_BOUND ( 'NONE', #18729, .T. ) ;
#17587=VERTEX_POINT ( 'NONE', #470 ) ;
#17588=LINE ( 'NONE', #11889, #34279 ) ;
#17589=ORIENTED_EDGE ( 'NONE', *, *, #16790, .T. ) ;
#17590=EDGE_CURVE ( 'NONE', #33889, #26771, #13896, .T. ) ;
#17591=LINE ( 'NONE', #24862, #20195 ) ;
#17594=VECTOR ( 'NONE', #12743, 1000.000000000000000 ) ;
#17597=EDGE_CURVE ( 'NONE', #10465, #10319, #21817, .T. ) ;
#17598=DIRECTION ( 'NONE',  ( 0.000000000000000000, 1.000000000000000000, 5.053935297177146739E-49 ) ) ;
#17602=ORIENTED_EDGE ( 'NONE', *, *, #15479, .F. ) ;
#17608=CIRCLE ( 'NONE', #18742, 4.000000000000003553 ) ;
#17610=DIRECTION ( 'NONE',  ( -1.000000000000000000, 0.000000000000000000, 0.000000000000000000 ) ) ;
#17613=ORIENTED_EDGE ( 'NONE', *, *, #27808, .F. ) ;
#17614=ORIENTED_EDGE ( 'NONE', *, *, #11059, .F. ) ;
#17617=CARTESIAN_POINT ( 'NONE',  ( 11.99999999999999645, -124.9999999999999432, -154.9999999999999716 ) ) ;
#17620=FACE_OUTER_BOUND ( 'NONE', #23146, .T. ) ;
#17622=LINE ( 'NONE', #1576, #25392 ) ;
#17624=VERTEX_POINT ( 'NONE', #8294 ) ;
#17632=EDGE_CURVE ( 'NONE', #12833, #29646, #22967, .T. ) ;
#17635=EDGE_CURVE ( 'NONE', #30234, #23829, #30012, .T. ) ;
#17641=ORIENTED_EDGE ( 'NONE', *, *, #27386, .T. ) ;
#17645=CARTESIAN_POINT ( 'NONE',  ( -499.9999999999999432, 112.9999999999999574, -162.9999999999999716 ) ) ;
#17646=CARTESIAN_POINT ( 'NONE',  ( -442.0000000000000000, -124.9999999999999858, -73.99999999999998579 ) ) ;
#17648=ORIENTED_EDGE ( 'NONE', *, *, #31303, .T. ) ;
#17650=CARTESIAN_POINT ( 'NONE',  ( -449.9999999999999432, 137.0000000000000000, -155.0000000000000000 ) ) ;
#17655=DIRECTION ( 'NONE',  ( 1.000000000000000000, 0.000000000000000000, 5.546364386991661285E-52 ) ) ;
#17656=CARTESIAN_POINT ( 'NONE',  ( -499.9999999999999432, 136.9999999999999432, 190.9999999999999716 ) ) ;
#17660=EDGE_CURVE ( 'NONE', #25758, #14377, #19570, .T. ) ;
#17664=LINE ( 'NONE', #15333, #406 ) ;
#17668=DIRECTION ( 'NONE',  ( -1.232595164407831220E-32, 3.421138828918010427E-49, -1.000000000000000000 ) ) ;
#17671=CARTESIAN_POINT ( 'NONE',  ( -418.0000000000000000, -125.0000000000000000, 190.9999999999999716 ) ) ;
#17672=ADVANCED_FACE ( 'NONE', ( #33552 ), #1167, .F. ) ;
#17678=DIRECTION ( 'NONE',  ( 1.000000000000000000, 0.000000000000000000, 0.000000000000000000 ) ) ;
#17680=VERTEX_POINT ( 'NONE', #1516 ) ;
#17686=ORIENTED_EDGE ( 'NONE', *, *, #9526, .T. ) ;
#17688=DIRECTION ( 'NONE',  ( 1.000000000000000000, 3.040835319149746090E-31, 1.232595164407830946E-32 ) ) ;
#17689=EDGE_CURVE ( 'NONE', #9096, #30302, #30888, .T. ) ;
#17690=ADVANCED_FACE ( 'NONE', ( #7015 ), #12039, .F. ) ;
#17691=VERTEX_POINT ( 'NONE', #9355 ) ;
#17692=DIRECTION ( 'NONE',  ( -0.000000000000000000, 1.000000000000000000, -0.000000000000000000 ) ) ;
#17693=CARTESIAN_POINT ( 'NONE',  ( 11.99999999999999645, 136.9999999999999716, 155.0000000000000000 ) ) ;
#17694=ORIENTED_EDGE ( 'NONE', *, *, #1691, .F. ) ;
#17697=CIRCLE ( 'NONE', #14849, 3.999999999999976019 ) ;
#17699=CARTESIAN_POINT ( 'NONE',  ( -12.00000000000001066, -24.99999999999999289, 154.9999999999999716 ) ) ;
#17700=DIRECTION ( 'NONE',  ( -0.000000000000000000, -1.000000000000000000, -0.000000000000000000 ) ) ;
#17706=DIRECTION ( 'NONE',  ( -5.546364386991661285E-52, 0.000000000000000000, -1.000000000000000000 ) ) ;
#17707=ORIENTED_EDGE ( 'NONE', *, *, #13190, .F. ) ;
#17710=DIRECTION ( 'NONE',  ( 0.000000000000000000, 1.000000000000000000, 1.224646799147353207E-16 ) ) ;
#17711=CARTESIAN_POINT ( 'NONE',  ( -442.0000000000000000, 104.9999999999999858, -187.0000000000000000 ) ) ;
#17715=LINE ( 'NONE', #17022, #11006 ) ;
#17717=CARTESIAN_POINT ( 'NONE',  ( -442.0000000000000000, 137.0000000000000000, 154.9999999999999716 ) ) ;
#17718=DIRECTION ( 'NONE',  ( -1.000000000000000000, 0.000000000000000000, 0.000000000000000000 ) ) ;
#17719=CARTESIAN_POINT ( 'NONE',  ( -70.00000000000000000, 75.55999999999990280, -177.7400000000000091 ) ) ;
#17720=ORIENTED_EDGE ( 'NONE', *, *, #34504, .T. ) ;
#17721=CARTESIAN_POINT ( 'NONE',  ( 19.99999999999998224, -115.0000000000000000, -158.9999999999999716 ) ) ;
#17728=ORIENTED_EDGE ( 'NONE', *, *, #14727, .T. ) ;
#17730=CARTESIAN_POINT ( 'NONE',  ( -414.0000000000000568, -124.9999999999999716, 132.0000000000000000 ) ) ;
#17732=EDGE_CURVE ( 'NONE', #10757, #23038, #1970, .T. ) ;
#17734=EDGE_CURVE ( 'NONE', #31513, #31845, #6671, .T. ) ;
#17735=EDGE_CURVE ( 'NONE', #9803, #24429, #4508, .T. ) ;
#17736=CARTESIAN_POINT ( 'NONE',  ( -418.0000000000000000, 105.0000000000000142, 187.0000000000000000 ) ) ;
#17740=AXIS2_PLACEMENT_3D ( 'NONE', #140, #10998, #32706 ) ;
#17742=CARTESIAN_POINT ( 'NONE',  ( 11.99999999999999645, -115.0000000000000000, 162.9999999999999716 ) ) ;
#17744=CIRCLE ( 'NONE', #22269, 3.999999999999976019 ) ;
#17747=DIRECTION ( 'NONE',  ( -0.000000000000000000, 1.000000000000000000, -0.000000000000000000 ) ) ;
#17748=CARTESIAN_POINT ( 'NONE',  ( -20.00000000000004619, 136.9999999999999432, -194.9999999999999432 ) ) ;
#17750=EDGE_LOOP ( 'NONE', ( #2984, #6653, #14456, #23705 ) ) ;
#17751=CARTESIAN_POINT ( 'NONE',  ( -442.0000000000000000, -104.9999999999999858, -159.0000000000000000 ) ) ;
#17755=ORIENTED_EDGE ( 'NONE', *, *, #15255, .T. ) ;
#17756=LINE ( 'NONE', #34101, #17257 ) ;
#17760=CIRCLE ( 'NONE', #10339, 7.999999999999952038 ) ;
#17761=EDGE_LOOP ( 'NONE', ( #25233, #899, #14770, #20926 ) ) ;
#17762=AXIS2_PLACEMENT_3D ( 'NONE', #7424, #18320, #9465 ) ;
#17763=CYLINDRICAL_SURFACE ( 'NONE', #16591, 7.999999999999979572 ) ;
#17765=AXIS2_PLACEMENT_3D ( 'NONE', #8849, #25211, #33407 ) ;
#17766=ORIENTED_EDGE ( 'NONE', *, *, #2134, .T. ) ;
#17771=DIRECTION ( 'NONE',  ( -1.000000000000000000, -3.040835319149746528E-31, -1.232595164407830946E-32 ) ) ;
#17772=EDGE_CURVE ( 'NONE', #11839, #32731, #3988, .T. ) ;
#17773=CYLINDRICAL_SURFACE ( 'NONE', #19825, 3.999999999999976019 ) ;
#17778=ORIENTED_EDGE ( 'NONE', *, *, #9911, .F. ) ;
#17781=CLOSED_SHELL ( 'NONE', ( #24297, #22782, #16560, #24480, #18931, #10238, #16205, #13314, #12026, #13384, #30055, #24549, #15551, #32530, #31766, #14964, #1733, #25128 ) ) ;
#17782=EDGE_CURVE ( 'NONE', #31630, #14082, #23567, .T. ) ;
#17786=CARTESIAN_POINT ( 'NONE',  ( -418.0000000000000000, 105.0000000000000000, 139.9999999999999716 ) ) ;
#17787=DIRECTION ( 'NONE',  ( 0.000000000000000000, 0.000000000000000000, -1.000000000000000000 ) ) ;
#17797=EDGE_CURVE ( 'NONE', #14255, #10121, #21862, .T. ) ;
#17800=EDGE_LOOP ( 'NONE', ( #10212, #22876, #12959, #21682, #2131, #18702, #16719, #30620 ) ) ;
#17801=CARTESIAN_POINT ( 'NONE',  ( -500.0000000000000000, -137.0000000000000000, 194.9999999999999716 ) ) ;
#17802=CARTESIAN_POINT ( 'NONE',  ( 12.00000000000001066, -24.99999999999999289, -154.9999999999999716 ) ) ;
#17806=DIRECTION ( 'NONE',  ( -3.040835319149746090E-31, -1.000000000000000000, 0.000000000000000000 ) ) ;
#17807=CARTESIAN_POINT ( 'NONE',  ( -410.0000000000000568, 113.0000000000000000, -175.0000000000000000 ) ) ;
#17808=ORIENTED_EDGE ( 'NONE', *, *, #32870, .T. ) ;
#17810=ORIENTED_EDGE ( 'NONE', *, *, #8899, .T. ) ;
#17812=( GEOMETRIC_REPRESENTATION_CONTEXT ( 3 ) GLOBAL_UNCERTAINTY_ASSIGNED_CONTEXT ( ( #20292 ) ) GLOBAL_UNIT_ASSIGNED_CONTEXT ( ( #22824, #12678, #6957 ) ) REPRESENTATION_CONTEXT ( 'NONE', 'WORKASPACE' ) );
#17814=VECTOR ( 'NONE', #21754, 1000.000000000000000 ) ;
#17815=ORIENTED_EDGE ( 'NONE', *, *, #18334, .T. ) ;
#17820=FACE_OUTER_BOUND ( 'NONE', #22930, .T. ) ;
#17821=FACE_OUTER_BOUND ( 'NONE', #18546, .T. ) ;
#17822=EDGE_CURVE ( 'NONE', #22648, #7666, #21289, .T. ) ;
#17825=DIRECTION ( 'NONE',  ( 0.000000000000000000, 0.000000000000000000, -1.000000000000000000 ) ) ;
#17828=EDGE_CURVE ( 'NONE', #19084, #31987, #34786, .T. ) ;
#17829=ADVANCED_FACE ( 'NONE', ( #24084 ), #24711, .F. ) ;
#17830=CARTESIAN_POINT ( 'NONE',  ( -19.99999999999998934, -32.99999999999997158, -175.0000000000000000 ) ) ;
#17837=VECTOR ( 'NONE', #26878, 1000.000000000000000 ) ;
#17838=ORIENTED_EDGE ( 'NONE', *, *, #27854, .T. ) ;
#17840=DIRECTION ( 'NONE',  ( 1.000000000000000000, 0.000000000000000000, 0.000000000000000000 ) ) ;
#17841=ADVANCED_FACE ( 'NONE', ( #2210, #26766 ), #31917, .T. ) ;
#17842=CYLINDRICAL_SURFACE ( 'NONE', #14987, 3.999999999999976019 ) ;
#17844=DIRECTION ( 'NONE',  ( 0.000000000000000000, 3.374343856708137958E-53, -1.000000000000000000 ) ) ;
#17848=FACE_OUTER_BOUND ( 'NONE', #33435, .T. ) ;
#17851=AXIS2_PLACEMENT_3D ( 'NONE', #25466, #1094, #14101 ) ;
#17858=AXIS2_PLACEMENT_3D ( 'NONE', #4892, #13284, #10609 ) ;
#17862=ORIENTED_EDGE ( 'NONE', *, *, #11305, .F. ) ;
#17864=LINE ( 'NONE', #22672, #28148 ) ;
#17865=VERTEX_POINT ( 'NONE', #4863 ) ;
#17869=EDGE_LOOP ( 'NONE', ( #26045, #31975, #19829, #6091, #2497, #20814, #8997, #14741 ) ) ;
#17871=EDGE_CURVE ( 'NONE', #11374, #26985, #26943, .T. ) ;
#17874=CARTESIAN_POINT ( 'NONE',  ( -20.00000000000007461, 136.9999999999999432, 190.9999999999999716 ) ) ;
#17878=LINE ( 'NONE', #28710, #10300 ) ;
#17879=ORIENTED_EDGE ( 'NONE', *, *, #18340, .T. ) ;
#17882=AXIS2_PLACEMENT_3D ( 'NONE', #1725, #18133, #31448 ) ;
#17885=ORIENTED_EDGE ( 'NONE', *, *, #20299, .F. ) ;
#17888=DIRECTION ( 'NONE',  ( 0.000000000000000000, 0.000000000000000000, 1.000000000000000000 ) ) ;
#17889=DIRECTION ( 'NONE',  ( 0.000000000000000000, -1.000000000000000000, 0.000000000000000000 ) ) ;
#17891=CARTESIAN_POINT ( 'NONE',  ( -418.0000000000000000, 105.0000000000000142, -175.0000000000000000 ) ) ;
#17892=FACE_OUTER_BOUND ( 'NONE', #21310, .T. ) ;
#17893=CYLINDRICAL_SURFACE ( 'NONE', #27594, 7.999999999999979572 ) ;
#17894=VECTOR ( 'NONE', #9645, 1000.000000000000000 ) ;
#17895=CARTESIAN_POINT ( 'NONE',  ( -20.00000000000001776, -113.0000000000000000, 159.0000000000000000 ) ) ;
#17896=ORIENTED_EDGE ( 'NONE', *, *, #30326, .T. ) ;
#17899=CARTESIAN_POINT ( 'NONE',  ( 19.99999999999998934, -124.9999999999999432, -162.9999999999999432 ) ) ;
#17901=EDGE_CURVE ( 'NONE', #29621, #4287, #24261, .T. ) ;
#17907=VECTOR ( 'NONE', #22887, 1000.000000000000000 ) ;
#17908=EDGE_CURVE ( 'NONE', #2780, #31630, #23909, .T. ) ;
#17909=EDGE_CURVE ( 'NONE', #26816, #8431, #34612, .T. ) ;
#17912=ORIENTED_EDGE ( 'NONE', *, *, #13869, .F. ) ;
#17913=EDGE_LOOP ( 'NONE', ( #7455, #17294 ) ) ;
#17914=DIRECTION ( 'NONE',  ( 3.469446951953832974E-18, 1.000000000000000000, 7.888609052210116302E-31 ) ) ;
#17915=VECTOR ( 'NONE', #31128, 1000.000000000000000 ) ;
#17917=AXIS2_PLACEMENT_3D ( 'NONE', #12532, #34238, #9849 ) ;
#17919=CARTESIAN_POINT ( 'NONE',  ( -499.9999999999999432, 112.9999999999999574, -187.0000000000000000 ) ) ;
#17921=VERTEX_POINT ( 'NONE', #5043 ) ;
#17923=CARTESIAN_POINT ( 'NONE',  ( -499.9999999999999432, 112.9999999999999574, 155.0000000000000000 ) ) ;
#17924=DIRECTION ( 'NONE',  ( 1.000000000000000000, 3.469446951953834515E-18, 0.000000000000000000 ) ) ;
#17925=VECTOR ( 'NONE', #9743, 1000.000000000000000 ) ;
#17926=CARTESIAN_POINT ( 'NONE',  ( -418.0000000000000000, 105.0000000000000142, -101.9999999999999858 ) ) ;
#17927=CARTESIAN_POINT ( 'NONE',  ( -418.0000000000000000, -105.0000000000000142, 190.9999999999999716 ) ) ;
#17928=ORIENTED_EDGE ( 'NONE', *, *, #25667, .F. ) ;
#17932=EDGE_CURVE ( 'NONE', #6669, #9466, #15940, .T. ) ;
#17934=DIRECTION ( 'NONE',  ( 1.000000000000000000, 0.000000000000000000, 0.000000000000000000 ) ) ;
#17938=LINE ( 'NONE', #31097, #4158 ) ;
#17939=ORIENTED_EDGE ( 'NONE', *, *, #11762, .F. ) ;
#17941=DIRECTION ( 'NONE',  ( 0.000000000000000000, 0.000000000000000000, 1.000000000000000000 ) ) ;
#17943=CARTESIAN_POINT ( 'NONE',  ( 11.99999999999999645, -124.9999999999999432, -162.9999999999999432 ) ) ;
#17948=EDGE_CURVE ( 'NONE', #31845, #32751, #31520, .T. ) ;
#17950=AXIS2_PLACEMENT_3D ( 'NONE', #5993, #11896, #27720 ) ;
#17953=CLOSED_SHELL ( 'NONE', ( #14440, #11716, #8676, #6332, #1324, #21461, #33107, #28896, #26535, #5083, #6298, #14957, #13282, #13113, #30975, #34813, #22552, #33299 ) ) ;
#17956=ORIENTED_EDGE ( 'NONE', *, *, #6366, .F. ) ;
#17959=DIRECTION ( 'NONE',  ( -0.000000000000000000, -1.000000000000000000, -0.000000000000000000 ) ) ;
#17963=CARTESIAN_POINT ( 'NONE',  ( 11.99999999999999645, 112.9999999999999574, -155.0000000000000000 ) ) ;
#17965=ORIENTED_EDGE ( 'NONE', *, *, #68, .T. ) ;
#17966=ORIENTED_EDGE ( 'NONE', *, *, #6002, .F. ) ;
#17972=CARTESIAN_POINT ( 'NONE',  ( -12.00000000000001066, 124.9999999999999716, 187.0000000000000000 ) ) ;
#17973=DIRECTION ( 'NONE',  ( 0.000000000000000000, -0.000000000000000000, 1.000000000000000000 ) ) ;
#17975=LINE ( 'NONE', #4402, #25496 ) ;
#17977=VECTOR ( 'NONE', #25304, 1000.000000000000000 ) ;
#17983=ADVANCED_FACE ( 'NONE', ( #6263 ), #21777, .T. ) ;
#17984=DIRECTION ( 'NONE',  ( -1.000000000000000000, -3.040835319149746528E-31, -1.232595164407830946E-32 ) ) ;
#17989=( NAMED_UNIT ( * ) PLANE_ANGLE_UNIT ( ) SI_UNIT ( $, .RADIAN. ) );
#17996=VECTOR ( 'NONE', #23265, 1000.000000000000000 ) ;
#18001=ORIENTED_EDGE ( 'NONE', *, *, #21553, .F. ) ;
#18003=CARTESIAN_POINT ( 'NONE',  ( -355.0000000000000000, 130.9999999999999716, 130.0000000000000000 ) ) ;
#18005=VECTOR ( 'NONE', #7111, 1000.000000000000000 ) ;
#18010=CARTESIAN_POINT ( 'NONE',  ( -347.0000000000000000, -135.0000000000000000, 126.0000000000000000 ) ) ;
#18020=EDGE_CURVE ( 'NONE', #16015, #1917, #17348, .T. ) ;
#18022=DIRECTION ( 'NONE',  ( 1.000000000000000000, 0.000000000000000000, 0.000000000000000000 ) ) ;
#18034=EDGE_CURVE ( 'NONE', #27889, #19582, #34943, .T. ) ;
#18036=ORIENTED_EDGE ( 'NONE', *, *, #33383, .T. ) ;
#18041=EDGE_LOOP ( 'NONE', ( #19866, #27748, #12164, #1980, #13980, #4719, #15793, #20112 ) ) ;
#18042=ORIENTED_EDGE ( 'NONE', *, *, #33985, .T. ) ;
#18043=LINE ( 'NONE', #24040, #23019 ) ;
#18044=EDGE_CURVE ( 'NONE', #33196, #22205, #34367, .T. ) ;
#18049=VERTEX_POINT ( 'NONE', #14131 ) ;
#18051=DIRECTION ( 'NONE',  ( 1.000000000000000000, 0.000000000000000000, 0.000000000000000000 ) ) ;
#18058=VECTOR ( 'NONE', #15732, 1000.000000000000000 ) ;
#18059=DIRECTION ( 'NONE',  ( -0.000000000000000000, 0.000000000000000000, 1.000000000000000000 ) ) ;
#18065=CARTESIAN_POINT ( 'NONE',  ( -430.0000000000000000, -117.0000000000000000, 126.0000000000000000 ) ) ;
#18070=DIRECTION ( 'NONE',  ( 0.000000000000000000, 0.000000000000000000, -1.000000000000000000 ) ) ;
#18071=ORIENTED_EDGE ( 'NONE', *, *, #22404, .F. ) ;
#18075=VECTOR ( 'NONE', #29278, 1000.000000000000000 ) ;
#18078=EDGE_CURVE ( 'NONE', #6435, #15089, #33157, .T. ) ;
#18082=CIRCLE ( 'NONE', #2703, 8.000000000000007105 ) ;
#18092=CARTESIAN_POINT ( 'NONE',  ( -500.0000000000000000, -145.0000000000000000, 187.0000000000000000 ) ) ;
#18093=DIRECTION ( 'NONE',  ( 1.000000000000000000, 3.040835319149746528E-31, 1.232595164407830946E-32 ) ) ;
#18102=EDGE_LOOP ( 'NONE', ( #25536, #2565 ) ) ;
#18103=ADVANCED_FACE ( 'NONE', ( #9655 ), #3604, .F. ) ;
#18104=VERTEX_POINT ( 'NONE', #20692 ) ;
#18106=CARTESIAN_POINT ( 'NONE',  ( -499.9999999999999432, 112.9999999999999574, -194.9999999999999716 ) ) ;
#18108=VERTEX_POINT ( 'NONE', #9126 ) ;
#18109=DIRECTION ( 'NONE',  ( 0.000000000000000000, 1.000000000000000000, -3.374343856708137958E-53 ) ) ;
#18114=VECTOR ( 'NONE', #32029, 1000.000000000000000 ) ;
#18115=AXIS2_PLACEMENT_3D ( 'NONE', #32854, #13648, #30189 ) ;
#18118=DIRECTION ( 'NONE',  ( 1.000000000000000000, 0.000000000000000000, 0.000000000000000000 ) ) ;
#18124=DIRECTION ( 'NONE',  ( 0.000000000000000000, 1.000000000000000000, 5.053935297177146739E-49 ) ) ;
#18125=CARTESIAN_POINT ( 'NONE',  ( -449.9999999999999432, 113.0000000000000000, 154.9999999999999716 ) ) ;
#18127=VECTOR ( 'NONE', #13011, 1000.000000000000000 ) ;
#18130=ORIENTED_EDGE ( 'NONE', *, *, #23713, .F. ) ;
#18132=VERTEX_POINT ( 'NONE', #28177 ) ;
#18133=DIRECTION ( 'NONE',  ( 2.736911063134582149E-48, -7.888609052210118054E-31, -1.000000000000000000 ) ) ;
#18134=CARTESIAN_POINT ( 'NONE',  ( 11.99999999999999645, 124.9999999999999716, 162.9999999999999716 ) ) ;
#18141=EDGE_LOOP ( 'NONE', ( #15397, #8451, #34092, #8364, #29283, #4093, #1393, #4988 ) ) ;
#18143=CARTESIAN_POINT ( 'NONE',  ( -19.99999999999996092, 125.0000000000000568, 155.0000000000000000 ) ) ;
#18144=AXIS2_PLACEMENT_3D ( 'NONE', #24148, #18832, #2788 ) ;
#18145=ADVANCED_FACE ( 'NONE', ( #25321 ), #12512, .T. ) ;
#18146=EDGE_CURVE ( 'NONE', #22205, #4014, #23353, .T. ) ;
#18147=CARTESIAN_POINT ( 'NONE',  ( -499.9999999999999432, 136.9999999999999432, 194.9999999999999716 ) ) ;
#18152=FACE_OUTER_BOUND ( 'NONE', #17244, .T. ) ;
#18153=FACE_OUTER_BOUND ( 'NONE', #128, .T. ) ;
#18154=DIRECTION ( 'NONE',  ( 0.000000000000000000, -1.000000000000000000, 6.842277657836020854E-49 ) ) ;
#18155=VERTEX_POINT ( 'NONE', #6624 ) ;
#18156=CIRCLE ( 'NONE', #23239, 7.999999999999979572 ) ;
#18158=ORIENTED_EDGE ( 'NONE', *, *, #16852, .F. ) ;
#18159=DIRECTION ( 'NONE',  ( 0.000000000000000000, 0.000000000000000000, -1.000000000000000000 ) ) ;
#18162=LINE ( 'NONE', #4578, #21329 ) ;
#18163=CARTESIAN_POINT ( 'NONE',  ( -355.0000000000000000, 134.9999999999999716, 113.9999999999999858 ) ) ;
#18165=AXIS2_PLACEMENT_3D ( 'NONE', #5057, #443, #5747 ) ;
#18166=ORIENTED_EDGE ( 'NONE', *, *, #4516, .F. ) ;
#18169=LINE ( 'NONE', #4588, #15840 ) ;
#18171=DIRECTION ( 'NONE',  ( -0.000000000000000000, -0.000000000000000000, -1.000000000000000000 ) ) ;
#18172=FACE_OUTER_BOUND ( 'NONE', #14089, .T. ) ;
#18176=EDGE_CURVE ( 'NONE', #639, #9452, #17165, .T. ) ;
#18179=ORIENTED_EDGE ( 'NONE', *, *, #32786, .T. ) ;
#18180=ORIENTED_EDGE ( 'NONE', *, *, #33747, .F. ) ;
#18182=ORIENTED_EDGE ( 'NONE', *, *, #4155, .F. ) ;
#18185=CARTESIAN_POINT ( 'NONE',  ( -442.0000000000000000, -105.0000000000000142, 104.0000000000000142 ) ) ;
#18187=AXIS2_PLACEMENT_3D ( 'NONE', #24834, #25000, #17520 ) ;
#18188=DIRECTION ( 'NONE',  ( 1.000000000000000000, 0.000000000000000000, 0.000000000000000000 ) ) ;
#18190=DIRECTION ( 'NONE',  ( 0.000000000000000000, 0.000000000000000000, 1.000000000000000000 ) ) ;
#18191=DIRECTION ( 'NONE',  ( 1.000000000000000000, 0.000000000000000000, 0.000000000000000000 ) ) ;
#18194=CARTESIAN_POINT ( 'NONE',  ( -442.0000000000000000, -105.0000000000000142, 104.0000000000000142 ) ) ;
#18196=CARTESIAN_POINT ( 'NONE',  ( 11.99999999999995559, -134.9999999999999716, -194.9999999999999432 ) ) ;
#18201=VERTEX_POINT ( 'NONE', #15012 ) ;
#18202=EDGE_LOOP ( 'NONE', ( #33009, #14423, #1208, #15096 ) ) ;
#18203=VECTOR ( 'NONE', #18344, 1000.000000000000000 ) ;
#18209=ORIENTED_EDGE ( 'NONE', *, *, #8348, .F. ) ;
#18211=ADVANCED_FACE ( 'NONE', ( #30844 ), #33509, .F. ) ;
#18213=DIRECTION ( 'NONE',  ( 1.000000000000000000, 0.000000000000000000, 0.000000000000000000 ) ) ;
#18214=DIRECTION ( 'NONE',  ( -0.000000000000000000, 0.000000000000000000, 1.000000000000000000 ) ) ;
#18215=ORIENTED_EDGE ( 'NONE', *, *, #15652, .F. ) ;
#18216=VERTEX_POINT ( 'NONE', #25852 ) ;
#18219=EDGE_CURVE ( 'NONE', #25754, #28711, #14523, .T. ) ;
#18222=CARTESIAN_POINT ( 'NONE',  ( -499.9999999999999432, -113.0000000000000000, -194.9999999999999716 ) ) ;
#18223=ORIENTED_EDGE ( 'NONE', *, *, #10313, .T. ) ;
#18226=EDGE_CURVE ( 'NONE', #27398, #24475, #26439, .T. ) ;
#18227=VERTEX_POINT ( 'NONE', #17347 ) ;
#18229=FACE_OUTER_BOUND ( 'NONE', #14139, .T. ) ;
#18230=EDGE_CURVE ( 'NONE', #7322, #18350, #17864, .T. ) ;
#18233=DIRECTION ( 'NONE',  ( 1.000000000000000000, 0.000000000000000000, -1.232595164407831220E-32 ) ) ;
#18234=DIRECTION ( 'NONE',  ( -0.000000000000000000, 0.000000000000000000, 1.000000000000000000 ) ) ;
#18239=DIRECTION ( 'NONE',  ( -1.300283923313630633E-47, 0.000000000000000000, 1.000000000000000000 ) ) ;
#18245=CARTESIAN_POINT ( 'NONE',  ( -20.00000000000007461, 112.9999999999999574, -187.0000000000000000 ) ) ;
#18247=ORIENTED_EDGE ( 'NONE', *, *, #10516, .T. ) ;
#18251=CARTESIAN_POINT ( 'NONE',  ( 11.99999999999999645, 144.9999999999999716, 190.9999999999999716 ) ) ;
#18261=EDGE_LOOP ( 'NONE', ( #3349, #21859, #23269, #22946, #1266, #2064, #18215, #19219 ) ) ;
#18263=CIRCLE ( 'NONE', #14274, 3.999999999999976019 ) ;
#18266=DIRECTION ( 'NONE',  ( 1.000000000000000000, 0.000000000000000000, 0.000000000000000000 ) ) ;
#18270=CARTESIAN_POINT ( 'NONE',  ( -430.0000000000000000, -119.0000000000000000, 111.9999999999999858 ) ) ;
#18272=ORIENTED_EDGE ( 'NONE', *, *, #8464, .T. ) ;
#18273=PLANE ( 'NONE',  #12123 ) ;
#18274=ORIENTED_EDGE ( 'NONE', *, *, #22391, .F. ) ;
#18275=PLANE ( 'NONE',  #16691 ) ;
#18276=ORIENTED_EDGE ( 'NONE', *, *, #31894, .T. ) ;
#18278=LINE ( 'NONE', #9562, #19964 ) ;
#18281=EDGE_CURVE ( 'NONE', #23168, #25561, #16066, .T. ) ;
#18282=AXIS2_PLACEMENT_3D ( 'NONE', #24087, #24123, #8077 ) ;
#18285=DIRECTION ( 'NONE',  ( 0.000000000000000000, 1.000000000000000000, 1.224646799147353207E-16 ) ) ;
#18289=EDGE_CURVE ( 'NONE', #25102, #27224, #23706, .T. ) ;
#18291=AXIS2_PLACEMENT_3D ( 'NONE', #30075, #24720, #11214 ) ;
#18294=EDGE_LOOP ( 'NONE', ( #27414, #11109, #1163, #21888 ) ) ;
#18296=ORIENTED_EDGE ( 'NONE', *, *, #34835, .F. ) ;
#18300=DIRECTION ( 'NONE',  ( -3.040835319149746528E-31, -1.000000000000000000, 0.000000000000000000 ) ) ;
#18304=ORIENTED_EDGE ( 'NONE', *, *, #24953, .T. ) ;
#18306=ORIENTED_EDGE ( 'NONE', *, *, #2646, .F. ) ;
#18309=VECTOR ( 'NONE', #33161, 1000.000000000000000 ) ;
#18312=EDGE_CURVE ( 'NONE', #9284, #27942, #7142, .T. ) ;
#18314=DIRECTION ( 'NONE',  ( 1.000000000000000000, 0.000000000000000000, 0.000000000000000000 ) ) ;
#18317=PLANE ( 'NONE',  #21394 ) ;
#18319=VECTOR ( 'NONE', #29694, 1000.000000000000000 ) ;
#18320=DIRECTION ( 'NONE',  ( -0.000000000000000000, 1.000000000000000000, -0.000000000000000000 ) ) ;
#18322=VECTOR ( 'NONE', #31256, 1000.000000000000000 ) ;
#18328=FACE_OUTER_BOUND ( 'NONE', #14358, .T. ) ;
#18329=ORIENTED_EDGE ( 'NONE', *, *, #6102, .T. ) ;
#18333=ORIENTED_EDGE ( 'NONE', *, *, #18146, .F. ) ;
#18334=EDGE_CURVE ( 'NONE', #23700, #7091, #18043, .T. ) ;
#18335=EDGE_CURVE ( 'NONE', #13338, #34601, #9406, .T. ) ;
#18336=ORIENTED_EDGE ( 'NONE', *, *, #22907, .T. ) ;
#18339=ORIENTED_EDGE ( 'NONE', *, *, #1161, .F. ) ;
#18340=EDGE_CURVE ( 'NONE', #21426, #13149, #7494, .T. ) ;
#18342=VECTOR ( 'NONE', #22329, 1000.000000000000000 ) ;
#18344=DIRECTION ( 'NONE',  ( -0.000000000000000000, -1.000000000000000000, -0.000000000000000000 ) ) ;
#18348=DIRECTION ( 'NONE',  ( -0.000000000000000000, -0.000000000000000000, 1.000000000000000000 ) ) ;
#18349=PLANE ( 'NONE',  #19819 ) ;
#18350=VERTEX_POINT ( 'NONE', #34388 ) ;
#18353=ORIENTED_EDGE ( 'NONE', *, *, #21355, .T. ) ;
#18354=LINE ( 'NONE', #10510, #18127 ) ;
#18355=LINE ( 'NONE', #18185, #8020 ) ;
#18357=CARTESIAN_POINT ( 'NONE',  ( -499.9999999999999432, 136.9999999999999432, 155.0000000000000000 ) ) ;
#18358=ORIENTED_EDGE ( 'NONE', *, *, #25662, .F. ) ;
#18361=PLANE ( 'NONE',  #4603 ) ;
#18362=CARTESIAN_POINT ( 'NONE',  ( 19.99999999999996092, -134.9999999999999716, 162.9999999999999716 ) ) ;
#18364=DIRECTION ( 'NONE',  ( 1.000000000000000000, 0.000000000000000000, 0.000000000000000000 ) ) ;
#18366=CIRCLE ( 'NONE', #16081, 7.999999999999979572 ) ;
#18368=CIRCLE ( 'NONE', #23455, 3.999999999999976019 ) ;
#18369=DIRECTION ( 'NONE',  ( 0.000000000000000000, 2.309213040847544338E-50, 1.000000000000000000 ) ) ;
#18371=CARTESIAN_POINT ( 'NONE',  ( 19.99999999999998934, -145.0000000000000000, 187.0000000000000000 ) ) ;
#18375=EDGE_CURVE ( 'NONE', #13276, #11080, #11067, .T. ) ;
#18376=ORIENTED_EDGE ( 'NONE', *, *, #4536, .T. ) ;
#18379=EDGE_LOOP ( 'NONE', ( #15600, #9718, #4820, #21160 ) ) ;
#18381=EDGE_LOOP ( 'NONE', ( #22216, #9968, #2931, #13914 ) ) ;
#18383=VERTEX_POINT ( 'NONE', #29749 ) ;
#18388=AXIS2_PLACEMENT_3D ( 'NONE', #18839, #5284, #16174 ) ;
#18389=FACE_OUTER_BOUND ( 'NONE', #18764, .T. ) ;
#18390=ORIENTED_EDGE ( 'NONE', *, *, #18340, .F. ) ;
#18391=VERTEX_POINT ( 'NONE', #24564 ) ;
#18392=AXIS2_PLACEMENT_3D ( 'NONE', #13755, #16085, #2535 ) ;
#18393=CYLINDRICAL_SURFACE ( 'NONE', #30488, 7.999999999999979572 ) ;
#18396=DIRECTION ( 'NONE',  ( -1.000000000000000000, 0.000000000000000000, -5.546364386991661285E-52 ) ) ;
#18402=DIRECTION ( 'NONE',  ( 0.000000000000000000, 1.000000000000000000, 1.224646799147353207E-16 ) ) ;
#18406=AXIS2_PLACEMENT_3D ( 'NONE', #19911, #33418, #22577 ) ;
#18408=DIRECTION ( 'NONE',  ( 1.000000000000000000, 0.000000000000000000, -1.232595164407831220E-32 ) ) ;
#18410=CARTESIAN_POINT ( 'NONE',  ( -442.0000000000000000, 124.9999999999999432, -155.0000000000000000 ) ) ;
#18411=DIRECTION ( 'NONE',  ( 0.000000000000000000, -1.000000000000000000, 0.000000000000000000 ) ) ;
#18412=DIRECTION ( 'NONE',  ( 1.000000000000000000, 0.000000000000000000, -1.232595164407831220E-32 ) ) ;
#18416=VECTOR ( 'NONE', #28024, 1000.000000000000000 ) ;
#18419=PLANE ( 'NONE',  #8660 ) ;
#18421=EDGE_CURVE ( 'NONE', #33196, #8817, #21, .T. ) ;
#18423=ORIENTED_EDGE ( 'NONE', *, *, #7584, .T. ) ;
#18424=LINE ( 'NONE', #31580, #32642 ) ;
#18427=DIRECTION ( 'NONE',  ( -0.000000000000000000, -1.131431318426415506E-52, -1.000000000000000000 ) ) ;
#18428=EDGE_CURVE ( 'NONE', #18484, #18104, #22270, .T. ) ;
#18429=VECTOR ( 'NONE', #17215, 1000.000000000000000 ) ;
#18430=CARTESIAN_POINT ( 'NONE',  ( -19.99999999999998934, -112.9999999999999858, 155.0000000000000000 ) ) ;
#18431=CARTESIAN_POINT ( 'NONE',  ( -355.0000000000000000, 114.9999999999999716, 126.0000000000000000 ) ) ;
#18438=LINE ( 'NONE', #34801, #27909 ) ;
#18442=CARTESIAN_POINT ( 'NONE',  ( -500.0000000000000000, -109.0000000000000142, 162.9999999999999716 ) ) ;
#18443=VECTOR ( 'NONE', #8578, 1000.000000000000000 ) ;
#18444=CIRCLE ( 'NONE', #12200, 3.999999999999948042 ) ;
#18445=FACE_OUTER_BOUND ( 'NONE', #49, .T. ) ;
#18446=VERTEX_POINT ( 'NONE', #10886 ) ;
#18447=CIRCLE ( 'NONE', #29810, 4.750000000000004441 ) ;
#18450=FACE_OUTER_BOUND ( 'NONE', #2570, .T. ) ;
#18451=ORIENTED_EDGE ( 'NONE', *, *, #27373, .T. ) ;
#18453=ORIENTED_EDGE ( 'NONE', *, *, #17908, .T. ) ;
#18454=DIRECTION ( 'NONE',  ( 0.000000000000000000, 0.000000000000000000, 1.000000000000000000 ) ) ;
#18456=CARTESIAN_POINT ( 'NONE',  ( -499.9999999999999432, 112.9999999999999574, 155.0000000000000000 ) ) ;
#18457=CARTESIAN_POINT ( 'NONE',  ( -20.00000000000007461, 140.9999999999999716, 162.9999999999999716 ) ) ;
#18458=DIRECTION ( 'NONE',  ( -0.000000000000000000, -1.000000000000000000, -0.000000000000000000 ) ) ;
#18462=FACE_OUTER_BOUND ( 'NONE', #10381, .T. ) ;
#18464=EDGE_CURVE ( 'NONE', #15074, #10505, #8730, .T. ) ;
#18465=VECTOR ( 'NONE', #7451, 1000.000000000000000 ) ;
#18467=VERTEX_POINT ( 'NONE', #16953 ) ;
#18469=VECTOR ( 'NONE', #45, 1000.000000000000000 ) ;
#18470=EDGE_CURVE ( 'NONE', #15934, #20393, #14267, .T. ) ;
#18471=EDGE_CURVE ( 'NONE', #10892, #6969, #28698, .T. ) ;
#18477=EDGE_LOOP ( 'NONE', ( #2361, #26654, #8165, #26874 ) ) ;
#18478=DIRECTION ( 'NONE',  ( 0.000000000000000000, -1.000000000000000000, -2.309213040847544338E-50 ) ) ;
#18482=DIRECTION ( 'NONE',  ( 0.000000000000000000, 0.000000000000000000, -1.000000000000000000 ) ) ;
#18484=VERTEX_POINT ( 'NONE', #13730 ) ;
#18487=CARTESIAN_POINT ( 'NONE',  ( -355.0000000000000000, -117.0000000000000000, 113.9999999999999858 ) ) ;
#18490=AXIS2_PLACEMENT_3D ( 'NONE', #12732, #18427, #34435 ) ;
#18492=CYLINDRICAL_SURFACE ( 'NONE', #29655, 3.999999999999976019 ) ;
#18493=LINE ( 'NONE', #29331, #26006 ) ;
#18494=FACE_OUTER_BOUND ( 'NONE', #4947, .T. ) ;
#18495=ORIENTED_EDGE ( 'NONE', *, *, #21380, .F. ) ;
#18496=VECTOR ( 'NONE', #6370, 1000.000000000000000 ) ;
#18497=DIRECTION ( 'NONE',  ( 1.848892746611746419E-32, 6.842277657836020854E-49, -1.000000000000000000 ) ) ;
#18498=DIRECTION ( 'NONE',  ( 0.000000000000000000, -1.000000000000000000, 1.131431318426415506E-52 ) ) ;
#18499=CARTESIAN_POINT ( 'NONE',  ( -355.0000000000000000, 135.0000000000000000, 130.0000000000000000 ) ) ;
#18502=CIRCLE ( 'NONE', #21328, 4.750000000000004441 ) ;
#18503=EDGE_CURVE ( 'NONE', #35039, #10023, #13372, .T. ) ;
#18504=AXIS2_PLACEMENT_3D ( 'NONE', #9075, #25078, #11764 ) ;
#18506=ORIENTED_EDGE ( 'NONE', *, *, #7857, .F. ) ;
#18508=CLOSED_SHELL ( 'NONE', ( #22171, #11133, #20628, #27601, #21842, #30706, #29494, #26831, #10666, #22042, #16315, #2974, #22477, #13281, #1794, #31461, #16001, #29594 ) ) ;
#18516=ORIENTED_EDGE ( 'NONE', *, *, #23509, .T. ) ;
#18517=EDGE_CURVE ( 'NONE', #1469, #5175, #8912, .T. ) ;
#18523=CARTESIAN_POINT ( 'NONE',  ( -15.99999999999998579, 75.55999999999990280, -172.9900000000000091 ) ) ;
#18524=DIRECTION ( 'NONE',  ( 0.000000000000000000, 1.000000000000000000, 5.145227585319922065E-49 ) ) ;
#18529=ORIENTED_EDGE ( 'NONE', *, *, #9275, .T. ) ;
#18532=FACE_OUTER_BOUND ( 'NONE', #22493, .T. ) ;
#18537=EDGE_CURVE ( 'NONE', #5880, #31793, #31320, .T. ) ;
#18540=ORIENTED_EDGE ( 'NONE', *, *, #24210, .F. ) ;
#18541=ADVANCED_FACE ( 'NONE', ( #4078 ), #6930, .T. ) ;
#18542=ADVANCED_FACE ( 'NONE', ( #17820 ), #25626, .T. ) ;
#18543=VECTOR ( 'NONE', #6680, 1000.000000000000000 ) ;
#18544=DIRECTION ( 'NONE',  ( -0.000000000000000000, 1.000000000000000000, -0.000000000000000000 ) ) ;
#18546=EDGE_LOOP ( 'NONE', ( #16112, #13783, #12456, #18247 ) ) ;
#18548=CARTESIAN_POINT ( 'NONE',  ( -442.0000000000000000, 105.0000000000000142, 155.0000000000000000 ) ) ;
#18552=LINE ( 'NONE', #15882, #1482 ) ;
#18555=FACE_OUTER_BOUND ( 'NONE', #7664, .T. ) ;
#18557=CARTESIAN_POINT ( 'NONE',  ( 11.99999999999999645, 144.9999999999999716, -194.9999999999999432 ) ) ;
#18559=ORIENTED_EDGE ( 'NONE', *, *, #24746, .T. ) ;
#18562=VERTEX_POINT ( 'NONE', #31161 ) ;
#18568=VECTOR ( 'NONE', #28329, 1000.000000000000000 ) ;
#18579=CARTESIAN_POINT ( 'NONE',  ( -12.00000000000001243, 144.9999999999999716, -154.9999999999999716 ) ) ;
#18583=PLANE ( 'NONE',  #16937 ) ;
#18585=EDGE_CURVE ( 'NONE', #5208, #169, #864, .T. ) ;
#18587=DIRECTION ( 'NONE',  ( -1.000000000000000000, 0.000000000000000000, 0.000000000000000000 ) ) ;
#18590=CARTESIAN_POINT ( 'NONE',  ( -20.00000000000007461, 136.9999999999999432, 187.0000000000000000 ) ) ;
#18591=EDGE_LOOP ( 'NONE', ( #7427, #10732, #22606, #30710 ) ) ;
#18593=DIRECTION ( 'NONE',  ( -1.000000000000000000, -3.469446951953834515E-18, 0.000000000000000000 ) ) ;
#18596=CARTESIAN_POINT ( 'NONE',  ( 12.00000000000003730, -115.0000000000000000, -154.9999999999999716 ) ) ;
#18598=ORIENTED_EDGE ( 'NONE', *, *, #16889, .F. ) ;
#18602=CARTESIAN_POINT ( 'NONE',  ( -442.0000000000000000, -105.0000000000000142, 155.0000000000000000 ) ) ;
#18603=VECTOR ( 'NONE', #5756, 1000.000000000000000 ) ;
#18604=AXIS2_PLACEMENT_3D ( 'NONE', #14055, #2659, #22063 ) ;
#18605=STYLED_ITEM('',(#35254),#11180);
#18606=DIRECTION ( 'NONE',  ( 0.000000000000000000, 1.000000000000000000, 1.224646799147353207E-16 ) ) ;
#18607=FACE_OUTER_BOUND ( 'NONE', #12855, .T. ) ;
#18609=ORIENTED_EDGE ( 'NONE', *, *, #29387, .T. ) ;
#18610=LINE ( 'NONE', #7908, #14000 ) ;
#18611=CARTESIAN_POINT ( 'NONE',  ( -19.99999999999998934, -134.9999999999999716, 162.9999999999999716 ) ) ;
#18618=EDGE_CURVE ( 'NONE', #25432, #30178, #6222, .T. ) ;
#18619=CYLINDRICAL_SURFACE ( 'NONE', #18165, 4.000000000000003553 ) ;
#18620=ORIENTED_EDGE ( 'NONE', *, *, #34751, .T. ) ;
#18621=VECTOR ( 'NONE', #19913, 1000.000000000000000 ) ;
#18623=DIRECTION ( 'NONE',  ( 1.000000000000000000, 0.000000000000000000, -1.232595164407831220E-32 ) ) ;
#18624=CARTESIAN_POINT ( 'NONE',  ( -19.99999999999998934, -134.9999999999999716, 162.9999999999999716 ) ) ;
#18625=DIRECTION ( 'NONE',  ( 0.000000000000000000, 1.310824597558155437E-49, 1.000000000000000000 ) ) ;
#18626=ORIENTED_EDGE ( 'NONE', *, *, #16173, .F. ) ;
#18628=ORIENTED_EDGE ( 'NONE', *, *, #33674, .T. ) ;
#18629=AXIS2_PLACEMENT_3D ( 'NONE', #21919, #7724, #5050 ) ;
#18630=CARTESIAN_POINT ( 'NONE',  ( -442.0000000000000000, -105.0000000000000142, -77.99999999999997158 ) ) ;
#18634=CARTESIAN_POINT ( 'NONE',  ( 11.99999999999999645, 124.9999999999999716, 155.0000000000000000 ) ) ;
#18640=VERTEX_POINT ( 'NONE', #1260 ) ;
#18643=EDGE_LOOP ( 'NONE', ( #8762, #7011, #17349, #6269 ) ) ;
#18652=ORIENTED_EDGE ( 'NONE', *, *, #26906, .F. ) ;
#18655=DIRECTION ( 'NONE',  ( 1.000000000000000000, 0.000000000000000000, -1.232595164407831220E-32 ) ) ;
#18656=ADVANCED_FACE ( 'NONE', ( #22970 ), #33825, .T. ) ;
#18657=DIRECTION ( 'NONE',  ( 1.000000000000000000, 0.000000000000000000, 0.000000000000000000 ) ) ;
#18658=AXIS2_PLACEMENT_3D ( 'NONE', #18523, #29357, #4952 ) ;
#18661=CARTESIAN_POINT ( 'NONE',  ( -418.0000000000000568, 105.0000000000000142, -105.9999999999999574 ) ) ;
#18663=CARTESIAN_POINT ( 'NONE',  ( -418.0000000000000000, -112.9999999999999858, 155.0000000000000000 ) ) ;
#18664=ORIENTED_EDGE ( 'NONE', *, *, #2322, .T. ) ;
#18667=EDGE_CURVE ( 'NONE', #33325, #29191, #15099, .T. ) ;
#18668=CARTESIAN_POINT ( 'NONE',  ( 12.00000000000001066, -105.0000000000000142, -155.0000000000000000 ) ) ;
#18669=VECTOR ( 'NONE', #780, 1000.000000000000000 ) ;
#18671=ORIENTED_EDGE ( 'NONE', *, *, #34523, .T. ) ;
#18672=ADVANCED_FACE ( 'NONE', ( #5094 ), #13883, .F. ) ;
#18673=EDGE_CURVE ( 'NONE', #11377, #13666, #29844, .T. ) ;
#18674=DIRECTION ( 'NONE',  ( -0.000000000000000000, -0.000000000000000000, -1.000000000000000000 ) ) ;
#18680=ORIENTED_EDGE ( 'NONE', *, *, #12341, .F. ) ;
#18681=DIRECTION ( 'NONE',  ( 0.000000000000000000, 0.000000000000000000, 1.000000000000000000 ) ) ;
#18685=AXIS2_PLACEMENT_3D ( 'NONE', #9261, #30799, #19952 ) ;
#18693=DIRECTION ( 'NONE',  ( 0.000000000000000000, 0.000000000000000000, -1.000000000000000000 ) ) ;
#18696=ORIENTED_EDGE ( 'NONE', *, *, #34790, .T. ) ;
#18698=AXIS2_PLACEMENT_3D ( 'NONE', #8701, #30424, #3715 ) ;
#18701=AXIS2_PLACEMENT_3D ( 'NONE', #10769, #26424, #13090 ) ;
#18702=ORIENTED_EDGE ( 'NONE', *, *, #24584, .T. ) ;
#18703=ORIENTED_EDGE ( 'NONE', *, *, #18537, .T. ) ;
#18708=DIRECTION ( 'NONE',  ( 1.000000000000000000, 0.000000000000000000, 1.300283923313630633E-47 ) ) ;
#18709=VERTEX_POINT ( 'NONE', #8301 ) ;
#18710=DIRECTION ( 'NONE',  ( 0.000000000000000000, 1.000000000000000000, 1.224646799147353207E-16 ) ) ;
#18711=EDGE_CURVE ( 'NONE', #13597, #25101, #5417, .T. ) ;
#18712=EDGE_CURVE ( 'NONE', #34350, #726, #10455, .T. ) ;
#18714=DIRECTION ( 'NONE',  ( 0.000000000000000000, 0.000000000000000000, -1.000000000000000000 ) ) ;
#18715=ORIENTED_EDGE ( 'NONE', *, *, #13540, .T. ) ;
#18719=MECHANICAL_DESIGN_GEOMETRIC_PRESENTATION_REPRESENTATION('',(#17028),#4449);
#18720=CARTESIAN_POINT ( 'NONE',  ( -500.0000000000000000, -113.0000000000000000, 155.0000000000000000 ) ) ;
#18721=DIRECTION ( 'NONE',  ( 0.000000000000000000, 0.000000000000000000, 1.000000000000000000 ) ) ;
#18722=DIRECTION ( 'NONE',  ( 0.000000000000000000, 0.000000000000000000, 1.000000000000000000 ) ) ;
#18723=DIRECTION ( 'NONE',  ( 0.000000000000000000, 0.000000000000000000, -1.000000000000000000 ) ) ;
#18726=ORIENTED_EDGE ( 'NONE', *, *, #1413, .T. ) ;
#18729=EDGE_LOOP ( 'NONE', ( #34404, #959, #20958, #22170, #21249, #13096, #4678, #12692, #3954, #5635 ) ) ;
#18731=ORIENTED_EDGE ( 'NONE', *, *, #27878, .F. ) ;
#18741=EDGE_CURVE ( 'NONE', #19872, #26754, #12260, .T. ) ;
#18742=AXIS2_PLACEMENT_3D ( 'NONE', #3797, #1145, #3098 ) ;
#18745=ORIENTED_EDGE ( 'NONE', *, *, #17660, .F. ) ;
#18750=CARTESIAN_POINT ( 'NONE',  ( -442.0000000000000000, 113.0000000000000000, -155.0000000000000000 ) ) ;
#18755=FACE_OUTER_BOUND ( 'NONE', #30064, .T. ) ;
#18756=VECTOR ( 'NONE', #22685, 1000.000000000000000 ) ;
#18757=EDGE_CURVE ( 'NONE', #28398, #21809, #28826, .T. ) ;
#18764=EDGE_LOOP ( 'NONE', ( #21823, #13367, #20102, #29497 ) ) ;
#18768=ORIENTED_EDGE ( 'NONE', *, *, #6369, .T. ) ;
#18769=DIRECTION ( 'NONE',  ( 1.000000000000000000, -0.000000000000000000, -0.000000000000000000 ) ) ;
#18772=EDGE_CURVE ( 'NONE', #32250, #16547, #7947, .T. ) ;
#18777=CARTESIAN_POINT ( 'NONE',  ( 11.99999999999999645, 134.9999999999999432, -186.9999999999999716 ) ) ;
#18779=DIRECTION ( 'NONE',  ( 1.300283923313630633E-47, 0.000000000000000000, 1.000000000000000000 ) ) ;
#18780=ORIENTED_EDGE ( 'NONE', *, *, #34607, .F. ) ;
#18783=EDGE_CURVE ( 'NONE', #32668, #31670, #19091, .T. ) ;
#18784=DIRECTION ( 'NONE',  ( -1.000000000000000000, 0.000000000000000000, -5.546364386991661285E-52 ) ) ;
#18790=VERTEX_POINT ( 'NONE', #19002 ) ;
#18795=CARTESIAN_POINT ( 'NONE',  ( 11.99999999999999645, 144.9999999999999716, -190.9999999999999432 ) ) ;
#18797=DIRECTION ( 'NONE',  ( 0.000000000000000000, 1.131431318426415506E-52, 1.000000000000000000 ) ) ;
#18798=ORIENTED_EDGE ( 'NONE', *, *, #20238, .T. ) ;
#18802=( NAMED_UNIT ( * ) SI_UNIT ( $, .STERADIAN. ) SOLID_ANGLE_UNIT ( ) );
#18803=VERTEX_POINT ( 'NONE', #24476 ) ;
#18804=PLANE ( 'NONE',  #84 ) ;
#18806=EDGE_CURVE ( 'NONE', #9216, #2852, #29876, .T. ) ;
#18808=AXIS2_PLACEMENT_3D ( 'NONE', #26286, #34839, #29321 ) ;
#18810=EDGE_CURVE ( 'NONE', #24390, #4119, #14187, .T. ) ;
#18813=DIRECTION ( 'NONE',  ( 1.000000000000000000, -0.000000000000000000, -0.000000000000000000 ) ) ;
#18819=AXIS2_PLACEMENT_3D ( 'NONE', #3792, #15194, #26202 ) ;
#18821=ORIENTED_EDGE ( 'NONE', *, *, #15306, .T. ) ;
#18827=DIRECTION ( 'NONE',  ( 1.000000000000000000, 0.000000000000000000, -1.232595164407831220E-32 ) ) ;
#18832=DIRECTION ( 'NONE',  ( 1.000000000000000000, 0.000000000000000000, 5.546364386991661285E-52 ) ) ;
#18838=VERTEX_POINT ( 'NONE', #3480 ) ;
#18839=CARTESIAN_POINT ( 'NONE',  ( -418.0000000000000000, 124.9999999999999574, -194.9999999999999716 ) ) ;
#18841=LINE ( 'NONE', #321, #13209 ) ;
#18842=CYLINDRICAL_SURFACE ( 'NONE', #22978, 7.999999999999979572 ) ;
#18844=ORIENTED_EDGE ( 'NONE', *, *, #11535, .T. ) ;
#18847=DIRECTION ( 'NONE',  ( 1.000000000000000000, 0.000000000000000000, 0.000000000000000000 ) ) ;
#18849=DIRECTION ( 'NONE',  ( 0.000000000000000000, 0.000000000000000000, -1.000000000000000000 ) ) ;
#18850=CARTESIAN_POINT ( 'NONE',  ( -500.0000000000000000, 144.9999999999999716, 155.0000000000000000 ) ) ;
#18851=AXIS2_PLACEMENT_3D ( 'NONE', #13369, #8536, #10699 ) ;
#18855=ORIENTED_EDGE ( 'NONE', *, *, #9731, .F. ) ;
#18859=ORIENTED_EDGE ( 'NONE', *, *, #32190, .F. ) ;
#18862=DIRECTION ( 'NONE',  ( -1.000000000000000000, 0.000000000000000000, -5.546364386991661285E-52 ) ) ;
#18864=EDGE_LOOP ( 'NONE', ( #28738, #28192, #16826, #12706 ) ) ;
#18865=DIRECTION ( 'NONE',  ( 0.000000000000000000, 2.309213040847544338E-50, 1.000000000000000000 ) ) ;
#18866=ADVANCED_FACE ( 'NONE', ( #33559 ), #3310, .F. ) ;
#18868=CARTESIAN_POINT ( 'NONE',  ( -12.00000000000001066, -64.99999999999997158, -175.0000000000000000 ) ) ;
#18870=AXIS2_PLACEMENT_3D ( 'NONE', #2832, #3716, #884 ) ;
#18875=ORIENTED_EDGE ( 'NONE', *, *, #31323, .F. ) ;
#18880=ORIENTED_EDGE ( 'NONE', *, *, #26385, .F. ) ;
#18883=VERTEX_POINT ( 'NONE', #2952 ) ;
#18885=DIRECTION ( 'NONE',  ( 0.000000000000000000, 1.310824597558155437E-49, 1.000000000000000000 ) ) ;
#18889=DIRECTION ( 'NONE',  ( -3.040835319149746090E-31, -1.000000000000000000, 0.000000000000000000 ) ) ;
#18900=ORIENTED_EDGE ( 'NONE', *, *, #27703, .F. ) ;
#18909=CARTESIAN_POINT ( 'NONE',  ( -442.0000000000000000, -105.0000000000000142, 107.9999999999999858 ) ) ;
#18910=ORIENTED_EDGE ( 'NONE', *, *, #15161, .T. ) ;
#18912=DIRECTION ( 'NONE',  ( -1.000000000000000000, -3.040835319149746090E-31, -1.232595164407830946E-32 ) ) ;
#18914=CARTESIAN_POINT ( 'NONE',  ( -12.00000000000003908, -134.9999999999999716, -162.9999999999999432 ) ) ;
#18915=LINE ( 'NONE', #398, #34713 ) ;
#18921=CARTESIAN_POINT ( 'NONE',  ( -361.0000000000000000, 124.9999999999999432, 164.9999999999999716 ) ) ;
#18922=VECTOR ( 'NONE', #28294, 1000.000000000000000 ) ;
#18923=AXIS2_PLACEMENT_3D ( 'NONE', #25704, #31229, #20547 ) ;
#18929=FACE_OUTER_BOUND ( 'NONE', #14909, .T. ) ;
#18930=EDGE_CURVE ( 'NONE', #28532, #29779, #22011, .T. ) ;
#18931=ADVANCED_FACE ( 'NONE', ( #30188 ), #6144, .T. ) ;
#18935=DIRECTION ( 'NONE',  ( 0.000000000000000000, 0.000000000000000000, -1.000000000000000000 ) ) ;
#18938=LINE ( 'NONE', #32093, #2964 ) ;
#18939=ORIENTED_EDGE ( 'NONE', *, *, #30452, .F. ) ;
#18941=AXIS2_PLACEMENT_3D ( 'NONE', #19541, #495, #24860 ) ;
#18943=ADVANCED_FACE ( 'NONE', ( #24843 ), #476, .T. ) ;
#18944=EDGE_CURVE ( 'NONE', #28271, #31232, #6845, .T. ) ;
#18945=CIRCLE ( 'NONE', #6981, 4.750000000000004441 ) ;
#18946=ORIENTED_EDGE ( 'NONE', *, *, #3107, .T. ) ;
#18947=DIRECTION ( 'NONE',  ( 0.000000000000000000, 1.000000000000000000, -5.053935297177146739E-49 ) ) ;
#18950=DIRECTION ( 'NONE',  ( 1.000000000000000000, 0.000000000000000000, 0.000000000000000000 ) ) ;
#18952=DIRECTION ( 'NONE',  ( 0.000000000000000000, 1.000000000000000000, -3.374343856708137958E-53 ) ) ;
#18956=CARTESIAN_POINT ( 'NONE',  ( -20.00000000000001776, -113.0000000000000000, 162.9999999999999716 ) ) ;
#18957=( LENGTH_UNIT ( ) NAMED_UNIT ( * ) SI_UNIT ( .MILLI., .METRE. ) );
#18962=FACE_OUTER_BOUND ( 'NONE', #11378, .T. ) ;
#18967=EDGE_CURVE ( 'NONE', #15089, #3779, #34441, .T. ) ;
#18973=VECTOR ( 'NONE', #30787, 1000.000000000000000 ) ;
#18976=DIRECTION ( 'NONE',  ( 1.000000000000000000, 0.000000000000000000, 0.000000000000000000 ) ) ;
#18977=DIRECTION ( 'NONE',  ( 0.000000000000000000, 1.131431318426415506E-52, 1.000000000000000000 ) ) ;
#18978=CARTESIAN_POINT ( 'NONE',  ( -15.99999999999998579, 112.9999999999999574, 155.0000000000000000 ) ) ;
#18979=ADVANCED_FACE ( 'NONE', ( #4177 ), #10057, .T. ) ;
#18980=EDGE_CURVE ( 'NONE', #7133, #11066, #23406, .T. ) ;
#18984=DIRECTION ( 'NONE',  ( 0.000000000000000000, 1.000000000000000000, -6.123233995736766036E-17 ) ) ;
#18986=VECTOR ( 'NONE', #30753, 1000.000000000000000 ) ;
#18987=ORIENTED_EDGE ( 'NONE', *, *, #32856, .F. ) ;
#18990=EDGE_LOOP ( 'NONE', ( #14186, #7912, #15931 ) ) ;
#18992=DIRECTION ( 'NONE',  ( -0.000000000000000000, 1.000000000000000000, -0.000000000000000000 ) ) ;
#18995=AXIS2_PLACEMENT_3D ( 'NONE', #18590, #18408, #29429 ) ;
#18997=CARTESIAN_POINT ( 'NONE',  ( -355.0000000000000000, -119.0000000000000000, 113.9999999999999858 ) ) ;
#18998=VERTEX_POINT ( 'NONE', #23584 ) ;
#19002=CARTESIAN_POINT ( 'NONE',  ( 15.99999999999998579, 144.9999999999999716, -162.9999999999999432 ) ) ;
#19005=CARTESIAN_POINT ( 'NONE',  ( 15.99999999999998579, -115.0000000000000000, 155.0000000000000000 ) ) ;
#19010=LINE ( 'NONE', #17538, #14076 ) ;
#19012=ORIENTED_EDGE ( 'NONE', *, *, #12983, .F. ) ;
#19014=CARTESIAN_POINT ( 'NONE',  ( -12.00000000000001066, 144.9999999999999716, -154.9999999999999716 ) ) ;
#19015=CARTESIAN_POINT ( 'NONE',  ( -12.00000000000001066, -28.99999999999999645, 154.9999999999999716 ) ) ;
#19017=DIRECTION ( 'NONE',  ( -1.292961597001347186E-16, 0.000000000000000000, 1.000000000000000000 ) ) ;
#19018=ORIENTED_EDGE ( 'NONE', *, *, #30814, .F. ) ;
#19019=EDGE_CURVE ( 'NONE', #13074, #1683, #25548, .T. ) ;
#19021=CYLINDRICAL_SURFACE ( 'NONE', #21770, 7.999999999999979572 ) ;
#19022=VERTEX_POINT ( 'NONE', #33739 ) ;
#19023=CIRCLE ( 'NONE', #8761, 2.000000000000001776 ) ;
#19028=EDGE_LOOP ( 'NONE', ( #10583, #22101, #26838, #24604, #260, #216, #12546, #13554 ) ) ;
#19030=CARTESIAN_POINT ( 'NONE',  ( -418.0000000000000000, -105.0000000000000142, -77.99999999999997158 ) ) ;
#19031=DIRECTION ( 'NONE',  ( -5.546364386991661285E-52, 0.000000000000000000, -1.000000000000000000 ) ) ;
#19034=VERTEX_POINT ( 'NONE', #31246 ) ;
#19037=CARTESIAN_POINT ( 'NONE',  ( -347.0000000000000000, -125.0000000000000284, 181.0000000000000000 ) ) ;
#19038=VERTEX_POINT ( 'NONE', #31589 ) ;
#19040=CARTESIAN_POINT ( 'NONE',  ( -15.99999999999998579, -137.0000000000000000, 174.9999999999999432 ) ) ;
#19046=EDGE_LOOP ( 'NONE', ( #928, #15093, #15346, #19426, #20909, #10819, #31014, #27876 ) ) ;
#19051=CARTESIAN_POINT ( 'NONE',  ( -410.0000000000000568, -105.0000000000000142, -174.9999999999999716 ) ) ;
#19053=ORIENTED_EDGE ( 'NONE', *, *, #16300, .T. ) ;
#19060=DIRECTION ( 'NONE',  ( 0.000000000000000000, 5.145227585319922065E-49, 1.000000000000000000 ) ) ;
#19063=DIRECTION ( 'NONE',  ( 0.000000000000000000, -1.000000000000000000, -5.053935297177146739E-49 ) ) ;
#19064=EDGE_CURVE ( 'NONE', #25899, #1486, #31082, .T. ) ;
#19066=VERTEX_POINT ( 'NONE', #4513 ) ;
#19069=LINE ( 'NONE', #29559, #3598 ) ;
#19071=AXIS2_PLACEMENT_3D ( 'NONE', #17486, #33297, #30634 ) ;
#19074=DIRECTION ( 'NONE',  ( 0.000000000000000000, 1.310824597558155437E-49, 1.000000000000000000 ) ) ;
#19076=CIRCLE ( 'NONE', #23606, 7.999999999999979572 ) ;
#19077=EDGE_CURVE ( 'NONE', #32120, #33261, #28407, .T. ) ;
#19078=CARTESIAN_POINT ( 'NONE',  ( -418.0000000000000000, 104.9999999999999858, -162.9999999999999716 ) ) ;
#19080=DIRECTION ( 'NONE',  ( -0.000000000000000000, 1.000000000000000000, -0.000000000000000000 ) ) ;
#19084=VERTEX_POINT ( 'NONE', #29455 ) ;
#19086=DIRECTION ( 'NONE',  ( 0.000000000000000000, -1.000000000000000000, -5.053935297177146739E-49 ) ) ;
#19088=VERTEX_POINT ( 'NONE', #7723 ) ;
#19091=CIRCLE ( 'NONE', #12839, 7.999999999999979572 ) ;
#19093=ORIENTED_EDGE ( 'NONE', *, *, #16852, .T. ) ;
#19095=DIRECTION ( 'NONE',  ( -1.000000000000000000, -0.000000000000000000, -0.000000000000000000 ) ) ;
#19096=CYLINDRICAL_SURFACE ( 'NONE', #13549, 7.999999999999979572 ) ;
#19097=AXIS2_PLACEMENT_3D ( 'NONE', #12359, #9668, #30859 ) ;
#19098=EDGE_CURVE ( 'NONE', #2489, #6590, #26596, .T. ) ;
#19099=DIRECTION ( 'NONE',  ( 0.000000000000000000, 0.000000000000000000, -1.000000000000000000 ) ) ;
#19103=CARTESIAN_POINT ( 'NONE',  ( -499.9999999999999432, -113.0000000000000000, -155.0000000000000000 ) ) ;
#19105=CARTESIAN_POINT ( 'NONE',  ( -418.0000000000000000, -141.0000000000000000, -155.0000000000000000 ) ) ;
#19106=EDGE_CURVE ( 'NONE', #14881, #12542, #25344, .T. ) ;
#19108=CARTESIAN_POINT ( 'NONE',  ( -418.0000000000000000, 105.0000000000000142, 190.9999999999999716 ) ) ;
#19109=LINE ( 'NONE', #2877, #26331 ) ;
#19110=EDGE_CURVE ( 'NONE', #32967, #1944, #18610, .T. ) ;
#19120=CARTESIAN_POINT ( 'NONE',  ( -499.9999999999999432, 144.9999999999999716, -162.9999999999999716 ) ) ;
#19122=AXIS2_PLACEMENT_3D ( 'NONE', #18956, #32631, #74 ) ;
#19123=VERTEX_POINT ( 'NONE', #13264 ) ;
#19128=ORIENTED_EDGE ( 'NONE', *, *, #10044, .F. ) ;
#19131=VECTOR ( 'NONE', #13108, 1000.000000000000000 ) ;
#19133=DIRECTION ( 'NONE',  ( -3.040835319149746090E-31, -1.000000000000000000, 3.748118910144520367E-63 ) ) ;
#19134=DIRECTION ( 'NONE',  ( -1.000000000000000000, 0.000000000000000000, 0.000000000000000000 ) ) ;
#19141=PLANE ( 'NONE',  #30167 ) ;
#19144=CARTESIAN_POINT ( 'NONE',  ( -12.00000000000001066, -28.99999999999999645, -154.9999999999999716 ) ) ;
#19146=VERTEX_POINT ( 'NONE', #32453 ) ;
#19150=DIRECTION ( 'NONE',  ( 0.000000000000000000, 2.465190328815661892E-32, 1.000000000000000000 ) ) ;
#19152=EDGE_LOOP ( 'NONE', ( #24770, #31285, #31135, #4765 ) ) ;
#19154=EDGE_CURVE ( 'NONE', #32312, #9482, #359, .T. ) ;
#19159=AXIS2_PLACEMENT_3D ( 'NONE', #17199, #17026, #8989 ) ;
#19163=CIRCLE ( 'NONE', #35064, 3.999999999999976019 ) ;
#19172=LINE ( 'NONE', #25364, #18429 ) ;
#19175=CARTESIAN_POINT ( 'NONE',  ( -449.9999999999999432, 105.0000000000000142, 187.0000000000000000 ) ) ;
#19178=CARTESIAN_POINT ( 'NONE',  ( -499.9999999999999432, 136.9999999999999432, -162.9999999999999716 ) ) ;
#19179=VERTEX_POINT ( 'NONE', #21263 ) ;
#19180=ORIENTED_EDGE ( 'NONE', *, *, #20522, .T. ) ;
#19181=DIRECTION ( 'NONE',  ( 0.000000000000000000, 0.000000000000000000, -1.000000000000000000 ) ) ;
#19182=DIRECTION ( 'NONE',  ( 0.000000000000000000, 1.310824597558155437E-49, 1.000000000000000000 ) ) ;
#19184=EDGE_CURVE ( 'NONE', #15995, #17865, #10593, .T. ) ;
#19187=CARTESIAN_POINT ( 'NONE',  ( 11.99999999999999645, 124.9999999999999716, 155.0000000000000000 ) ) ;
#19195=VECTOR ( 'NONE', #12490, 1000.000000000000000 ) ;
#19197=FACE_OUTER_BOUND ( 'NONE', #15912, .T. ) ;
#19198=VERTEX_POINT ( 'NONE', #32283 ) ;
#19200=CARTESIAN_POINT ( 'NONE',  ( -20.00000000000004619, -134.9999999999999716, -162.9999999999999432 ) ) ;
#19201=VECTOR ( 'NONE', #18827, 1000.000000000000000 ) ;
#19203=PLANE ( 'NONE',  #34201 ) ;
#19204=CARTESIAN_POINT ( 'NONE',  ( 11.99999999999999645, -145.0000000000000000, 174.9999999999999432 ) ) ;
#19205=DIRECTION ( 'NONE',  ( -1.000000000000000000, 0.000000000000000000, -5.546364386991661285E-52 ) ) ;
#19206=ORIENTED_EDGE ( 'NONE', *, *, #31412, .T. ) ;
#19207=VERTEX_POINT ( 'NONE', #13087 ) ;
#19208=VECTOR ( 'NONE', #31420, 1000.000000000000000 ) ;
#19210=DIRECTION ( 'NONE',  ( 1.000000000000000000, 0.000000000000000000, -1.232595164407831220E-32 ) ) ;
#19214=CARTESIAN_POINT ( 'NONE',  ( -361.0000000000000000, -125.0000000000000284, 126.0000000000000000 ) ) ;
#19218=CARTESIAN_POINT ( 'NONE',  ( 15.99999999999998579, -145.0000000000000000, -186.9999999999999716 ) ) ;
#19219=ORIENTED_EDGE ( 'NONE', *, *, #25395, .F. ) ;
#19222=ORIENTED_EDGE ( 'NONE', *, *, #26086, .F. ) ;
#19223=LINE ( 'NONE', #11020, #32302 ) ;
#19226=CARTESIAN_POINT ( 'NONE',  ( -355.0000000000000000, 118.9999999999999716, 113.9999999999999858 ) ) ;
#19228=ORIENTED_EDGE ( 'NONE', *, *, #23910, .T. ) ;
#19233=ORIENTED_EDGE ( 'NONE', *, *, #15929, .F. ) ;
#19234=VERTEX_POINT ( 'NONE', #8967 ) ;
#19245=LINE ( 'NONE', #19415, #28492 ) ;
#19247=DIRECTION ( 'NONE',  ( 1.848892746611746419E-32, 6.842277657836020854E-49, -1.000000000000000000 ) ) ;
#19250=DIRECTION ( 'NONE',  ( -1.000000000000000000, -0.000000000000000000, -0.000000000000000000 ) ) ;
#19253=ORIENTED_EDGE ( 'NONE', *, *, #30385, .F. ) ;
#19256=EDGE_CURVE ( 'NONE', #30159, #32496, #33164, .T. ) ;
#19259=LINE ( 'NONE', #30454, #9116 ) ;
#19262=CARTESIAN_POINT ( 'NONE',  ( -347.0000000000000000, -125.0000000000000284, 181.0000000000000000 ) ) ;
#19263=CARTESIAN_POINT ( 'NONE',  ( -449.9999999999999432, 137.0000000000000000, 154.9999999999999716 ) ) ;
#19265=VECTOR ( 'NONE', #10446, 1000.000000000000000 ) ;
#19266=DIRECTION ( 'NONE',  ( 0.000000000000000000, 0.000000000000000000, 1.000000000000000000 ) ) ;
#19269=ORIENTED_EDGE ( 'NONE', *, *, #16373, .F. ) ;
#19276=VECTOR ( 'NONE', #5101, 1000.000000000000000 ) ;
#19278=PLANE ( 'NONE',  #31059 ) ;
#19281=DIRECTION ( 'NONE',  ( 0.000000000000000000, 0.000000000000000000, 1.000000000000000000 ) ) ;
#19284=VECTOR ( 'NONE', #7988, 1000.000000000000000 ) ;
#19286=ORIENTED_EDGE ( 'NONE', *, *, #25749, .T. ) ;
#19287=CARTESIAN_POINT ( 'NONE',  ( 11.99999999999999645, 108.9999999999999858, -175.0000000000000284 ) ) ;
#19288=CARTESIAN_POINT ( 'NONE',  ( -355.0000000000000000, -135.0000000000000000, 109.9999999999999858 ) ) ;
#19294=AXIS2_PLACEMENT_3D ( 'NONE', #8087, #21976, #29463 ) ;
#19297=VERTEX_POINT ( 'NONE', #21967 ) ;
#19298=ORIENTED_EDGE ( 'NONE', *, *, #18219, .T. ) ;
#19300=DIRECTION ( 'NONE',  ( 0.000000000000000000, 1.224646799147353207E-16, -1.000000000000000000 ) ) ;
#19301=CIRCLE ( 'NONE', #20446, 7.999999999999979572 ) ;
#19302=LINE ( 'NONE', #2733, #16957 ) ;
#19303=CARTESIAN_POINT ( 'NONE',  ( -361.0000000000000000, 134.9999999999999716, 126.0000000000000000 ) ) ;
#19305=EDGE_CURVE ( 'NONE', #2690, #22142, #22498, .T. ) ;
#19307=DIRECTION ( 'NONE',  ( 0.000000000000000000, -3.374343856708137958E-53, 1.000000000000000000 ) ) ;
#19308=DIRECTION ( 'NONE',  ( 0.000000000000000000, 1.310824597558155437E-49, 1.000000000000000000 ) ) ;
#19311=CYLINDRICAL_SURFACE ( 'NONE', #8571, 7.999999999999979572 ) ;
#19312=EDGE_LOOP ( 'NONE', ( #28501, #19907, #15237, #33976 ) ) ;
#19313=EDGE_CURVE ( 'NONE', #26108, #10330, #14321, .T. ) ;
#19314=LINE ( 'NONE', #3095, #20786 ) ;
#19318=DIRECTION ( 'NONE',  ( 0.000000000000000000, 0.000000000000000000, -1.000000000000000000 ) ) ;
#19320=CIRCLE ( 'NONE', #558, 4.750000000000004441 ) ;
#19321=DIRECTION ( 'NONE',  ( 0.000000000000000000, 2.309213040847544338E-50, 1.000000000000000000 ) ) ;
#19322=ORIENTED_EDGE ( 'NONE', *, *, #17590, .T. ) ;
#19323=DIRECTION ( 'NONE',  ( 0.000000000000000000, 2.309213040847544338E-50, 1.000000000000000000 ) ) ;
#19331=CYLINDRICAL_SURFACE ( 'NONE', #16032, 3.999999999999982681 ) ;
#19335=CARTESIAN_POINT ( 'NONE',  ( -20.00000000000007461, 136.9999999999999432, -159.0000000000000000 ) ) ;
#19336=CARTESIAN_POINT ( 'NONE',  ( -20.00000000000007461, 104.9999999999999858, -187.0000000000000000 ) ) ;
#19338=VERTEX_POINT ( 'NONE', #6103 ) ;
#19339=FACE_OUTER_BOUND ( 'NONE', #32665, .T. ) ;
#19344=CARTESIAN_POINT ( 'NONE',  ( -442.0000000000000000, 105.0000000000000000, 132.0000000000000000 ) ) ;
#19347=ADVANCED_FACE ( 'NONE', ( #17002, #779 ), #11648, .T. ) ;
#19352=CARTESIAN_POINT ( 'NONE',  ( -349.0000000000000000, -135.0000000000000000, 126.0000000000000000 ) ) ;
#19353=LINE ( 'NONE', #3316, #25894 ) ;
#19354=FACE_OUTER_BOUND ( 'NONE', #14178, .T. ) ;
#19359=ADVANCED_FACE ( 'NONE', ( #599 ), #16467, .F. ) ;
#19367=VECTOR ( 'NONE', #31971, 1000.000000000000000 ) ;
#19369=EDGE_CURVE ( 'NONE', #15358, #17291, #31546, .T. ) ;
#19371=DIRECTION ( 'NONE',  ( 1.848892746611746419E-32, 6.842277657836020854E-49, -1.000000000000000000 ) ) ;
#19372=CARTESIAN_POINT ( 'NONE',  ( -418.0000000000000000, -105.0000000000000142, -105.9999999999999574 ) ) ;
#19373=CARTESIAN_POINT ( 'NONE',  ( -12.00000000000001066, -109.0000000000000142, -155.0000000000000284 ) ) ;
#19375=EDGE_LOOP ( 'NONE', ( #7479, #28932, #5943, #9785 ) ) ;
#19381=DIRECTION ( 'NONE',  ( 0.000000000000000000, -0.000000000000000000, 1.000000000000000000 ) ) ;
#19383=DIRECTION ( 'NONE',  ( -3.040835319149746090E-31, -1.000000000000000000, 0.000000000000000000 ) ) ;
#19387=ORIENTED_EDGE ( 'NONE', *, *, #26521, .F. ) ;
#19389=ORIENTED_EDGE ( 'NONE', *, *, #5835, .F. ) ;
#19391=CIRCLE ( 'NONE', #1743, 3.999999999999976019 ) ;
#19393=DIRECTION ( 'NONE',  ( 0.000000000000000000, 0.000000000000000000, -1.000000000000000000 ) ) ;
#19394=AXIS2_PLACEMENT_3D ( 'NONE', #17919, #4346, #15403 ) ;
#19395=CARTESIAN_POINT ( 'NONE',  ( -15.99999999999998579, 4.559999999999908127, 172.9900000000000091 ) ) ;
#19399=ORIENTED_EDGE ( 'NONE', *, *, #10175, .F. ) ;
#19401=DIRECTION ( 'NONE',  ( -0.000000000000000000, 1.000000000000000000, -0.000000000000000000 ) ) ;
#19403=ORIENTED_EDGE ( 'NONE', *, *, #28692, .F. ) ;
#19408=ORIENTED_EDGE ( 'NONE', *, *, #18772, .F. ) ;
#19412=EDGE_CURVE ( 'NONE', #30341, #3104, #32153, .T. ) ;
#19413=DIRECTION ( 'NONE',  ( 0.000000000000000000, 0.000000000000000000, -1.000000000000000000 ) ) ;
#19414=EDGE_CURVE ( 'NONE', #19338, #29324, #12305, .T. ) ;
#19415=CARTESIAN_POINT ( 'NONE',  ( -12.00000000000001066, -124.9999999999999432, -154.9999999999999716 ) ) ;
#19417=VECTOR ( 'NONE', #6810, 1000.000000000000000 ) ;
#19420=VECTOR ( 'NONE', #16999, 1000.000000000000000 ) ;
#19426=ORIENTED_EDGE ( 'NONE', *, *, #14879, .F. ) ;
#19432=VECTOR ( 'NONE', #15222, 1000.000000000000000 ) ;
#19433=AXIS2_PLACEMENT_3D ( 'NONE', #931, #11801, #33662 ) ;
#19440=CARTESIAN_POINT ( 'NONE',  ( 12.00000000000003908, -115.0000000000000000, -158.9999999999999716 ) ) ;
#19443=CARTESIAN_POINT ( 'NONE',  ( 15.99999999999997868, -137.0000000000000000, 155.0000000000000000 ) ) ;
#19446=VECTOR ( 'NONE', #26293, 1000.000000000000000 ) ;
#19450=EDGE_LOOP ( 'NONE', ( #31579, #31869, #11450, #29078, #33870, #16432 ) ) ;
#19453=CARTESIAN_POINT ( 'NONE',  ( -449.9999999999999432, 113.0000000000000000, -175.0000000000000000 ) ) ;
#19455=EDGE_CURVE ( 'NONE', #26862, #11246, #1819, .T. ) ;
#19456=CIRCLE ( 'NONE', #20014, 7.999999999999979572 ) ;
#19459=ADVANCED_FACE ( 'NONE', ( #26032 ), #9661, .T. ) ;
#19461=LINE ( 'NONE', #14115, #26931 ) ;
#19462=ORIENTED_EDGE ( 'NONE', *, *, #30508, .F. ) ;
#19463=CYLINDRICAL_SURFACE ( 'NONE', #20168, 7.999999999999979572 ) ;
#19464=CIRCLE ( 'NONE', #8641, 3.999999999999976019 ) ;
#19469=CARTESIAN_POINT ( 'NONE',  ( 11.99999999999999645, -145.0000000000000000, -194.9999999999999432 ) ) ;
#19471=ORIENTED_EDGE ( 'NONE', *, *, #4540, .F. ) ;
#19475=ORIENTED_EDGE ( 'NONE', *, *, #18020, .T. ) ;
#19476=CARTESIAN_POINT ( 'NONE',  ( 11.99999999999999645, 136.9999999999999716, -155.0000000000000000 ) ) ;
#19478=CARTESIAN_POINT ( 'NONE',  ( -499.9999999999999432, -105.0000000000000142, -187.0000000000000000 ) ) ;
#19479=ORIENTED_EDGE ( 'NONE', *, *, #25230, .T. ) ;
#19489=DIRECTION ( 'NONE',  ( 1.000000000000000000, -0.000000000000000000, -0.000000000000000000 ) ) ;
#19490=ORIENTED_EDGE ( 'NONE', *, *, #13663, .T. ) ;
#19495=PLANE ( 'NONE',  #4696 ) ;
#19497=ORIENTED_EDGE ( 'NONE', *, *, #29083, .T. ) ;
#19499=EDGE_CURVE ( 'NONE', #9157, #28176, #10573, .T. ) ;
#19500=CARTESIAN_POINT ( 'NONE',  ( -499.9999999999999432, 136.9999999999999432, -194.9999999999999716 ) ) ;
#19504=CARTESIAN_POINT ( 'NONE',  ( -442.0000000000000000, 137.0000000000000000, -175.0000000000000000 ) ) ;
#19506=VECTOR ( 'NONE', #9600, 1000.000000000000000 ) ;
#19507=ORIENTED_EDGE ( 'NONE', *, *, #9275, .F. ) ;
#19508=VECTOR ( 'NONE', #13199, 1000.000000000000000 ) ;
#19510=DIRECTION ( 'NONE',  ( -1.000000000000000000, 0.000000000000000000, 0.000000000000000000 ) ) ;
#19513=ORIENTED_EDGE ( 'NONE', *, *, #34641, .F. ) ;
#19520=DIRECTION ( 'NONE',  ( 2.891205793294675368E-16, 7.888609052210118054E-31, 1.000000000000000000 ) ) ;
#19522=DIRECTION ( 'NONE',  ( 0.000000000000000000, -0.000000000000000000, 1.000000000000000000 ) ) ;
#19528=LINE ( 'NONE', #3135, #10655 ) ;
#19529=DIRECTION ( 'NONE',  ( 0.000000000000000000, -1.000000000000000000, 6.123233995736766036E-17 ) ) ;
#19535=EDGE_LOOP ( 'NONE', ( #1735, #17641, #13435, #22692 ) ) ;
#19538=EDGE_CURVE ( 'NONE', #3093, #16221, #2629, .T. ) ;
#19539=CARTESIAN_POINT ( 'NONE',  ( -500.0000000000000000, -113.0000000000000000, 194.9999999999999716 ) ) ;
#19541=CARTESIAN_POINT ( 'NONE',  ( -418.0000000000000000, -112.9999999999999858, -174.9999999999999716 ) ) ;
#19544=LINE ( 'NONE', #11531, #29271 ) ;
#19545=DIRECTION ( 'NONE',  ( 1.000000000000000000, 3.040835319149746528E-31, 1.232595164407830946E-32 ) ) ;
#19549=EDGE_CURVE ( 'NONE', #8592, #32250, #7679, .T. ) ;
#19551=FACE_OUTER_BOUND ( 'NONE', #20315, .T. ) ;
#19552=PLANE ( 'NONE',  #11494 ) ;
#19553=ORIENTED_EDGE ( 'NONE', *, *, #8934, .F. ) ;
#19560=EDGE_CURVE ( 'NONE', #15708, #21709, #7168, .T. ) ;
#19563=DIRECTION ( 'NONE',  ( 0.000000000000000000, -1.224646799147353207E-16, 1.000000000000000000 ) ) ;
#19565=VERTEX_POINT ( 'NONE', #15538 ) ;
#19566=VERTEX_POINT ( 'NONE', #21575 ) ;
#19567=CARTESIAN_POINT ( 'NONE',  ( -345.0000000000000000, -135.0000000000000000, 126.0000000000000000 ) ) ;
#19568=CARTESIAN_POINT ( 'NONE',  ( -430.0000000000000000, -114.9999999999999858, 126.0000000000000000 ) ) ;
#19570=CIRCLE ( 'NONE', #30350, 7.999999999999979572 ) ;
#19572=EDGE_CURVE ( 'NONE', #28310, #21537, #27082, .T. ) ;
#19575=LINE ( 'NONE', #6019, #16322 ) ;
#19576=ORIENTED_EDGE ( 'NONE', *, *, #31183, .F. ) ;
#19577=VECTOR ( 'NONE', #18348, 1000.000000000000000 ) ;
#19578=FACE_OUTER_BOUND ( 'NONE', #11659, .T. ) ;
#19579=FACE_OUTER_BOUND ( 'NONE', #14175, .T. ) ;
#19581=ADVANCED_FACE ( 'NONE', ( #29783 ), #32437, .F. ) ;
#19582=VERTEX_POINT ( 'NONE', #23536 ) ;
#19586=CARTESIAN_POINT ( 'NONE',  ( -12.00000000000001066, -32.99999999999997158, -175.0000000000000000 ) ) ;
#19587=ORIENTED_EDGE ( 'NONE', *, *, #16683, .T. ) ;
#19591=CARTESIAN_POINT ( 'NONE',  ( 11.99999999999999645, -115.0000000000000000, 162.9999999999999716 ) ) ;
#19592=DIRECTION ( 'NONE',  ( -1.000000000000000000, -3.469446951953834515E-18, 0.000000000000000000 ) ) ;
#19593=ADVANCED_FACE ( 'NONE', ( #29756 ), #34397, .F. ) ;
#19595=DIRECTION ( 'NONE',  ( -0.000000000000000000, -0.000000000000000000, -1.000000000000000000 ) ) ;
#19597=DIRECTION ( 'NONE',  ( -1.000000000000000000, 0.000000000000000000, -0.000000000000000000 ) ) ;
#19598=AXIS2_PLACEMENT_3D ( 'NONE', #27286, #27643, #3258 ) ;
#19604=EDGE_CURVE ( 'NONE', #30730, #1893, #10549, .T. ) ;
#19616=ADVANCED_FACE ( 'NONE', ( #10726 ), #18393, .T. ) ;
#19627=DIRECTION ( 'NONE',  ( -1.000000000000000000, 0.000000000000000000, 1.848892746611746966E-32 ) ) ;
#19630=VERTEX_POINT ( 'NONE', #22277 ) ;
#19631=AXIS2_PLACEMENT_3D ( 'NONE', #32118, #31767, #8086 ) ;
#19633=CARTESIAN_POINT ( 'NONE',  ( 12.00000000000001066, -109.0000000000000142, 155.0000000000000000 ) ) ;
#19637=DIRECTION ( 'NONE',  ( 1.000000000000000000, 0.000000000000000000, 0.000000000000000000 ) ) ;
#19648=AXIS2_PLACEMENT_3D ( 'NONE', #20403, #9368, #1693 ) ;
#19652=ORIENTED_EDGE ( 'NONE', *, *, #4662, .F. ) ;
#19659=CARTESIAN_POINT ( 'NONE',  ( -418.0000000000000000, 105.0000000000000142, 162.9999999999999716 ) ) ;
#19661=ORIENTED_EDGE ( 'NONE', *, *, #1413, .F. ) ;
#19662=ORIENTED_EDGE ( 'NONE', *, *, #34113, .F. ) ;
#19667=FACE_OUTER_BOUND ( 'NONE', #13364, .T. ) ;
#19668=DIRECTION ( 'NONE',  ( 0.000000000000000000, 1.000000000000000000, 0.000000000000000000 ) ) ;
#19672=ORIENTED_EDGE ( 'NONE', *, *, #23283, .T. ) ;
#19675=CARTESIAN_POINT ( 'NONE',  ( -499.9999999999999432, 140.9999999999999716, 187.0000000000000000 ) ) ;
#19676=DIRECTION ( 'NONE',  ( 0.000000000000000000, 1.000000000000000000, 5.053935297177146739E-49 ) ) ;
#19683=ORIENTED_EDGE ( 'NONE', *, *, #34646, .F. ) ;
#19685=( NAMED_UNIT ( * ) SI_UNIT ( $, .STERADIAN. ) SOLID_ANGLE_UNIT ( ) );
#19687=CIRCLE ( 'NONE', #13430, 3.999999999999976019 ) ;
#19689=AXIS2_PLACEMENT_3D ( 'NONE', #28044, #28402, #9538 ) ;
#19692=ORIENTED_EDGE ( 'NONE', *, *, #22059, .F. ) ;
#19693=VERTEX_POINT ( 'NONE', #8919 ) ;
#19694=DIRECTION ( 'NONE',  ( 0.000000000000000000, 0.000000000000000000, -1.000000000000000000 ) ) ;
#19700=LINE ( 'NONE', #8646, #6868 ) ;
#19701=ORIENTED_EDGE ( 'NONE', *, *, #17131, .T. ) ;
#19704=LINE ( 'NONE', #3311, #3315 ) ;
#19707=VECTOR ( 'NONE', #6155, 1000.000000000000000 ) ;
#19710=CARTESIAN_POINT ( 'NONE',  ( -418.0000000000000000, -105.0000000000000142, 132.0000000000000000 ) ) ;
#19711=DIRECTION ( 'NONE',  ( 0.000000000000000000, -3.374343856708137958E-53, 1.000000000000000000 ) ) ;
#19713=CIRCLE ( 'NONE', #33338, 7.999999999999979572 ) ;
#19715=CARTESIAN_POINT ( 'NONE',  ( -500.0000000000000000, -141.0000000000000000, 162.9999999999999716 ) ) ;
#19719=ORIENTED_EDGE ( 'NONE', *, *, #33499, .F. ) ;
#19720=DIRECTION ( 'NONE',  ( -0.000000000000000000, 1.000000000000000000, -0.000000000000000000 ) ) ;
#19721=DIRECTION ( 'NONE',  ( 1.000000000000000000, 0.000000000000000000, 0.000000000000000000 ) ) ;
#19722=VECTOR ( 'NONE', #23166, 1000.000000000000000 ) ;
#19726=CARTESIAN_POINT ( 'NONE',  ( -500.0000000000000000, -137.0000000000000000, 155.0000000000000000 ) ) ;
#19728=ORIENTED_EDGE ( 'NONE', *, *, #32844, .T. ) ;
#19736=CARTESIAN_POINT ( 'NONE',  ( -347.0000000000000000, -125.0000000000000284, 126.0000000000000000 ) ) ;
#19738=ORIENTED_EDGE ( 'NONE', *, *, #22711, .T. ) ;
#19740=ORIENTED_EDGE ( 'NONE', *, *, #19184, .T. ) ;
#19743=LINE ( 'NONE', #9226, #3319 ) ;
#19744=VECTOR ( 'NONE', #20925, 1000.000000000000000 ) ;
#19745=EDGE_CURVE ( 'NONE', #29922, #1812, #29, .T. ) ;
#19746=CARTESIAN_POINT ( 'NONE',  ( -499.9999999999999432, -105.0000000000000142, -162.9999999999999716 ) ) ;
#19748=AXIS2_PLACEMENT_3D ( 'NONE', #4094, #6601, #19973 ) ;
#19749=LINE ( 'NONE', #3180, #24120 ) ;
#19750=DIRECTION ( 'NONE',  ( 1.000000000000000000, 0.000000000000000000, 0.000000000000000000 ) ) ;
#19752=EDGE_LOOP ( 'NONE', ( #2075, #9709, #28593, #4176 ) ) ;
#19756=LINE ( 'NONE', #25245, #5021 ) ;
#19760=CIRCLE ( 'NONE', #4378, 4.000000000000003553 ) ;
#19763=VERTEX_POINT ( 'NONE', #32589 ) ;
#19764=DIRECTION ( 'NONE',  ( 0.000000000000000000, -1.000000000000000000, 0.000000000000000000 ) ) ;
#19766=DIRECTION ( 'NONE',  ( 0.000000000000000000, 0.000000000000000000, 1.000000000000000000 ) ) ;
#19768=CIRCLE ( 'NONE', #33203, 4.000000000000003553 ) ;
#19771=CARTESIAN_POINT ( 'NONE',  ( -410.0000000000000568, 113.0000000000000000, -175.0000000000000000 ) ) ;
#19772=EDGE_LOOP ( 'NONE', ( #18768, #20918, #32881, #21060 ) ) ;
#19773=VECTOR ( 'NONE', #15915, 1000.000000000000000 ) ;
#19774=AXIS2_PLACEMENT_3D ( 'NONE', #6031, #10864, #22248 ) ;
#19781=CARTESIAN_POINT ( 'NONE',  ( -442.0000000000000000, 104.9999999999999858, -155.0000000000000000 ) ) ;
#19786=EDGE_CURVE ( 'NONE', #17680, #12453, #16960, .T. ) ;
#19788=CARTESIAN_POINT ( 'NONE',  ( -12.00000000000001066, -28.99999999999999645, -154.9999999999999716 ) ) ;
#19789=CARTESIAN_POINT ( 'NONE',  ( -418.0000000000000000, 141.0000000000000000, -175.0000000000000000 ) ) ;
#19797=CARTESIAN_POINT ( 'NONE',  ( -414.0000000000000568, 105.0000000000000142, 162.9999999999999716 ) ) ;
#19798=FACE_OUTER_BOUND ( 'NONE', #3378, .T. ) ;
#19799=EDGE_LOOP ( 'NONE', ( #3817, #1044, #12392, #5575 ) ) ;
#19802=AXIS2_PLACEMENT_3D ( 'NONE', #23150, #20816, #15314 ) ;
#19803=DIRECTION ( 'NONE',  ( 0.000000000000000000, 0.000000000000000000, -1.000000000000000000 ) ) ;
#19806=DIRECTION ( 'NONE',  ( 1.000000000000000000, 0.000000000000000000, 1.300283923313630633E-47 ) ) ;
#19808=EDGE_CURVE ( 'NONE', #34124, #32414, #21923, .T. ) ;
#19811=DIRECTION ( 'NONE',  ( 0.000000000000000000, -1.000000000000000000, -0.000000000000000000 ) ) ;
#19813=DIRECTION ( 'NONE',  ( 0.000000000000000000, 1.310824597558155437E-49, 1.000000000000000000 ) ) ;
#19815=DIRECTION ( 'NONE',  ( -1.000000000000000000, 0.000000000000000000, 0.000000000000000000 ) ) ;
#19818=EDGE_CURVE ( 'NONE', #30600, #24075, #23132, .T. ) ;
#19819=AXIS2_PLACEMENT_3D ( 'NONE', #10316, #21176, #12831 ) ;
#19825=AXIS2_PLACEMENT_3D ( 'NONE', #34119, #31625, #1210 ) ;
#19826=ORIENTED_EDGE ( 'NONE', *, *, #9797, .T. ) ;
#19829=ORIENTED_EDGE ( 'NONE', *, *, #5193, .T. ) ;
#19830=DIRECTION ( 'NONE',  ( -1.000000000000000000, 0.000000000000000000, 0.000000000000000000 ) ) ;
#19833=ORIENTED_EDGE ( 'NONE', *, *, #28653, .F. ) ;
#19834=CARTESIAN_POINT ( 'NONE',  ( -15.99999999999998579, 75.55999999999990280, 172.9900000000000091 ) ) ;
#19835=CARTESIAN_POINT ( 'NONE',  ( -445.9999999999999432, 137.0000000000000000, -155.0000000000000000 ) ) ;
#19836=EDGE_LOOP ( 'NONE', ( #31991, #23867, #2060, #13526 ) ) ;
#19843=DIRECTION ( 'NONE',  ( 0.000000000000000000, 1.000000000000000000, 1.310824597558155437E-49 ) ) ;
#19846=AXIS2_PLACEMENT_3D ( 'NONE', #9016, #30556, #27696 ) ;
#19848=EDGE_LOOP ( 'NONE', ( #23503, #19692, #4365, #2742, #3271, #11436, #11400, #9739 ) ) ;
#19857=DIRECTION ( 'NONE',  ( 1.000000000000000000, 0.000000000000000000, 0.000000000000000000 ) ) ;
#19858=CARTESIAN_POINT ( 'NONE',  ( -445.9999999999999432, -125.0000000000000000, -101.9999999999999858 ) ) ;
#19859=CARTESIAN_POINT ( 'NONE',  ( -361.0000000000000000, -125.0000000000000284, 130.0000000000000000 ) ) ;
#19861=EDGE_CURVE ( 'NONE', #11184, #6968, #1610, .T. ) ;
#19866=ORIENTED_EDGE ( 'NONE', *, *, #9937, .T. ) ;
#19868=VECTOR ( 'NONE', #34046, 1000.000000000000000 ) ;
#19872=VERTEX_POINT ( 'NONE', #9273 ) ;
#19873=ORIENTED_EDGE ( 'NONE', *, *, #3932, .T. ) ;
#19877=LINE ( 'NONE', #7017, #2623 ) ;
#19878=DIRECTION ( 'NONE',  ( 0.000000000000000000, 0.000000000000000000, 1.000000000000000000 ) ) ;
#19879=EDGE_LOOP ( 'NONE', ( #7852, #10615, #20314, #6544 ) ) ;
#19880=ORIENTED_EDGE ( 'NONE', *, *, #3696, .F. ) ;
#19883=CARTESIAN_POINT ( 'NONE',  ( -349.0000000000000000, 124.9999999999999432, 185.0000000000000000 ) ) ;
#19884=CARTESIAN_POINT ( 'NONE',  ( -12.00000000000001066, -137.0000000000000000, 155.0000000000000000 ) ) ;
#19885=CARTESIAN_POINT ( 'NONE',  ( -418.0000000000000000, 124.9999999999999574, -187.0000000000000000 ) ) ;
#19886=DIRECTION ( 'NONE',  ( 0.000000000000000000, 0.000000000000000000, -1.000000000000000000 ) ) ;
#19887=DIRECTION ( 'NONE',  ( 0.000000000000000000, 1.000000000000000000, 1.224646799147353207E-16 ) ) ;
#19890=DIRECTION ( 'NONE',  ( 1.000000000000000000, 3.040835319149746090E-31, 1.232595164407830946E-32 ) ) ;
#19895=CYLINDRICAL_SURFACE ( 'NONE', #25171, 7.999999999999979572 ) ;
#19897=DIRECTION ( 'NONE',  ( 0.000000000000000000, -1.000000000000000000, 6.123233995736766036E-17 ) ) ;
#19899=EDGE_CURVE ( 'NONE', #5382, #9264, #14027, .T. ) ;
#19903=DIRECTION ( 'NONE',  ( 5.546364386991661285E-52, 0.000000000000000000, 1.000000000000000000 ) ) ;
#19904=FACE_OUTER_BOUND ( 'NONE', #10267, .T. ) ;
#19907=ORIENTED_EDGE ( 'NONE', *, *, #10276, .F. ) ;
#19911=CARTESIAN_POINT ( 'NONE',  ( 19.99999999999996092, -134.9999999999999716, 162.9999999999999716 ) ) ;
#19912=CARTESIAN_POINT ( 'NONE',  ( -361.0000000000000000, -125.0000000000000284, 164.9999999999999716 ) ) ;
#19913=DIRECTION ( 'NONE',  ( -0.000000000000000000, 1.000000000000000000, -0.000000000000000000 ) ) ;
#19918=CARTESIAN_POINT ( 'NONE',  ( -449.9999999999999432, -125.0000000000000000, 107.9999999999999858 ) ) ;
#19922=ORIENTED_EDGE ( 'NONE', *, *, #22, .T. ) ;
#19925=VERTEX_POINT ( 'NONE', #30990 ) ;
#19926=PLANE ( 'NONE',  #18698 ) ;
#19930=ORIENTED_EDGE ( 'NONE', *, *, #25463, .T. ) ;
#19931=( NAMED_UNIT ( * ) SI_UNIT ( $, .STERADIAN. ) SOLID_ANGLE_UNIT ( ) );
#19932=EDGE_CURVE ( 'NONE', #11236, #31513, #8885, .T. ) ;
#19933=CARTESIAN_POINT ( 'NONE',  ( -20.00000000000007461, 144.9999999999999716, -162.9999999999999716 ) ) ;
#19936=EDGE_CURVE ( 'NONE', #904, #27132, #12311, .T. ) ;
#19941=CARTESIAN_POINT ( 'NONE',  ( -12.00000000000003908, -134.9999999999999716, -186.9999999999999716 ) ) ;
#19942=CARTESIAN_POINT ( 'NONE',  ( -442.0000000000000000, 105.0000000000000142, 187.0000000000000000 ) ) ;
#19943=ADVANCED_FACE ( 'NONE', ( #6767 ), #6937, .F. ) ;
#19944=VERTEX_POINT ( 'NONE', #23326 ) ;
#19945=ORIENTED_EDGE ( 'NONE', *, *, #16119, .F. ) ;
#19948=ORIENTED_EDGE ( 'NONE', *, *, #18471, .T. ) ;
#19949=ORIENTED_EDGE ( 'NONE', *, *, #4086, .F. ) ;
#19950=ADVANCED_FACE ( 'NONE', ( #34173 ), #25286, .T. ) ;
#19952=DIRECTION ( 'NONE',  ( 0.000000000000000000, 0.000000000000000000, -1.000000000000000000 ) ) ;
#19957=LINE ( 'NONE', #22099, #10499 ) ;
#19958=DIRECTION ( 'NONE',  ( 1.000000000000000000, 3.040835319149746090E-31, 1.232595164407830946E-32 ) ) ;
#19959=AXIS2_PLACEMENT_3D ( 'NONE', #10730, #10554, #24234 ) ;
#19962=CARTESIAN_POINT ( 'NONE',  ( -12.00000000000001066, -124.9999999999999432, -190.9999999999999432 ) ) ;
#19964=VECTOR ( 'NONE', #31948, 1000.000000000000000 ) ;
#19969=FACE_OUTER_BOUND ( 'NONE', #22772, .T. ) ;
#19971=ORIENTED_EDGE ( 'NONE', *, *, #8826, .F. ) ;
#19973=DIRECTION ( 'NONE',  ( 0.000000000000000000, 0.000000000000000000, -1.000000000000000000 ) ) ;
#19974=CARTESIAN_POINT ( 'NONE',  ( 19.99999999999998224, 134.9999999999999432, -186.9999999999999716 ) ) ;
#19981=VERTEX_POINT ( 'NONE', #18010 ) ;
#19982=DIRECTION ( 'NONE',  ( 0.000000000000000000, 0.000000000000000000, -1.000000000000000000 ) ) ;
#19984=EDGE_CURVE ( 'NONE', #8292, #18383, #3569, .T. ) ;
#19986=EDGE_CURVE ( 'NONE', #2032, #30341, #22636, .T. ) ;
#19987=VERTEX_POINT ( 'NONE', #17313 ) ;
#19992=VECTOR ( 'NONE', #14526, 1000.000000000000000 ) ;
#19993=AXIS2_PLACEMENT_3D ( 'NONE', #26349, #12665, #17840 ) ;
#19994=ORIENTED_EDGE ( 'NONE', *, *, #3557, .T. ) ;
#20000=EDGE_CURVE ( 'NONE', #14902, #13361, #34704, .T. ) ;
#20004=CARTESIAN_POINT ( 'NONE',  ( -363.0000000000000000, -125.0000000000000284, 114.0000000000000000 ) ) ;
#20008=CARTESIAN_POINT ( 'NONE',  ( -12.00000000000001066, 144.9999999999999716, -186.9999999999999716 ) ) ;
#20010=DIRECTION ( 'NONE',  ( -0.000000000000000000, 1.131431318426415506E-52, 1.000000000000000000 ) ) ;
#20013=ORIENTED_EDGE ( 'NONE', *, *, #30645, .T. ) ;
#20014=AXIS2_PLACEMENT_3D ( 'NONE', #23142, #25970, #30968 ) ;
#20015=EDGE_CURVE ( 'NONE', #21709, #15708, #14050, .T. ) ;
#20016=DIRECTION ( 'NONE',  ( -0.000000000000000000, 1.000000000000000000, -0.000000000000000000 ) ) ;
#20023=LINE ( 'NONE', #1147, #2578 ) ;
#20026=DIRECTION ( 'NONE',  ( 0.000000000000000000, 1.000000000000000000, 2.465190328815662439E-32 ) ) ;
#20028=CARTESIAN_POINT ( 'NONE',  ( -445.9999999999999432, -105.0000000000000142, 187.0000000000000000 ) ) ;
#20032=CARTESIAN_POINT ( 'NONE',  ( 19.99999999999998934, -137.0000000000000000, 155.0000000000000000 ) ) ;
#20037=CLOSED_SHELL ( 'NONE', ( #9084, #22386, #23184, #6852, #14439, #7391, #27632, #7837, #25016, #1499, #22603, #17239, #7683, #21123, #7694, #14789, #19347, #7957 ) ) ;
#20038=PLANE ( 'NONE',  #8025 ) ;
#20041=ORIENTED_EDGE ( 'NONE', *, *, #7540, .F. ) ;
#20042=AXIS2_PLACEMENT_3D ( 'NONE', #13420, #5725, #27105 ) ;
#20043=AXIS2_PLACEMENT_3D ( 'NONE', #10069, #31772, #7378 ) ;
#20050=DIRECTION ( 'NONE',  ( -0.000000000000000000, 1.000000000000000000, -0.000000000000000000 ) ) ;
#20051=CARTESIAN_POINT ( 'NONE',  ( -361.0000000000000000, -125.0000000000000284, 183.0000000000000000 ) ) ;
#20055=CARTESIAN_POINT ( 'NONE',  ( -449.9999999999999432, -125.0000000000000000, -101.9999999999999858 ) ) ;
#20057=LINE ( 'NONE', #11694, #34374 ) ;
#20058=LINE ( 'NONE', #25911, #34027 ) ;
#20059=CARTESIAN_POINT ( 'NONE',  ( -445.9999999999999432, -112.9999999999999858, -155.0000000000000000 ) ) ;
#20063=PLANE ( 'NONE',  #20962 ) ;
#20065=CARTESIAN_POINT ( 'NONE',  ( -500.0000000000000000, -137.0000000000000000, 187.0000000000000000 ) ) ;
#20067=DIRECTION ( 'NONE',  ( 1.000000000000000000, -0.000000000000000000, -0.000000000000000000 ) ) ;
#20069=LINE ( 'NONE', #6335, #21195 ) ;
#20073=AXIS2_PLACEMENT_3D ( 'NONE', #29990, #32821, #16480 ) ;
#20075=LINE ( 'NONE', #9560, #2435 ) ;
#20076=VERTEX_POINT ( 'NONE', #21001 ) ;
#20078=EDGE_LOOP ( 'NONE', ( #2281, #31328, #18859, #34738 ) ) ;
#20082=ORIENTED_EDGE ( 'NONE', *, *, #29812, .F. ) ;
#20090=CARTESIAN_POINT ( 'NONE',  ( 11.99999999999999645, -145.0000000000000000, -162.9999999999999432 ) ) ;
#20091=LINE ( 'NONE', #19736, #24463 ) ;
#20097=LINE ( 'NONE', #1571, #8596 ) ;
#20102=ORIENTED_EDGE ( 'NONE', *, *, #2444, .F. ) ;
#20105=ORIENTED_EDGE ( 'NONE', *, *, #4935, .F. ) ;
#20109=DIRECTION ( 'NONE',  ( -0.000000000000000000, 1.000000000000000000, -0.000000000000000000 ) ) ;
#20110=VECTOR ( 'NONE', #29058, 1000.000000000000000 ) ;
#20111=CARTESIAN_POINT ( 'NONE',  ( -12.00000000000001066, 112.9999999999999574, -155.0000000000000000 ) ) ;
#20112=ORIENTED_EDGE ( 'NONE', *, *, #901, .T. ) ;
#20113=CYLINDRICAL_SURFACE ( 'NONE', #6125, 3.999999999999976019 ) ;
#20114=DIRECTION ( 'NONE',  ( 0.000000000000000000, -1.000000000000000000, -1.224646799147353207E-16 ) ) ;
#20115=CARTESIAN_POINT ( 'NONE',  ( 15.99999999999998579, 4.559999999999908127, -177.7400000000000091 ) ) ;
#20117=CIRCLE ( 'NONE', #33749, 7.999999999999979572 ) ;
#20118=VECTOR ( 'NONE', #34905, 1000.000000000000000 ) ;
#20120=CARTESIAN_POINT ( 'NONE',  ( -19.99999999999998934, -124.9999999999999432, -186.9999999999999716 ) ) ;
#20126=DIRECTION ( 'NONE',  ( 1.000000000000000000, 3.469446951953834515E-18, 0.000000000000000000 ) ) ;
#20128=CARTESIAN_POINT ( 'NONE',  ( -12.00000000000001066, -105.0000000000000142, -154.9999999999999716 ) ) ;
#20130=VERTEX_POINT ( 'NONE', #32373 ) ;
#20131=CARTESIAN_POINT ( 'NONE',  ( -442.0000000000000000, 105.0000000000000142, 159.0000000000000000 ) ) ;
#20143=DIRECTION ( 'NONE',  ( 0.000000000000000000, 1.000000000000000000, 1.224646799147353207E-16 ) ) ;
#20145=CIRCLE ( 'NONE', #28114, 3.999999999999976019 ) ;
#20152=EDGE_LOOP ( 'NONE', ( #23819, #24217, #2416, #8190 ) ) ;
#20153=DIRECTION ( 'NONE',  ( 1.000000000000000000, 0.000000000000000000, -1.848892746611746966E-32 ) ) ;
#20162=DIRECTION ( 'NONE',  ( 0.000000000000000000, -1.000000000000000000, 6.123233995736766036E-17 ) ) ;
#20163=DIRECTION ( 'NONE',  ( -0.000000000000000000, 0.000000000000000000, 1.000000000000000000 ) ) ;
#20167=ORIENTED_EDGE ( 'NONE', *, *, #9962, .T. ) ;
#20168=AXIS2_PLACEMENT_3D ( 'NONE', #27101, #582, #14117 ) ;
#20171=LINE ( 'NONE', #22352, #5641 ) ;
#20177=VECTOR ( 'NONE', #7717, 1000.000000000000000 ) ;
#20179=DIRECTION ( 'NONE',  ( 0.000000000000000000, 0.000000000000000000, -1.000000000000000000 ) ) ;
#20183=DIRECTION ( 'NONE',  ( 1.000000000000000000, 0.000000000000000000, -1.232595164407831220E-32 ) ) ;
#20186=AXIS2_PLACEMENT_3D ( 'NONE', #9590, #20445, #20788 ) ;
#20187=EDGE_CURVE ( 'NONE', #17291, #33296, #10621, .T. ) ;
#20190=CARTESIAN_POINT ( 'NONE',  ( -15.99999999999998579, 112.9999999999999574, -155.0000000000000000 ) ) ;
#20192=CARTESIAN_POINT ( 'NONE',  ( -500.0000000000000000, -137.0000000000000000, 162.9999999999999716 ) ) ;
#20193=DIRECTION ( 'NONE',  ( 0.000000000000000000, 0.000000000000000000, -1.000000000000000000 ) ) ;
#20195=VECTOR ( 'NONE', #5988, 1000.000000000000000 ) ;
#20199=ORIENTED_EDGE ( 'NONE', *, *, #12489, .T. ) ;
#20200=CLOSED_SHELL ( 'NONE', ( #10820, #17983, #12351, #32607, #29074, #26488, #22015, #29358, #28356, #34976 ) ) ;
#20205=LINE ( 'NONE', #33360, #20643 ) ;
#20210=DIRECTION ( 'NONE',  ( -1.000000000000000000, 0.000000000000000000, 0.000000000000000000 ) ) ;
#20217=AXIS2_PLACEMENT_3D ( 'NONE', #26843, #29692, #16184 ) ;
#20218=VECTOR ( 'NONE', #9002, 1000.000000000000000 ) ;
#20220=DIRECTION ( 'NONE',  ( 0.000000000000000000, 1.000000000000000000, 5.053935297177146739E-49 ) ) ;
#20221=ORIENTED_EDGE ( 'NONE', *, *, #32146, .F. ) ;
#20226=AXIS2_PLACEMENT_3D ( 'NONE', #1687, #12915, #34614 ) ;
#20227=CARTESIAN_POINT ( 'NONE',  ( -414.0000000000000568, -105.0000000000000142, 162.9999999999999716 ) ) ;
#20229=ORIENTED_EDGE ( 'NONE', *, *, #28908, .F. ) ;
#20232=CARTESIAN_POINT ( 'NONE',  ( -500.0000000000000000, -141.0000000000000000, 162.9999999999999716 ) ) ;
#20234=CARTESIAN_POINT ( 'NONE',  ( -410.0000000000000568, 105.0000000000000142, 187.0000000000000000 ) ) ;
#20237=DIRECTION ( 'NONE',  ( 1.848892746611746966E-32, -6.842277657836020854E-49, 1.000000000000000000 ) ) ;
#20238=EDGE_CURVE ( 'NONE', #14266, #9246, #29392, .T. ) ;
#20239=ADVANCED_FACE ( 'NONE', ( #33263 ), #30072, .T. ) ;
#20241=ORIENTED_EDGE ( 'NONE', *, *, #18585, .F. ) ;
#20243=CYLINDRICAL_SURFACE ( 'NONE', #9412, 7.999999999999979572 ) ;
#20247=DIRECTION ( 'NONE',  ( 0.000000000000000000, 1.000000000000000000, 5.145227585319922065E-49 ) ) ;
#20248=ORIENTED_EDGE ( 'NONE', *, *, #2762, .F. ) ;
#20249=DIRECTION ( 'NONE',  ( 0.000000000000000000, 1.000000000000000000, 0.000000000000000000 ) ) ;
#20254=DIRECTION ( 'NONE',  ( 0.000000000000000000, -2.465190328815661892E-32, -1.000000000000000000 ) ) ;
#20256=EDGE_CURVE ( 'NONE', #2574, #25012, #11210, .T. ) ;
#20257=EDGE_LOOP ( 'NONE', ( #23629, #27646, #17965, #18946 ) ) ;
#20259=EDGE_CURVE ( 'NONE', #33397, #8951, #23151, .T. ) ;
#20263=EDGE_LOOP ( 'NONE', ( #4698, #22160, #33730, #34439 ) ) ;
#20265=CARTESIAN_POINT ( 'NONE',  ( 12.00000000000001066, -64.99999999999997158, -154.9999999999999716 ) ) ;
#20266=EDGE_CURVE ( 'NONE', #21471, #16703, #19575, .T. ) ;
#20269=DIRECTION ( 'NONE',  ( -1.000000000000000000, 0.000000000000000000, 1.232595164407831220E-32 ) ) ;
#20271=VERTEX_POINT ( 'NONE', #27570 ) ;
#20275=DIRECTION ( 'NONE',  ( -3.469446951953832974E-18, -1.000000000000000000, -7.888609052210116302E-31 ) ) ;
#20276=EDGE_CURVE ( 'NONE', #33086, #29943, #8525, .T. ) ;
#20277=FACE_OUTER_BOUND ( 'NONE', #26775, .T. ) ;
#20279=VERTEX_POINT ( 'NONE', #30236 ) ;
#20284=CYLINDRICAL_SURFACE ( 'NONE', #28819, 7.999999999999979572 ) ;
#20285=LINE ( 'NONE', #31474, #27998 ) ;
#20289=LINE ( 'NONE', #14429, #9212 ) ;
#20292=UNCERTAINTY_MEASURE_WITH_UNIT (LENGTH_MEASURE( 1.000000000000000082E-05 ), #22824, 'distance_accuracy_value', 'NONE');
#20293=DIRECTION ( 'NONE',  ( -2.736911063134582149E-48, 7.888609052210118054E-31, 1.000000000000000000 ) ) ;
#20296=CIRCLE ( 'NONE', #35055, 3.999999999999982681 ) ;
#20298=EDGE_CURVE ( 'NONE', #27718, #11639, #21998, .T. ) ;
#20299=EDGE_CURVE ( 'NONE', #34042, #34303, #11920, .T. ) ;
#20300=VERTEX_POINT ( 'NONE', #33437 ) ;
#20302=ORIENTED_EDGE ( 'NONE', *, *, #31682, .F. ) ;
#20303=VECTOR ( 'NONE', #30996, 1000.000000000000000 ) ;
#20304=CARTESIAN_POINT ( 'NONE',  ( -349.0000000000000000, 134.9999999999999716, 111.9999999999999858 ) ) ;
#20306=AXIS2_PLACEMENT_3D ( 'NONE', #5486, #24521, #24002 ) ;
#20309=ORIENTED_EDGE ( 'NONE', *, *, #28997, .F. ) ;
#20310=DIRECTION ( 'NONE',  ( 1.000000000000000000, 3.469446951953834515E-18, -2.736911063134582149E-48 ) ) ;
#20314=ORIENTED_EDGE ( 'NONE', *, *, #2520, .F. ) ;
#20315=EDGE_LOOP ( 'NONE', ( #17896, #30988, #33444, #32401 ) ) ;
#20316=CARTESIAN_POINT ( 'NONE',  ( -355.0000000000000000, -119.0000000000000000, 109.9999999999999858 ) ) ;
#20321=VECTOR ( 'NONE', #9545, 1000.000000000000000 ) ;
#20323=EDGE_CURVE ( 'NONE', #28711, #19987, #6894, .T. ) ;
#20330=CIRCLE ( 'NONE', #9528, 2.000000000000001776 ) ;
#20331=CARTESIAN_POINT ( 'NONE',  ( 11.99999999999999645, 104.9999999999999858, -175.0000000000000284 ) ) ;
#20333=ORIENTED_EDGE ( 'NONE', *, *, #27300, .F. ) ;
#20338=ADVANCED_FACE ( 'NONE', ( #15114 ), #14768, .T. ) ;
#20339=ADVANCED_FACE ( 'NONE', ( #20277 ), #9233, .T. ) ;
#20341=EDGE_CURVE ( 'NONE', #18803, #18049, #17622, .T. ) ;
#20348=DIRECTION ( 'NONE',  ( 0.000000000000000000, -1.131431318426415506E-52, -1.000000000000000000 ) ) ;
#20350=AXIS2_PLACEMENT_3D ( 'NONE', #29883, #24513, #16372 ) ;
#20351=AXIS2_PLACEMENT_3D ( 'NONE', #11223, #27228, #3013 ) ;
#20358=DIRECTION ( 'NONE',  ( -1.000000000000000000, -3.469446951953834515E-18, 0.000000000000000000 ) ) ;
#20359=DIRECTION ( 'NONE',  ( -1.000000000000000000, 0.000000000000000000, -5.546364386991661285E-52 ) ) ;
#20361=CARTESIAN_POINT ( 'NONE',  ( -20.00000000000007461, 144.9999999999999432, 162.9999999999999716 ) ) ;
#20364=STYLED_ITEM('',(#35254),#11835);
#20365=DIRECTION ( 'NONE',  ( 1.232595164407830946E-32, 3.421138828918010427E-49, -1.000000000000000000 ) ) ;
#20366=CYLINDRICAL_SURFACE ( 'NONE', #337, 7.999999999999979572 ) ;
#20367=CYLINDRICAL_SURFACE ( 'NONE', #34093, 4.000000000000003553 ) ;
#20368=EDGE_LOOP ( 'NONE', ( #4554, #32766, #31195, #12725 ) ) ;
#20373=CARTESIAN_POINT ( 'NONE',  ( -19.99999999999998934, 4.559999999999908127, -177.7400000000000091 ) ) ;
#20376=EDGE_CURVE ( 'NONE', #31329, #1812, #2105, .T. ) ;
#20384=ORIENTED_EDGE ( 'NONE', *, *, #9724, .F. ) ;
#20392=VERTEX_POINT ( 'NONE', #28449 ) ;
#20393=VERTEX_POINT ( 'NONE', #6557 ) ;
#20394=DIRECTION ( 'NONE',  ( 0.000000000000000000, 0.000000000000000000, 1.000000000000000000 ) ) ;
#20396=AXIS2_PLACEMENT_3D ( 'NONE', #14421, #22596, #3880 ) ;
#20399=DIRECTION ( 'NONE',  ( 0.000000000000000000, -1.000000000000000000, -2.465190328815662439E-32 ) ) ;
#20400=CARTESIAN_POINT ( 'NONE',  ( -442.0000000000000000, -145.0000000000000000, -155.0000000000000000 ) ) ;
#20402=ORIENTED_EDGE ( 'NONE', *, *, #33677, .T. ) ;
#20403=CARTESIAN_POINT ( 'NONE',  ( -347.0000000000000000, -125.0000000000000284, 126.0000000000000000 ) ) ;
#20405=CARTESIAN_POINT ( 'NONE',  ( -355.0000000000000000, 118.9999999999999716, 126.0000000000000000 ) ) ;
#20406=LINE ( 'NONE', #15070, #31213 ) ;
#20408=CIRCLE ( 'NONE', #7287, 7.999999999999979572 ) ;
#20409=FACE_OUTER_BOUND ( 'NONE', #2055, .T. ) ;
#20411=VERTEX_POINT ( 'NONE', #9420 ) ;
#20413=FACE_BOUND ( 'NONE', #16860, .T. ) ;
#20417=DIRECTION ( 'NONE',  ( 0.000000000000000000, 0.000000000000000000, 1.000000000000000000 ) ) ;
#20423=ORIENTED_EDGE ( 'NONE', *, *, #9086, .F. ) ;
#20424=LINE ( 'NONE', #33943, #31355 ) ;
#20429=ADVANCED_FACE ( 'NONE', ( #20448 ), #28797, .F. ) ;
#20430=EDGE_CURVE ( 'NONE', #17427, #143, #34131, .T. ) ;
#20433=ORIENTED_EDGE ( 'NONE', *, *, #28445, .T. ) ;
#20436=CYLINDRICAL_SURFACE ( 'NONE', #27197, 2.000000000000001776 ) ;
#20441=VERTEX_POINT ( 'NONE', #1911 ) ;
#20442=DIRECTION ( 'NONE',  ( 1.000000000000000000, 0.000000000000000000, 5.546364386991661285E-52 ) ) ;
#20444=DIRECTION ( 'NONE',  ( 0.000000000000000000, -5.053935297177146739E-49, -1.000000000000000000 ) ) ;
#20445=DIRECTION ( 'NONE',  ( -0.000000000000000000, 0.000000000000000000, 1.000000000000000000 ) ) ;
#20446=AXIS2_PLACEMENT_3D ( 'NONE', #12922, #22972, #7910 ) ;
#20447=CYLINDRICAL_SURFACE ( 'NONE', #33565, 3.999999999999976019 ) ;
#20448=FACE_OUTER_BOUND ( 'NONE', #6381, .T. ) ;
#20449=CYLINDRICAL_SURFACE ( 'NONE', #10159, 3.999999999999976019 ) ;
#20455=EDGE_CURVE ( 'NONE', #12627, #26996, #29147, .T. ) ;
#20458=CARTESIAN_POINT ( 'NONE',  ( -15.99999999999998579, 144.9999999999999716, -162.9999999999999432 ) ) ;
#20459=DIRECTION ( 'NONE',  ( 0.000000000000000000, -1.000000000000000000, -1.224646799147353207E-16 ) ) ;
#20463=DIRECTION ( 'NONE',  ( 1.000000000000000000, 0.000000000000000000, 0.000000000000000000 ) ) ;
#20465=ORIENTED_EDGE ( 'NONE', *, *, #15161, .F. ) ;
#20469=ORIENTED_EDGE ( 'NONE', *, *, #21309, .T. ) ;
#20474=EDGE_LOOP ( 'NONE', ( #5013, #11858, #34553, #28702 ) ) ;
#20477=VECTOR ( 'NONE', #17117, 1000.000000000000000 ) ;
#20480=CARTESIAN_POINT ( 'NONE',  ( 11.99999999999999645, 124.9999999999999716, 187.0000000000000000 ) ) ;
#20484=DIRECTION ( 'NONE',  ( -0.000000000000000000, 1.000000000000000000, -0.000000000000000000 ) ) ;
#20486=ORIENTED_EDGE ( 'NONE', *, *, #12465, .F. ) ;
#20490=EDGE_LOOP ( 'NONE', ( #29786, #9693, #33946, #31878, #34450, #30111, #14490, #10196 ) ) ;
#20491=CYLINDRICAL_SURFACE ( 'NONE', #25419, 7.999999999999979572 ) ;
#20500=DIRECTION ( 'NONE',  ( 0.000000000000000000, -1.000000000000000000, 0.000000000000000000 ) ) ;
#20502=CIRCLE ( 'NONE', #30742, 7.999999999999979572 ) ;
#20503=ORIENTED_EDGE ( 'NONE', *, *, #21100, .F. ) ;
#20505=ORIENTED_EDGE ( 'NONE', *, *, #14167, .T. ) ;
#20506=AXIS2_PLACEMENT_3D ( 'NONE', #21493, #782, #24974 ) ;
#20507=FACE_OUTER_BOUND ( 'NONE', #25906, .T. ) ;
#20508=AXIS2_PLACEMENT_3D ( 'NONE', #12417, #12582, #9900 ) ;
#20509=VERTEX_POINT ( 'NONE', #9932 ) ;
#20510=AXIS2_PLACEMENT_3D ( 'NONE', #33937, #28768, #31780 ) ;
#20511=ORIENTED_EDGE ( 'NONE', *, *, #18281, .F. ) ;
#20512=ORIENTED_EDGE ( 'NONE', *, *, #27413, .T. ) ;
#20522=EDGE_CURVE ( 'NONE', #32414, #6402, #29418, .T. ) ;
#20528=EDGE_CURVE ( 'NONE', #6277, #15141, #12966, .T. ) ;
#20529=LINE ( 'NONE', #23368, #4953 ) ;
#20531=EDGE_CURVE ( 'NONE', #26588, #25102, #18493, .T. ) ;
#20534=CARTESIAN_POINT ( 'NONE',  ( -410.0000000000000568, -104.9999999999999716, -187.0000000000000000 ) ) ;
#20536=LINE ( 'NONE', #8222, #12718 ) ;
#20540=AXIS2_PLACEMENT_3D ( 'NONE', #17315, #20660, #6769 ) ;
#20544=ORIENTED_EDGE ( 'NONE', *, *, #18078, .F. ) ;
#20547=DIRECTION ( 'NONE',  ( 1.232595164407830946E-32, 0.000000000000000000, 1.000000000000000000 ) ) ;
#20548=CARTESIAN_POINT ( 'NONE',  ( -363.0000000000000000, 124.9999999999999432, 168.9999999999999716 ) ) ;
#20550=CARTESIAN_POINT ( 'NONE',  ( -12.00000000000006573, -145.0000000000000000, -194.9999999999999432 ) ) ;
#20551=AXIS2_PLACEMENT_3D ( 'NONE', #24054, #24235, #31525 ) ;
#20552=ORIENTED_EDGE ( 'NONE', *, *, #21125, .T. ) ;
#20556=CARTESIAN_POINT ( 'NONE',  ( -20.00000000000007461, 112.9999999999999574, -190.9999999999999716 ) ) ;
#20558=EDGE_LOOP ( 'NONE', ( #11632, #25571, #2225, #20503 ) ) ;
#20562=DIRECTION ( 'NONE',  ( -1.000000000000000000, 0.000000000000000000, 0.000000000000000000 ) ) ;
#20566=EDGE_CURVE ( 'NONE', #16065, #28035, #2262, .T. ) ;
#20567=DIRECTION ( 'NONE',  ( 0.000000000000000000, 3.374343856708137958E-53, -1.000000000000000000 ) ) ;
#20568=DIRECTION ( 'NONE',  ( -3.040835319149746528E-31, -1.000000000000000000, 0.000000000000000000 ) ) ;
#20570=AXIS2_PLACEMENT_3D ( 'NONE', #17282, #20114, #17100 ) ;
#20574=DIRECTION ( 'NONE',  ( 1.000000000000000000, 0.000000000000000000, 1.300283923313630633E-47 ) ) ;
#20575=ORIENTED_EDGE ( 'NONE', *, *, #31080, .T. ) ;
#20578=DIRECTION ( 'NONE',  ( -1.000000000000000000, 0.000000000000000000, 0.000000000000000000 ) ) ;
#20580=EDGE_CURVE ( 'NONE', #21426, #27971, #8654, .T. ) ;
#20584=DIRECTION ( 'NONE',  ( 0.000000000000000000, -1.000000000000000000, 3.421138828918010427E-49 ) ) ;
#20585=ORIENTED_EDGE ( 'NONE', *, *, #6889, .F. ) ;
#20586=DIRECTION ( 'NONE',  ( 0.000000000000000000, -1.000000000000000000, 0.000000000000000000 ) ) ;
#20589=DIRECTION ( 'NONE',  ( 1.000000000000000000, 3.469446951953834515E-18, 0.000000000000000000 ) ) ;
#20592=VECTOR ( 'NONE', #8615, 1000.000000000000000 ) ;
#20593=ORIENTED_EDGE ( 'NONE', *, *, #28915, .F. ) ;
#20597=ORIENTED_EDGE ( 'NONE', *, *, #31544, .F. ) ;
#20599=EDGE_LOOP ( 'NONE', ( #17885, #3358, #6619, #22965 ) ) ;
#20601=EDGE_LOOP ( 'NONE', ( #15755, #2450, #7410, #32445, #30881, #16371, #33306, #6442 ) ) ;
#20602=DIRECTION ( 'NONE',  ( 0.000000000000000000, 1.000000000000000000, 1.224646799147353207E-16 ) ) ;
#20607=ORIENTED_EDGE ( 'NONE', *, *, #27436, .F. ) ;
#20609=EDGE_LOOP ( 'NONE', ( #7934, #17231, #33199, #1692 ) ) ;
#20611=PLANE ( 'NONE',  #6674 ) ;
#20612=EDGE_CURVE ( 'NONE', #23038, #26511, #5454, .T. ) ;
#20613=LINE ( 'NONE', #2259, #31293 ) ;
#20616=DIRECTION ( 'NONE',  ( 1.000000000000000000, 0.000000000000000000, 5.546364386991661285E-52 ) ) ;
#20618=AXIS2_PLACEMENT_3D ( 'NONE', #20891, #28728, #15217 ) ;
#20619=DIRECTION ( 'NONE',  ( 0.000000000000000000, 1.310824597558155437E-49, 1.000000000000000000 ) ) ;
#20622=EDGE_LOOP ( 'NONE', ( #13127, #22542, #8085, #351 ) ) ;
#20623=ADVANCED_FACE ( 'NONE', ( #8129 ), #10983, .T. ) ;
#20624=EDGE_CURVE ( 'NONE', #5775, #32496, #5619, .T. ) ;
#20626=EDGE_LOOP ( 'NONE', ( #2935, #27326, #29066, #11888 ) ) ;
#20628=ADVANCED_FACE ( 'NONE', ( #19354 ), #3317, .T. ) ;
#20630=VERTEX_POINT ( 'NONE', #35029 ) ;
#20631=LINE ( 'NONE', #6741, #26248 ) ;
#20636=VERTEX_POINT ( 'NONE', #32686 ) ;
#20643=VECTOR ( 'NONE', #6287, 1000.000000000000000 ) ;
#20649=ORIENTED_EDGE ( 'NONE', *, *, #19604, .T. ) ;
#20650=CARTESIAN_POINT ( 'NONE',  ( -12.00000000000001066, -145.0000000000000000, 187.0000000000000000 ) ) ;
#20651=LINE ( 'NONE', #18003, #30615 ) ;
#20653=CARTESIAN_POINT ( 'NONE',  ( -418.0000000000000000, -145.0000000000000000, -155.0000000000000000 ) ) ;
#20657=DIRECTION ( 'NONE',  ( 0.000000000000000000, 0.000000000000000000, -1.000000000000000000 ) ) ;
#20659=CARTESIAN_POINT ( 'NONE',  ( -445.9999999999999432, 105.0000000000000142, 107.9999999999999858 ) ) ;
#20660=DIRECTION ( 'NONE',  ( 0.000000000000000000, 1.000000000000000000, -2.465190328815661892E-32 ) ) ;
#20661=VERTEX_POINT ( 'NONE', #16875 ) ;
#20665=EDGE_CURVE ( 'NONE', #18227, #20630, #14012, .T. ) ;
#20670=FACE_OUTER_BOUND ( 'NONE', #25482, .T. ) ;
#20676=CARTESIAN_POINT ( 'NONE',  ( -418.0000000000000000, 109.0000000000000142, -155.0000000000000000 ) ) ;
#20680=EDGE_LOOP ( 'NONE', ( #13847, #14828, #3573, #11646, #26317, #3955, #20710, #3256 ) ) ;
#20682=VERTEX_POINT ( 'NONE', #11655 ) ;
#20683=EDGE_CURVE ( 'NONE', #11568, #24757, #29674, .T. ) ;
#20686=VECTOR ( 'NONE', #22656, 1000.000000000000000 ) ;
#20687=DIRECTION ( 'NONE',  ( 0.000000000000000000, 0.000000000000000000, 1.000000000000000000 ) ) ;
#20688=AXIS2_PLACEMENT_3D ( 'NONE', #30436, #23137, #23648 ) ;
#20690=ORIENTED_EDGE ( 'NONE', *, *, #23141, .T. ) ;
#20691=ORIENTED_EDGE ( 'NONE', *, *, #26475, .F. ) ;
#20692=CARTESIAN_POINT ( 'NONE',  ( -414.0000000000000568, 137.0000000000000000, 154.9999999999999716 ) ) ;
#20693=EDGE_CURVE ( 'NONE', #6940, #25387, #19010, .T. ) ;
#20698=ORIENTED_EDGE ( 'NONE', *, *, #31273, .T. ) ;
#20702=DIRECTION ( 'NONE',  ( 0.000000000000000000, 0.000000000000000000, 1.000000000000000000 ) ) ;
#20705=ORIENTED_EDGE ( 'NONE', *, *, #2133, .F. ) ;
#20706=FACE_OUTER_BOUND ( 'NONE', #34784, .T. ) ;
#20707=DIRECTION ( 'NONE',  ( 1.000000000000000000, 0.000000000000000000, 0.000000000000000000 ) ) ;
#20708=AXIS2_PLACEMENT_3D ( 'NONE', #7400, #21478, #5436 ) ;
#20709=CARTESIAN_POINT ( 'NONE',  ( -442.0000000000000000, -124.9999999999999716, 132.0000000000000000 ) ) ;
#20710=ORIENTED_EDGE ( 'NONE', *, *, #9993, .F. ) ;
#20711=AXIS2_PLACEMENT_3D ( 'NONE', #21264, #31590, #32112 ) ;
#20713=DIRECTION ( 'NONE',  ( -0.000000000000000000, -1.000000000000000000, -0.000000000000000000 ) ) ;
#20715=CARTESIAN_POINT ( 'NONE',  ( -499.9999999999999432, 112.9999999999999574, -159.0000000000000000 ) ) ;
#20718=AXIS2_PLACEMENT_3D ( 'NONE', #30481, #19811, #13757 ) ;
#20724=LINE ( 'NONE', #31568, #32195 ) ;
#20725=CIRCLE ( 'NONE', #1932, 3.999999999999976019 ) ;
#20729=EDGE_CURVE ( 'NONE', #13520, #7715, #20529, .T. ) ;
#20730=ADVANCED_FACE ( 'NONE', ( #31211 ), #26041, .T. ) ;
#20731=VECTOR ( 'NONE', #34257, 1000.000000000000000 ) ;
#20732=ORIENTED_EDGE ( 'NONE', *, *, #23047, .F. ) ;
#20734=ORIENTED_EDGE ( 'NONE', *, *, #27031, .T. ) ;
#20737=AXIS2_PLACEMENT_3D ( 'NONE', #33965, #34309, #9930 ) ;
#20739=VECTOR ( 'NONE', #25210, 1000.000000000000000 ) ;
#20741=CARTESIAN_POINT ( 'NONE',  ( -349.0000000000000000, -125.0000000000000284, 166.9999999999999716 ) ) ;
#20744=AXIS2_PLACEMENT_3D ( 'NONE', #5507, #3021, #34910 ) ;
#20746=LINE ( 'NONE', #18611, #18075 ) ;
#20748=CARTESIAN_POINT ( 'NONE',  ( -20.00000000000001776, -124.9999999999999432, -194.9999999999999432 ) ) ;
#20750=EDGE_LOOP ( 'NONE', ( #18798, #25060, #27462, #457, #354, #26721, #9912, #12333 ) ) ;
#20751=ORIENTED_EDGE ( 'NONE', *, *, #12397, .F. ) ;
#20754=ORIENTED_EDGE ( 'NONE', *, *, #32523, .F. ) ;
#20755=LINE ( 'NONE', #12756, #28150 ) ;
#20757=FACE_BOUND ( 'NONE', #5720, .T. ) ;
#20766=FACE_OUTER_BOUND ( 'NONE', #16882, .T. ) ;
#20768=AXIS2_PLACEMENT_3D ( 'NONE', #11848, #3626, #978 ) ;
#20779=AXIS2_PLACEMENT_3D ( 'NONE', #9620, #20310, #9453 ) ;
#20781=FACE_OUTER_BOUND ( 'NONE', #16167, .T. ) ;
#20783=ORIENTED_EDGE ( 'NONE', *, *, #7047, .T. ) ;
#20786=VECTOR ( 'NONE', #79, 1000.000000000000000 ) ;
#20788=DIRECTION ( 'NONE',  ( 1.000000000000000000, 0.000000000000000000, 0.000000000000000000 ) ) ;
#20789=LINE ( 'NONE', #7591, #26163 ) ;
#20792=ORIENTED_EDGE ( 'NONE', *, *, #8747, .F. ) ;
#20797=PLANE ( 'NONE',  #24555 ) ;
#20800=ORIENTED_EDGE ( 'NONE', *, *, #5450, .F. ) ;
#20805=DIRECTION ( 'NONE',  ( 1.000000000000000000, 0.000000000000000000, -1.848892746611746966E-32 ) ) ;
#20806=CARTESIAN_POINT ( 'NONE',  ( -442.0000000000000000, 137.0000000000000000, -155.0000000000000000 ) ) ;
#20808=ADVANCED_FACE ( 'NONE', ( #20706 ), #28372, .F. ) ;
#20809=ORIENTED_EDGE ( 'NONE', *, *, #22098, .F. ) ;
#20814=ORIENTED_EDGE ( 'NONE', *, *, #13751, .T. ) ;
#20815=CIRCLE ( 'NONE', #33318, 3.999999999999948042 ) ;
#20816=DIRECTION ( 'NONE',  ( -1.000000000000000000, -3.040835319149746528E-31, -1.232595164407830946E-32 ) ) ;
#20820=ADVANCED_FACE ( 'NONE', ( #14856 ), #25688, .T. ) ;
#20825=DIRECTION ( 'NONE',  ( 1.000000000000000000, 0.000000000000000000, -1.848892746611746966E-32 ) ) ;
#20834=VERTEX_POINT ( 'NONE', #6988 ) ;
#20837=VECTOR ( 'NONE', #10384, 1000.000000000000000 ) ;
#20839=DIRECTION ( 'NONE',  ( 1.000000000000000000, 0.000000000000000000, 0.000000000000000000 ) ) ;
#20841=LINE ( 'NONE', #4801, #11149 ) ;
#20844=LINE ( 'NONE', #9988, #26958 ) ;
#20847=AXIS2_PLACEMENT_3D ( 'NONE', #17498, #746, #3758 ) ;
#20849=ORIENTED_EDGE ( 'NONE', *, *, #29812, .T. ) ;
#20851=ORIENTED_EDGE ( 'NONE', *, *, #17253, .F. ) ;
#20854=EDGE_CURVE ( 'NONE', #9586, #16454, #3815, .T. ) ;
#20858=VERTEX_POINT ( 'NONE', #23032 ) ;
#20860=ORIENTED_EDGE ( 'NONE', *, *, #30493, .F. ) ;
#20863=ORIENTED_EDGE ( 'NONE', *, *, #2955, .F. ) ;
#20864=DIRECTION ( 'NONE',  ( 1.000000000000000000, -0.000000000000000000, -0.000000000000000000 ) ) ;
#20865=PLANE ( 'NONE',  #13164 ) ;
#20871=LINE ( 'NONE', #17535, #7430 ) ;
#20877=CARTESIAN_POINT ( 'NONE',  ( -349.0000000000000000, 124.9999999999999432, 181.0000000000000000 ) ) ;
#20880=ADVANCED_FACE ( 'NONE', ( #16078, #16258, #4652 ), #29762, .T. ) ;
#20881=DIRECTION ( 'NONE',  ( 2.530127506375325574E-80, -1.000000000000000000, -6.842277657836020854E-49 ) ) ;
#20884=CARTESIAN_POINT ( 'NONE',  ( -355.0000000000000000, 114.9999999999999574, 113.9999999999999858 ) ) ;
#20887=EDGE_CURVE ( 'NONE', #16498, #10319, #13054, .T. ) ;
#20889=ORIENTED_EDGE ( 'NONE', *, *, #22948, .F. ) ;
#20891=CARTESIAN_POINT ( 'NONE',  ( -70.00000000000000000, 4.559999999999908127, -172.9900000000000091 ) ) ;
#20893=EDGE_CURVE ( 'NONE', #12400, #27222, #10197, .T. ) ;
#20896=FACE_OUTER_BOUND ( 'NONE', #20601, .T. ) ;
#20900=EDGE_CURVE ( 'NONE', #26996, #8677, #3259, .T. ) ;
#20903=DIRECTION ( 'NONE',  ( 0.000000000000000000, 0.000000000000000000, -1.000000000000000000 ) ) ;
#20905=ORIENTED_EDGE ( 'NONE', *, *, #30814, .T. ) ;
#20909=ORIENTED_EDGE ( 'NONE', *, *, #22232, .F. ) ;
#20916=UNCERTAINTY_MEASURE_WITH_UNIT (LENGTH_MEASURE( 1.000000000000000082E-05 ), #5764, 'distance_accuracy_value', 'NONE');
#20917=ORIENTED_EDGE ( 'NONE', *, *, #25635, .T. ) ;
#20918=ORIENTED_EDGE ( 'NONE', *, *, #22209, .T. ) ;
#20920=AXIS2_PLACEMENT_3D ( 'NONE', #13603, #5398, #5565 ) ;
#20921=CARTESIAN_POINT ( 'NONE',  ( -442.0000000000000000, -112.9999999999999858, -174.9999999999999716 ) ) ;
#20923=DIRECTION ( 'NONE',  ( 0.000000000000000000, -1.000000000000000000, -1.224646799147353207E-16 ) ) ;
#20924=DIRECTION ( 'NONE',  ( -1.000000000000000000, 0.000000000000000000, -0.000000000000000000 ) ) ;
#20925=DIRECTION ( 'NONE',  ( 1.000000000000000000, 3.040835319149746090E-31, 1.232595164407830946E-32 ) ) ;
#20926=ORIENTED_EDGE ( 'NONE', *, *, #30453, .T. ) ;
#20928=CARTESIAN_POINT ( 'NONE',  ( -20.00000000000004619, 124.9999999999999716, 155.0000000000000000 ) ) ;
#20929=ORIENTED_EDGE ( 'NONE', *, *, #32824, .F. ) ;
#20930=CIRCLE ( 'NONE', #23224, 4.750000000000004441 ) ;
#20931=ADVANCED_FACE ( 'NONE', ( #21582 ), #18583, .T. ) ;
#20933=DIRECTION ( 'NONE',  ( 0.000000000000000000, 0.000000000000000000, -1.000000000000000000 ) ) ;
#20934=ORIENTED_EDGE ( 'NONE', *, *, #20299, .T. ) ;
#20935=FACE_OUTER_BOUND ( 'NONE', #18864, .T. ) ;
#20940=ORIENTED_EDGE ( 'NONE', *, *, #26178, .F. ) ;
#20941=CARTESIAN_POINT ( 'NONE',  ( -19.99999999999996092, -141.0000000000000000, 187.0000000000000000 ) ) ;
#20942=EDGE_CURVE ( 'NONE', #7557, #169, #10900, .T. ) ;
#20943=DIRECTION ( 'NONE',  ( 0.000000000000000000, 1.000000000000000000, -3.374343856708137958E-53 ) ) ;
#20947=ORIENTED_EDGE ( 'NONE', *, *, #2911, .F. ) ;
#20948=LINE ( 'NONE', #34652, #3390 ) ;
#20951=CARTESIAN_POINT ( 'NONE',  ( 19.99999999999998934, 136.9999999999999716, 155.0000000000000000 ) ) ;
#20952=VECTOR ( 'NONE', #23623, 1000.000000000000000 ) ;
#20954=PLANE ( 'NONE',  #15969 ) ;
#20956=ORIENTED_EDGE ( 'NONE', *, *, #21355, .F. ) ;
#20958=ORIENTED_EDGE ( 'NONE', *, *, #28480, .T. ) ;
#20959=EDGE_CURVE ( 'NONE', #11922, #9216, #15913, .T. ) ;
#20962=AXIS2_PLACEMENT_3D ( 'NONE', #6687, #8837, #6151 ) ;
#20964=CARTESIAN_POINT ( 'NONE',  ( -20.00000000000007461, -113.0000000000000000, -187.0000000000000000 ) ) ;
#20967=ORIENTED_EDGE ( 'NONE', *, *, #34712, .T. ) ;
#20970=PLANE ( 'NONE',  #34791 ) ;
#20971=ADVANCED_FACE ( 'NONE', ( #21227 ), #32071, .F. ) ;
#20973=ORIENTED_EDGE ( 'NONE', *, *, #30172, .F. ) ;
#20974=ADVANCED_FACE ( 'NONE', ( #26735 ), #27089, .F. ) ;
#20975=VECTOR ( 'NONE', #15242, 1000.000000000000000 ) ;
#20976=LINE ( 'NONE', #32177, #29173 ) ;
#20979=FACE_BOUND ( 'NONE', #32470, .T. ) ;
#20982=CARTESIAN_POINT ( 'NONE',  ( -361.0000000000000000, 124.9999999999999432, 185.0000000000000000 ) ) ;
#20985=EDGE_LOOP ( 'NONE', ( #29135, #23054, #10001, #17088 ) ) ;
#20991=VECTOR ( 'NONE', #4647, 1000.000000000000000 ) ;
#20992=DIRECTION ( 'NONE',  ( 2.891205793294675861E-16, 0.000000000000000000, -1.000000000000000000 ) ) ;
#20999=ORIENTED_EDGE ( 'NONE', *, *, #16173, .T. ) ;
#21000=ORIENTED_EDGE ( 'NONE', *, *, #5123, .F. ) ;
#21001=CARTESIAN_POINT ( 'NONE',  ( 12.00000000000001066, 144.9999999999999716, -154.9999999999999716 ) ) ;
#21004=ADVANCED_FACE ( 'NONE', ( #32252 ), #2871, .T. ) ;
#21013=EDGE_CURVE ( 'NONE', #7844, #14586, #22283, .T. ) ;
#21018=PLANE ( 'NONE',  #27039 ) ;
#21023=CARTESIAN_POINT ( 'NONE',  ( 15.99999999999998579, -55.00000000000000711, 0.000000000000000000 ) ) ;
#21026=ORIENTED_EDGE ( 'NONE', *, *, #24615, .T. ) ;
#21031=ORIENTED_EDGE ( 'NONE', *, *, #32221, .F. ) ;
#21032=ORIENTED_EDGE ( 'NONE', *, *, #30453, .F. ) ;
#21036=ORIENTED_EDGE ( 'NONE', *, *, #12534, .T. ) ;
#21039=VERTEX_POINT ( 'NONE', #22461 ) ;
#21043=LINE ( 'NONE', #29413, #20991 ) ;
#21048=DIRECTION ( 'NONE',  ( 1.000000000000000000, 3.469446951953834515E-18, 0.000000000000000000 ) ) ;
#21052=EDGE_CURVE ( 'NONE', #29922, #1478, #1592, .T. ) ;
#21056=DIRECTION ( 'NONE',  ( 0.000000000000000000, 1.000000000000000000, 5.145227585319922065E-49 ) ) ;
#21057=EDGE_CURVE ( 'NONE', #14037, #8068, #24289, .T. ) ;
#21060=ORIENTED_EDGE ( 'NONE', *, *, #22945, .T. ) ;
#21065=FACE_OUTER_BOUND ( 'NONE', #14166, .T. ) ;
#21071=DIRECTION ( 'NONE',  ( -0.000000000000000000, -0.000000000000000000, -1.000000000000000000 ) ) ;
#21073=EDGE_LOOP ( 'NONE', ( #1817, #2068, #3738, #21432 ) ) ;
#21074=CIRCLE ( 'NONE', #33575, 4.000000000000003553 ) ;
#21075=CARTESIAN_POINT ( 'NONE',  ( -442.0000000000000000, 109.0000000000000142, -175.0000000000000000 ) ) ;
#21077=ADVANCED_FACE ( 'NONE', ( #22111 ), #14284, .T. ) ;
#21082=ORIENTED_EDGE ( 'NONE', *, *, #26719, .F. ) ;
#21084=DIRECTION ( 'NONE',  ( 0.000000000000000000, 0.000000000000000000, -1.000000000000000000 ) ) ;
#21087=CARTESIAN_POINT ( 'NONE',  ( 11.99999999999999645, 108.9999999999999858, -155.0000000000000000 ) ) ;
#21089=CARTESIAN_POINT ( 'NONE',  ( -449.9999999999999432, -112.9999999999999858, 155.0000000000000000 ) ) ;
#21090=CIRCLE ( 'NONE', #31302, 7.999999999999986677 ) ;
#21092=ORIENTED_EDGE ( 'NONE', *, *, #24817, .F. ) ;
#21093=CIRCLE ( 'NONE', #16005, 7.999999999999979572 ) ;
#21095=DIRECTION ( 'NONE',  ( 1.000000000000000000, 0.000000000000000000, 0.000000000000000000 ) ) ;
#21100=EDGE_CURVE ( 'NONE', #2320, #30770, #24876, .T. ) ;
#21102=DIRECTION ( 'NONE',  ( -0.000000000000000000, -5.053935297177146739E-49, -1.000000000000000000 ) ) ;
#21109=ORIENTED_EDGE ( 'NONE', *, *, #6706, .T. ) ;
#21110=CYLINDRICAL_SURFACE ( 'NONE', #8052, 7.999999999999986677 ) ;
#21121=DIRECTION ( 'NONE',  ( 0.000000000000000000, 0.000000000000000000, -1.000000000000000000 ) ) ;
#21123=ADVANCED_FACE ( 'NONE', ( #13746 ), #217, .F. ) ;
#21125=EDGE_CURVE ( 'NONE', #12453, #19297, #21350, .T. ) ;
#21126=LINE ( 'NONE', #23798, #27106 ) ;
#21128=ORIENTED_EDGE ( 'NONE', *, *, #553, .F. ) ;
#21134=CYLINDRICAL_SURFACE ( 'NONE', #5397, 4.000000000000003553 ) ;
#21136=CARTESIAN_POINT ( 'NONE',  ( -355.0000000000000000, 130.9999999999999716, 126.0000000000000000 ) ) ;
#21138=ORIENTED_EDGE ( 'NONE', *, *, #6962, .F. ) ;
#21140=PLANE ( 'NONE',  #5449 ) ;
#21143=FACE_BOUND ( 'NONE', #12728, .T. ) ;
#21146=VECTOR ( 'NONE', #6514, 1000.000000000000000 ) ;
#21147=CIRCLE ( 'NONE', #6376, 7.999999999999979572 ) ;
#21149=ORIENTED_EDGE ( 'NONE', *, *, #4803, .F. ) ;
#21151=CARTESIAN_POINT ( 'NONE',  ( -365.0000000000000000, -119.0000000000000000, 111.9999999999999858 ) ) ;
#21152=PLANE ( 'NONE',  #3628 ) ;
#21155=CARTESIAN_POINT ( 'NONE',  ( -361.0000000000000000, 134.9999999999999716, 130.0000000000000000 ) ) ;
#21160=ORIENTED_EDGE ( 'NONE', *, *, #34012, .F. ) ;
#21166=VECTOR ( 'NONE', #10416, 1000.000000000000000 ) ;
#21171=VECTOR ( 'NONE', #460, 1000.000000000000000 ) ;
#21176=DIRECTION ( 'NONE',  ( -8.433758354584418579E-81, 1.000000000000000000, 3.421138828918010427E-49 ) ) ;
#21180=ORIENTED_EDGE ( 'NONE', *, *, #33674, .F. ) ;
#21182=DIRECTION ( 'NONE',  ( 0.000000000000000000, 0.000000000000000000, 1.000000000000000000 ) ) ;
#21183=ORIENTED_EDGE ( 'NONE', *, *, #28915, .T. ) ;
#21186=EDGE_LOOP ( 'NONE', ( #25795, #29377, #31531, #24047 ) ) ;
#21190=CARTESIAN_POINT ( 'NONE',  ( -418.0000000000000000, -125.0000000000000000, 187.0000000000000000 ) ) ;
#21193=VECTOR ( 'NONE', #362, 1000.000000000000000 ) ;
#21195=VECTOR ( 'NONE', #22905, 1000.000000000000000 ) ;
#21197=LINE ( 'NONE', #15884, #17894 ) ;
#21198=DIRECTION ( 'NONE',  ( 0.000000000000000000, -1.000000000000000000, 0.000000000000000000 ) ) ;
#21199=ORIENTED_EDGE ( 'NONE', *, *, #2870, .F. ) ;
#21202=ORIENTED_EDGE ( 'NONE', *, *, #18176, .T. ) ;
#21204=EDGE_CURVE ( 'NONE', #6833, #9096, #8156, .T. ) ;
#21205=VECTOR ( 'NONE', #20713, 1000.000000000000000 ) ;
#21209=ORIENTED_EDGE ( 'NONE', *, *, #16051, .F. ) ;
#21218=ORIENTED_EDGE ( 'NONE', *, *, #17226, .F. ) ;
#21219=ORIENTED_EDGE ( 'NONE', *, *, #1546, .T. ) ;
#21221=DIRECTION ( 'NONE',  ( 0.000000000000000000, -1.310824597558155437E-49, -1.000000000000000000 ) ) ;
#21223=DIRECTION ( 'NONE',  ( 0.000000000000000000, -1.000000000000000000, -1.131431318426415506E-52 ) ) ;
#21227=FACE_OUTER_BOUND ( 'NONE', #32895, .T. ) ;
#21231=CYLINDRICAL_SURFACE ( 'NONE', #1328, 7.999999999999979572 ) ;
#21234=CARTESIAN_POINT ( 'NONE',  ( 20.00000000000001776, -145.0000000000000000, -162.9999999999999432 ) ) ;
#21235=AXIS2_PLACEMENT_3D ( 'NONE', #32888, #19381, #5821 ) ;
#21236=DIRECTION ( 'NONE',  ( 0.000000000000000000, 0.000000000000000000, -1.000000000000000000 ) ) ;
#21238=DIRECTION ( 'NONE',  ( 0.000000000000000000, 0.000000000000000000, -1.000000000000000000 ) ) ;
#21240=DIRECTION ( 'NONE',  ( 0.000000000000000000, -1.000000000000000000, -2.465190328815662439E-32 ) ) ;
#21244=CIRCLE ( 'NONE', #13283, 7.999999999999979572 ) ;
#21249=ORIENTED_EDGE ( 'NONE', *, *, #13495, .T. ) ;
#21251=VERTEX_POINT ( 'NONE', #26850 ) ;
#21255=EDGE_CURVE ( 'NONE', #27132, #26055, #15818, .T. ) ;
#21258=DIRECTION ( 'NONE',  ( 0.000000000000000000, 0.000000000000000000, -1.000000000000000000 ) ) ;
#21259=EDGE_CURVE ( 'NONE', #3590, #15373, #33986, .T. ) ;
#21262=ORIENTED_EDGE ( 'NONE', *, *, #5750, .T. ) ;
#21263=CARTESIAN_POINT ( 'NONE',  ( 15.99999999999997868, -145.0000000000000000, 187.0000000000000000 ) ) ;
#21264=CARTESIAN_POINT ( 'NONE',  ( 11.99999999999999645, -137.0000000000000000, 155.0000000000000000 ) ) ;
#21266=EDGE_CURVE ( 'NONE', #15011, #2208, #15253, .T. ) ;
#21267=CYLINDRICAL_SURFACE ( 'NONE', #16462, 4.000000000000003553 ) ;
#21271=CARTESIAN_POINT ( 'NONE',  ( -445.9999999999999432, -105.0000000000000142, -101.9999999999999858 ) ) ;
#21272=VECTOR ( 'NONE', #19813, 1000.000000000000000 ) ;
#21273=CIRCLE ( 'NONE', #11606, 3.999999999999976019 ) ;
#21274=DIRECTION ( 'NONE',  ( 0.000000000000000000, 2.309213040847544338E-50, 1.000000000000000000 ) ) ;
#21277=CARTESIAN_POINT ( 'NONE',  ( -445.9999999999999432, 137.0000000000000000, 154.9999999999999716 ) ) ;
#21278=CARTESIAN_POINT ( 'NONE',  ( -349.0000000000000000, 124.9999999999999432, 166.9999999999999716 ) ) ;
#21280=ORIENTED_EDGE ( 'NONE', *, *, #28565, .T. ) ;
#21281=CARTESIAN_POINT ( 'NONE',  ( 11.99999999999999645, -115.0000000000000000, 162.9999999999999716 ) ) ;
#21284=CARTESIAN_POINT ( 'NONE',  ( -418.0000000000000000, 137.0000000000000000, 154.9999999999999716 ) ) ;
#21289=CIRCLE ( 'NONE', #4802, 7.999999999999979572 ) ;
#21293=VECTOR ( 'NONE', #20825, 1000.000000000000000 ) ;
#21294=ORIENTED_EDGE ( 'NONE', *, *, #21699, .F. ) ;
#21295=ADVANCED_FACE ( 'NONE', ( #21065 ), #18419, .T. ) ;
#21298=CIRCLE ( 'NONE', #14483, 7.999999999999979572 ) ;
#21301=EDGE_LOOP ( 'NONE', ( #28815, #32671, #11155, #6142 ) ) ;
#21303=EDGE_CURVE ( 'NONE', #30541, #196, #21932, .T. ) ;
#21304=LINE ( 'NONE', #15806, #533 ) ;
#21305=LINE ( 'NONE', #29320, #3249 ) ;
#21306=LINE ( 'NONE', #7763, #1168 ) ;
#21307=EDGE_CURVE ( 'NONE', #29646, #20682, #8404, .T. ) ;
#21309=EDGE_CURVE ( 'NONE', #28119, #30776, #18082, .T. ) ;
#21310=EDGE_LOOP ( 'NONE', ( #33622, #17109, #6261, #2030 ) ) ;
#21311=ORIENTED_EDGE ( 'NONE', *, *, #33182, .F. ) ;
#21312=CARTESIAN_POINT ( 'NONE',  ( -499.9999999999999432, 112.9999999999999574, 162.9999999999999716 ) ) ;
#21314=PLANE ( 'NONE',  #25108 ) ;
#21317=DIRECTION ( 'NONE',  ( 0.000000000000000000, 0.000000000000000000, -1.000000000000000000 ) ) ;
#21318=CARTESIAN_POINT ( 'NONE',  ( -347.0000000000000000, 134.9999999999999716, 125.9999999999999716 ) ) ;
#21320=ORIENTED_EDGE ( 'NONE', *, *, #10314, .T. ) ;
#21325=CARTESIAN_POINT ( 'NONE',  ( -15.99999999999998579, 136.9999999999999716, -155.0000000000000000 ) ) ;
#21326=ORIENTED_EDGE ( 'NONE', *, *, #12979, .F. ) ;
#21328=AXIS2_PLACEMENT_3D ( 'NONE', #34906, #9984, #8497 ) ;
#21329=VECTOR ( 'NONE', #29167, 1000.000000000000000 ) ;
#21331=ORIENTED_EDGE ( 'NONE', *, *, #28209, .T. ) ;
#21334=EDGE_CURVE ( 'NONE', #17164, #30600, #32948, .T. ) ;
#21335=DIRECTION ( 'NONE',  ( 0.000000000000000000, 1.000000000000000000, 1.224646799147353207E-16 ) ) ;
#21336=ADVANCED_FACE ( 'NONE', ( #18755 ), #3054, .F. ) ;
#21340=FACE_OUTER_BOUND ( 'NONE', #9883, .T. ) ;
#21342=DIRECTION ( 'NONE',  ( -1.000000000000000000, 0.000000000000000000, 0.000000000000000000 ) ) ;
#21344=ORIENTED_EDGE ( 'NONE', *, *, #11001, .T. ) ;
#21345=VECTOR ( 'NONE', #8478, 1000.000000000000000 ) ;
#21349=ORIENTED_EDGE ( 'NONE', *, *, #626, .T. ) ;
#21350=LINE ( 'NONE', #13163, #32830 ) ;
#21355=EDGE_CURVE ( 'NONE', #4287, #9216, #32777, .T. ) ;
#21357=ORIENTED_EDGE ( 'NONE', *, *, #11781, .F. ) ;
#21358=DIRECTION ( 'NONE',  ( 0.000000000000000000, 0.000000000000000000, -1.000000000000000000 ) ) ;
#21363=ORIENTED_EDGE ( 'NONE', *, *, #3107, .F. ) ;
#21365=ORIENTED_EDGE ( 'NONE', *, *, #19305, .F. ) ;
#21368=ORIENTED_EDGE ( 'NONE', *, *, #30326, .F. ) ;
#21372=EDGE_LOOP ( 'NONE', ( #22123, #25472, #12046, #20754 ) ) ;
#21374=CARTESIAN_POINT ( 'NONE',  ( -449.9999999999999432, -105.0000000000000142, 187.0000000000000000 ) ) ;
#21376=CARTESIAN_POINT ( 'NONE',  ( 15.99999999999997868, 144.9999999999999716, -186.9999999999999716 ) ) ;
#21377=ADVANCED_FACE ( 'NONE', ( #13578 ), #11259, .F. ) ;
#21379=CARTESIAN_POINT ( 'NONE',  ( -19.99999999999998934, 144.9999999999999716, -186.9999999999999716 ) ) ;
#21380=EDGE_CURVE ( 'NONE', #28865, #30842, #5017, .T. ) ;
#21381=CARTESIAN_POINT ( 'NONE',  ( -365.0000000000000000, -135.0000000000000000, 126.0000000000000000 ) ) ;
#21382=LINE ( 'NONE', #27236, #12251 ) ;
#21384=ORIENTED_EDGE ( 'NONE', *, *, #15762, .F. ) ;
#21388=ORIENTED_EDGE ( 'NONE', *, *, #26542, .T. ) ;
#21393=CARTESIAN_POINT ( 'NONE',  ( -20.00000000000004619, -134.9999999999999716, -186.9999999999999716 ) ) ;
#21394=AXIS2_PLACEMENT_3D ( 'NONE', #14285, #22810, #3757 ) ;
#21403=CARTESIAN_POINT ( 'NONE',  ( -414.0000000000000568, 113.0000000000000000, -155.0000000000000000 ) ) ;
#21407=DIRECTION ( 'NONE',  ( 1.000000000000000000, -0.000000000000000000, -0.000000000000000000 ) ) ;
#21408=FACE_OUTER_BOUND ( 'NONE', #3798, .T. ) ;
#21409=CARTESIAN_POINT ( 'NONE',  ( -442.0000000000000000, 113.0000000000000000, 154.9999999999999716 ) ) ;
#21412=EDGE_CURVE ( 'NONE', #19565, #27398, #10738, .T. ) ;
#21413=DIRECTION ( 'NONE',  ( 0.000000000000000000, 0.000000000000000000, 1.000000000000000000 ) ) ;
#21414=FACE_OUTER_BOUND ( 'NONE', #27104, .T. ) ;
#21418=AXIS2_PLACEMENT_3D ( 'NONE', #25956, #28625, #25773 ) ;
#21420=DIRECTION ( 'NONE',  ( -0.000000000000000000, 1.000000000000000000, -0.000000000000000000 ) ) ;
#21421=ORIENTED_EDGE ( 'NONE', *, *, #10566, .T. ) ;
#21426=VERTEX_POINT ( 'NONE', #19105 ) ;
#21427=DIRECTION ( 'NONE',  ( -0.000000000000000000, -0.000000000000000000, 1.000000000000000000 ) ) ;
#21428=ORIENTED_EDGE ( 'NONE', *, *, #21846, .F. ) ;
#21430=DIRECTION ( 'NONE',  ( 0.000000000000000000, -2.309213040847544338E-50, -1.000000000000000000 ) ) ;
#21432=ORIENTED_EDGE ( 'NONE', *, *, #27234, .F. ) ;
#21433=CARTESIAN_POINT ( 'NONE',  ( -355.0000000000000000, -114.9999999999999858, 113.9999999999999858 ) ) ;
#21438=EDGE_LOOP ( 'NONE', ( #15604, #14243, #7638, #21183, #1230, #2477, #19994, #32962 ) ) ;
#21446=DIRECTION ( 'NONE',  ( 0.000000000000000000, 0.000000000000000000, -1.000000000000000000 ) ) ;
#21450=CARTESIAN_POINT ( 'NONE',  ( -449.9999999999999432, -105.0000000000000142, 131.9999999999999716 ) ) ;
#21451=FACE_OUTER_BOUND ( 'NONE', #20599, .T. ) ;
#21456=VERTEX_POINT ( 'NONE', #22285 ) ;
#21457=VECTOR ( 'NONE', #14241, 1000.000000000000000 ) ;
#21458=DIRECTION ( 'NONE',  ( 0.000000000000000000, 1.000000000000000000, -3.374343856708137958E-53 ) ) ;
#21459=VECTOR ( 'NONE', #15763, 1000.000000000000000 ) ;
#21461=ADVANCED_FACE ( 'NONE', ( #14286 ), #11426, .F. ) ;
#21463=LINE ( 'NONE', #7389, #19131 ) ;
#21467=ORIENTED_EDGE ( 'NONE', *, *, #9330, .T. ) ;
#21468=( LENGTH_UNIT ( ) NAMED_UNIT ( * ) SI_UNIT ( .MILLI., .METRE. ) );
#21471=VERTEX_POINT ( 'NONE', #24937 ) ;
#21473=MECHANICAL_DESIGN_GEOMETRIC_PRESENTATION_REPRESENTATION('',(#27759),#9536);
#21477=ORIENTED_EDGE ( 'NONE', *, *, #6848, .F. ) ;
#21478=DIRECTION ( 'NONE',  ( 1.000000000000000000, 3.040835319149746528E-31, 1.232595164407830946E-32 ) ) ;
#21479=CARTESIAN_POINT ( 'NONE',  ( -20.00000000000007461, 140.9999999999999716, 187.0000000000000000 ) ) ;
#21484=ORIENTED_EDGE ( 'NONE', *, *, #29737, .F. ) ;
#21489=CARTESIAN_POINT ( 'NONE',  ( -430.0000000000000000, -117.0000000000000000, 113.9999999999999858 ) ) ;
#21491=VECTOR ( 'NONE', #31680, 1000.000000000000000 ) ;
#21493=CARTESIAN_POINT ( 'NONE',  ( -418.0000000000000000, 104.9999999999999858, -187.0000000000000000 ) ) ;
#21497=ORIENTED_EDGE ( 'NONE', *, *, #2377, .T. ) ;
#21501=CARTESIAN_POINT ( 'NONE',  ( -418.0000000000000000, -105.0000000000000142, 139.9999999999999716 ) ) ;
#21502=VERTEX_POINT ( 'NONE', #11615 ) ;
#21503=DIRECTION ( 'NONE',  ( -3.469446951953832974E-18, -1.000000000000000000, -7.888609052210116302E-31 ) ) ;
#21513=PLANE ( 'NONE',  #878 ) ;
#21514=LINE ( 'NONE', #16008, #7478 ) ;
#21519=AXIS2_PLACEMENT_3D ( 'NONE', #2291, #34886, #21358 ) ;
#21520=CARTESIAN_POINT ( 'NONE',  ( -12.00000000000001066, -124.9999999999999432, -158.9999999999999716 ) ) ;
#21523=EDGE_CURVE ( 'NONE', #4201, #19566, #25294, .T. ) ;
#21525=DIRECTION ( 'NONE',  ( 1.000000000000000000, 3.040835319149746090E-31, 1.232595164407830946E-32 ) ) ;
#21526=CARTESIAN_POINT ( 'NONE',  ( -20.00000000000007461, 112.9999999999999574, -162.9999999999999716 ) ) ;
#21528=ORIENTED_EDGE ( 'NONE', *, *, #19369, .T. ) ;
#21529=CARTESIAN_POINT ( 'NONE',  ( -418.0000000000000000, 124.9999999999999432, -159.0000000000000000 ) ) ;
#21532=LINE ( 'NONE', #18868, #19577 ) ;
#21536=EDGE_LOOP ( 'NONE', ( #21477, #18715, #9169, #12185 ) ) ;
#21537=VERTEX_POINT ( 'NONE', #30288 ) ;
#21539=ORIENTED_EDGE ( 'NONE', *, *, #24859, .T. ) ;
#21541=DIRECTION ( 'NONE',  ( -0.000000000000000000, 1.000000000000000000, -0.000000000000000000 ) ) ;
#21542=ORIENTED_EDGE ( 'NONE', *, *, #25634, .F. ) ;
#21543=STYLED_ITEM('',(#35254),#10344);
#21548=LINE ( 'NONE', #8006, #2705 ) ;
#21550=LINE ( 'NONE', #7832, #28058 ) ;
#21551=DIRECTION ( 'NONE',  ( 2.891205793294675861E-16, 0.000000000000000000, -1.000000000000000000 ) ) ;
#21552=EDGE_CURVE ( 'NONE', #6402, #5434, #5890, .T. ) ;
#21553=EDGE_CURVE ( 'NONE', #9444, #7282, #6598, .T. ) ;
#21557=EDGE_CURVE ( 'NONE', #19179, #10465, #19163, .T. ) ;
#21558=AXIS2_PLACEMENT_3D ( 'NONE', #18914, #32591, #19099 ) ;
#21559=EDGE_LOOP ( 'NONE', ( #26323, #4406, #34357, #15450, #14803, #22783, #32378, #11818 ) ) ;
#21562=EDGE_LOOP ( 'NONE', ( #18451, #24895, #21368, #19738 ) ) ;
#21567=ORIENTED_EDGE ( 'NONE', *, *, #11927, .T. ) ;
#21571=EDGE_CURVE ( 'NONE', #28489, #4850, #7288, .T. ) ;
#21574=ORIENTED_EDGE ( 'NONE', *, *, #22390, .F. ) ;
#21575=CARTESIAN_POINT ( 'NONE',  ( -19.99999999999998934, -56.99999999999996447, 155.0000000000000000 ) ) ;
#21579=CARTESIAN_POINT ( 'NONE',  ( -19.99999999999998934, 75.55999999999990280, 168.2400000000000091 ) ) ;
#21582=FACE_OUTER_BOUND ( 'NONE', #5610, .T. ) ;
#21585=EDGE_CURVE ( 'NONE', #5794, #5593, #12487, .T. ) ;
#21589=CYLINDRICAL_SURFACE ( 'NONE', #34855, 3.999999999999976019 ) ;
#21595=DIRECTION ( 'NONE',  ( 0.000000000000000000, -1.000000000000000000, -1.224646799147353207E-16 ) ) ;
#21598=EDGE_LOOP ( 'NONE', ( #31022, #516, #24284, #29189 ) ) ;
#21600=EDGE_CURVE ( 'NONE', #11445, #763, #17664, .T. ) ;
#21607=ADVANCED_FACE ( 'NONE', ( #26344 ), #29196, .T. ) ;
#21608=EDGE_CURVE ( 'NONE', #3207, #8431, #22565, .T. ) ;
#21610=FACE_OUTER_BOUND ( 'NONE', #30433, .T. ) ;
#21617=CARTESIAN_POINT ( 'NONE',  ( -445.9999999999999432, -112.9999999999999858, 155.0000000000000000 ) ) ;
#21618=ORIENTED_EDGE ( 'NONE', *, *, #21961, .F. ) ;
#21620=DIRECTION ( 'NONE',  ( -1.000000000000000000, 0.000000000000000000, 0.000000000000000000 ) ) ;
#21621=ORIENTED_EDGE ( 'NONE', *, *, #7351, .F. ) ;
#21622=CARTESIAN_POINT ( 'NONE',  ( -414.0000000000000568, 105.0000000000000142, -101.9999999999999858 ) ) ;
#21625=CARTESIAN_POINT ( 'NONE',  ( -11.99999999999998224, -134.9999999999999716, 155.0000000000000000 ) ) ;
#21626=ORIENTED_EDGE ( 'NONE', *, *, #32576, .T. ) ;
#21629=EDGE_LOOP ( 'NONE', ( #30897, #24322, #14121, #9885 ) ) ;
#21631=DIRECTION ( 'NONE',  ( 0.000000000000000000, 0.000000000000000000, -1.000000000000000000 ) ) ;
#21633=VERTEX_POINT ( 'NONE', #18357 ) ;
#21634=CARTESIAN_POINT ( 'NONE',  ( -449.9999999999999432, 105.0000000000000142, 162.9999999999999716 ) ) ;
#21638=ORIENTED_EDGE ( 'NONE', *, *, #7088, .F. ) ;
#21641=VERTEX_POINT ( 'NONE', #4444 ) ;
#21644=ADVANCED_FACE ( 'NONE', ( #34008 ), #31173, .T. ) ;
#21646=DIRECTION ( 'NONE',  ( 0.000000000000000000, 0.000000000000000000, 1.000000000000000000 ) ) ;
#21648=DIRECTION ( 'NONE',  ( 0.000000000000000000, 0.000000000000000000, 1.000000000000000000 ) ) ;
#21653=EDGE_CURVE ( 'NONE', #29676, #7312, #11204, .T. ) ;
#21654=CARTESIAN_POINT ( 'NONE',  ( -499.9999999999999432, 144.9999999999999716, 162.9999999999999716 ) ) ;
#21656=CARTESIAN_POINT ( 'NONE',  ( -500.0000000000000000, -137.0000000000000000, 159.0000000000000000 ) ) ;
#21657=CARTESIAN_POINT ( 'NONE',  ( -355.0000000000000000, 116.9999999999999716, 113.9999999999999858 ) ) ;
#21658=CARTESIAN_POINT ( 'NONE',  ( 11.99999999999999645, 134.9999999999998863, 194.9999999999999716 ) ) ;
#21661=CIRCLE ( 'NONE', #20551, 2.000000000000001776 ) ;
#21664=DIRECTION ( 'NONE',  ( -0.000000000000000000, 1.000000000000000000, -0.000000000000000000 ) ) ;
#21667=CYLINDRICAL_SURFACE ( 'NONE', #18941, 7.999999999999952038 ) ;
#21670=CARTESIAN_POINT ( 'NONE',  ( -19.99999999999998934, 134.9999999999999432, -162.9999999999999432 ) ) ;
#21674=LINE ( 'NONE', #16531, #2358 ) ;
#21675=CIRCLE ( 'NONE', #26219, 3.999999999999976019 ) ;
#21676=CARTESIAN_POINT ( 'NONE',  ( -418.0000000000000000, -125.0000000000000000, 155.0000000000000000 ) ) ;
#21677=CARTESIAN_POINT ( 'NONE',  ( -19.99999999999996092, -137.0000000000000284, 194.9999999999999716 ) ) ;
#21682=ORIENTED_EDGE ( 'NONE', *, *, #21334, .T. ) ;
#21685=VECTOR ( 'NONE', #6890, 1000.000000000000000 ) ;
#21689=VERTEX_POINT ( 'NONE', #4794 ) ;
#21691=FACE_OUTER_BOUND ( 'NONE', #22020, .T. ) ;
#21698=ORIENTED_EDGE ( 'NONE', *, *, #18967, .T. ) ;
#21699=EDGE_CURVE ( 'NONE', #32511, #9264, #29378, .T. ) ;
#21702=VECTOR ( 'NONE', #19371, 1000.000000000000000 ) ;
#21703=ORIENTED_EDGE ( 'NONE', *, *, #27209, .F. ) ;
#21706=ADVANCED_FACE ( 'NONE', ( #32738 ), #8174, .F. ) ;
#21709=VERTEX_POINT ( 'NONE', #13702 ) ;
#21712=ORIENTED_EDGE ( 'NONE', *, *, #33703, .F. ) ;
#21716=CARTESIAN_POINT ( 'NONE',  ( -500.0000000000000000, 104.9999999999999858, -155.0000000000000000 ) ) ;
#21719=CARTESIAN_POINT ( 'NONE',  ( -442.0000000000000000, -105.0000000000000142, -105.9999999999999574 ) ) ;
#21721=VECTOR ( 'NONE', #30790, 1000.000000000000000 ) ;
#21722=ORIENTED_EDGE ( 'NONE', *, *, #23305, .T. ) ;
#21724=CARTESIAN_POINT ( 'NONE',  ( -365.0000000000000000, -125.0000000000000284, 126.0000000000000000 ) ) ;
#21727=EDGE_LOOP ( 'NONE', ( #5497, #17778, #8736, #31572 ) ) ;
#21735=PLANE ( 'NONE',  #33447 ) ;
#21737=ORIENTED_EDGE ( 'NONE', *, *, #6022, .T. ) ;
#21738=ADVANCED_FACE ( 'NONE', ( #5669 ), #10857, .T. ) ;
#21743=DIRECTION ( 'NONE',  ( -1.000000000000000000, 0.000000000000000000, 0.000000000000000000 ) ) ;
#21745=ORIENTED_EDGE ( 'NONE', *, *, #9423, .T. ) ;
#21746=DIRECTION ( 'NONE',  ( 0.000000000000000000, 0.000000000000000000, -1.000000000000000000 ) ) ;
#21747=LINE ( 'NONE', #27791, #6030 ) ;
#21749=AXIS2_PLACEMENT_3D ( 'NONE', #15123, #25605, #7080 ) ;
#21752=LINE ( 'NONE', #32951, #10995 ) ;
#21753=EDGE_CURVE ( 'NONE', #16412, #6833, #16319, .T. ) ;
#21754=DIRECTION ( 'NONE',  ( -1.000000000000000000, 0.000000000000000000, -0.000000000000000000 ) ) ;
#21756=CARTESIAN_POINT ( 'NONE',  ( -19.99999999999998934, -113.0000000000000142, 155.0000000000000000 ) ) ;
#21760=DIRECTION ( 'NONE',  ( -1.000000000000000000, 0.000000000000000000, 0.000000000000000000 ) ) ;
#21763=EDGE_CURVE ( 'NONE', #15781, #11675, #29553, .T. ) ;
#21765=EDGE_LOOP ( 'NONE', ( #11997, #28920, #8636, #26119 ) ) ;
#21766=CARTESIAN_POINT ( 'NONE',  ( 12.00000000000001066, -32.99999999999997158, -175.0000000000000000 ) ) ;
#21768=ADVANCED_FACE ( 'NONE', ( #3007 ), #5145, .F. ) ;
#21770=AXIS2_PLACEMENT_3D ( 'NONE', #29866, #21838, #16355 ) ;
#21772=VECTOR ( 'NONE', #18233, 1000.000000000000000 ) ;
#21777=PLANE ( 'NONE',  #30384 ) ;
#21796=DIRECTION ( 'NONE',  ( -3.040835319149746090E-31, -1.000000000000000000, 0.000000000000000000 ) ) ;
#21804=EDGE_CURVE ( 'NONE', #34687, #25412, #30079, .T. ) ;
#21809=VERTEX_POINT ( 'NONE', #26698 ) ;
#21810=AXIS2_PLACEMENT_3D ( 'NONE', #13859, #24698, #30220 ) ;
#21813=DIRECTION ( 'NONE',  ( 1.000000000000000000, 0.000000000000000000, 5.546364386991661285E-52 ) ) ;
#21816=ORIENTED_EDGE ( 'NONE', *, *, #4331, .T. ) ;
#21817=LINE ( 'NONE', #32673, #2496 ) ;
#21820=LINE ( 'NONE', #22358, #25991 ) ;
#21823=ORIENTED_EDGE ( 'NONE', *, *, #23283, .F. ) ;
#21824=CARTESIAN_POINT ( 'NONE',  ( -499.9999999999999432, 104.9999999999999858, 162.9999999999999716 ) ) ;
#21827=VECTOR ( 'NONE', #28174, 1000.000000000000000 ) ;
#21830=DIRECTION ( 'NONE',  ( 0.000000000000000000, 2.309213040847544338E-50, 1.000000000000000000 ) ) ;
#21831=DIRECTION ( 'NONE',  ( 1.000000000000000000, 0.000000000000000000, 0.000000000000000000 ) ) ;
#21832=ORIENTED_EDGE ( 'NONE', *, *, #10737, .F. ) ;
#21835=DIRECTION ( 'NONE',  ( 0.000000000000000000, 0.000000000000000000, -1.000000000000000000 ) ) ;
#21838=DIRECTION ( 'NONE',  ( 1.000000000000000000, 0.000000000000000000, -1.232595164407831220E-32 ) ) ;
#21842=ADVANCED_FACE ( 'NONE', ( #888 ), #22241, .T. ) ;
#21846=EDGE_CURVE ( 'NONE', #10753, #5416, #14606, .T. ) ;
#21849=VECTOR ( 'NONE', #3415, 1000.000000000000000 ) ;
#21850=LINE ( 'NONE', #10657, #6905 ) ;
#21852=LINE ( 'NONE', #19373, #26832 ) ;
#21859=ORIENTED_EDGE ( 'NONE', *, *, #809, .F. ) ;
#21861=FACE_OUTER_BOUND ( 'NONE', #22738, .T. ) ;
#21862=CIRCLE ( 'NONE', #5366, 4.000000000000003553 ) ;
#21863=CARTESIAN_POINT ( 'NONE',  ( -499.9999999999999432, 108.9999999999999858, -162.9999999999999716 ) ) ;
#21869=DIRECTION ( 'NONE',  ( 0.000000000000000000, -1.000000000000000000, 6.842277657836020854E-49 ) ) ;
#21870=CIRCLE ( 'NONE', #20186, 7.999999999999986677 ) ;
#21872=ORIENTED_EDGE ( 'NONE', *, *, #19019, .T. ) ;
#21874=AXIS2_PLACEMENT_3D ( 'NONE', #17324, #1279, #33665 ) ;
#21876=ORIENTED_EDGE ( 'NONE', *, *, #20959, .T. ) ;
#21877=VECTOR ( 'NONE', #9436, 1000.000000000000000 ) ;
#21883=ORIENTED_EDGE ( 'NONE', *, *, #20256, .T. ) ;
#21885=CARTESIAN_POINT ( 'NONE',  ( 11.99999999999999645, -124.9999999999999432, -190.9999999999999432 ) ) ;
#21888=ORIENTED_EDGE ( 'NONE', *, *, #10737, .T. ) ;
#21891=EDGE_CURVE ( 'NONE', #31620, #21809, #9243, .T. ) ;
#21892=DIRECTION ( 'NONE',  ( 0.000000000000000000, 0.000000000000000000, 1.000000000000000000 ) ) ;
#21895=DIRECTION ( 'NONE',  ( 1.000000000000000000, -0.000000000000000000, -0.000000000000000000 ) ) ;
#21896=CARTESIAN_POINT ( 'NONE',  ( -365.0000000000000000, -133.0000000000000000, 126.0000000000000000 ) ) ;
#21899=AXIS2_PLACEMENT_3D ( 'NONE', #18106, #20237, #3663 ) ;
#21903=CARTESIAN_POINT ( 'NONE',  ( -19.99999999999998934, 136.9999999999999716, -155.0000000000000000 ) ) ;
#21904=CIRCLE ( 'NONE', #20217, 3.999999999999989786 ) ;
#21912=EDGE_CURVE ( 'NONE', #7236, #10395, #14648, .T. ) ;
#21915=ORIENTED_EDGE ( 'NONE', *, *, #9790, .F. ) ;
#21919=CARTESIAN_POINT ( 'NONE',  ( -70.00000000000000000, 4.559999999999908127, -172.9900000000000091 ) ) ;
#21921=EDGE_LOOP ( 'NONE', ( #25567, #23866, #5162, #6340 ) ) ;
#21923=LINE ( 'NONE', #211, #24805 ) ;
#21924=DIRECTION ( 'NONE',  ( -1.000000000000000000, 0.000000000000000000, 0.000000000000000000 ) ) ;
#21925=VECTOR ( 'NONE', #21048, 1000.000000000000000 ) ;
#21928=CARTESIAN_POINT ( 'NONE',  ( -12.00000000000001066, 124.9999999999999716, 155.0000000000000000 ) ) ;
#21929=EDGE_LOOP ( 'NONE', ( #27289, #11286, #5686, #14534 ) ) ;
#21930=CARTESIAN_POINT ( 'NONE',  ( -500.0000000000000000, -113.0000000000000000, 187.0000000000000000 ) ) ;
#21932=LINE ( 'NONE', #10902, #30567 ) ;
#21938=CARTESIAN_POINT ( 'NONE',  ( -418.0000000000000000, 145.0000000000000000, -175.0000000000000000 ) ) ;
#21940=CARTESIAN_POINT ( 'NONE',  ( -418.0000000000000000, 105.0000000000000142, 162.9999999999999716 ) ) ;
#21941=ORIENTED_EDGE ( 'NONE', *, *, #29209, .T. ) ;
#21942=LINE ( 'NONE', #19287, #3097 ) ;
#21944=LINE ( 'NONE', #30125, #28793 ) ;
#21945=MANIFOLD_SOLID_BREP ( 'Square tube 40 X 40 X 4(1)[6]', #3714 ) ;
#21946=ADVANCED_FACE ( 'NONE', ( #11217 ), #11930, .F. ) ;
#21947=VECTOR ( 'NONE', #19307, 1000.000000000000000 ) ;
#21949=ADVANCED_FACE ( 'NONE', ( #11386 ), #22773, .F. ) ;
#21957=VERTEX_POINT ( 'NONE', #9598 ) ;
#21961=EDGE_CURVE ( 'NONE', #26015, #18709, #34808, .T. ) ;
#21966=ORIENTED_EDGE ( 'NONE', *, *, #7875, .T. ) ;
#21967=CARTESIAN_POINT ( 'NONE',  ( 18.92820323027550344, -55.00000000000000711, -158.9999999999999716 ) ) ;
#21969=ADVANCED_FACE ( 'NONE', ( #4701 ), #6735, .T. ) ;
#21972=ORIENTED_EDGE ( 'NONE', *, *, #23464, .F. ) ;
#21974=CARTESIAN_POINT ( 'NONE',  ( -365.0000000000000000, 114.9999999999999574, 113.9999999999999858 ) ) ;
#21976=DIRECTION ( 'NONE',  ( 1.232595164407830946E-32, 7.496237820289040735E-63, -1.000000000000000000 ) ) ;
#21980=ADVANCED_FACE ( 'NONE', ( #29108 ), #34991, .T. ) ;
#21981=CARTESIAN_POINT ( 'NONE',  ( -499.9999999999999432, -141.0000000000000000, -187.0000000000000000 ) ) ;
#21982=CYLINDRICAL_SURFACE ( 'NONE', #7551, 7.999999999999979572 ) ;
#21984=ORIENTED_EDGE ( 'NONE', *, *, #4431, .F. ) ;
#21988=DIRECTION ( 'NONE',  ( 1.000000000000000000, 0.000000000000000000, 0.000000000000000000 ) ) ;
#21991=ORIENTED_EDGE ( 'NONE', *, *, #5891, .F. ) ;
#21993=ADVANCED_FACE ( 'NONE', ( #2398 ), #12104, .F. ) ;
#21997=ORIENTED_EDGE ( 'NONE', *, *, #18503, .F. ) ;
#21998=CIRCLE ( 'NONE', #35065, 7.999999999999979572 ) ;
#22004=CARTESIAN_POINT ( 'NONE',  ( 11.99999999999999645, 134.9999999999999432, -162.9999999999999432 ) ) ;
#22011=LINE ( 'NONE', #32853, #21345 ) ;
#22012=DIRECTION ( 'NONE',  ( -1.000000000000000000, 0.000000000000000000, 0.000000000000000000 ) ) ;
#22013=CARTESIAN_POINT ( 'NONE',  ( -365.0000000000000000, 118.9999999999999716, 113.9999999999999858 ) ) ;
#22015=ADVANCED_FACE ( 'NONE', ( #9428 ), #20284, .T. ) ;
#22016=ADVANCED_FACE ( 'NONE', ( #2059 ), #15955, .T. ) ;
#22019=LINE ( 'NONE', #127, #19276 ) ;
#22020=EDGE_LOOP ( 'NONE', ( #18158, #14392, #13311, #25672 ) ) ;
#22024=PLANE ( 'NONE',  #30264 ) ;
#22025=ORIENTED_EDGE ( 'NONE', *, *, #10314, .F. ) ;
#22034=CARTESIAN_POINT ( 'NONE',  ( -418.0000000000000568, 105.0000000000000142, 104.0000000000000142 ) ) ;
#22039=VECTOR ( 'NONE', #18813, 1000.000000000000000 ) ;
#22042=ADVANCED_FACE ( 'NONE', ( #18450 ), #15780, .F. ) ;
#22053=ORIENTED_EDGE ( 'NONE', *, *, #3603, .F. ) ;
#22058=EDGE_CURVE ( 'NONE', #1154, #20834, #30335, .T. ) ;
#22059=EDGE_CURVE ( 'NONE', #15373, #21689, #24813, .T. ) ;
#22061=ORIENTED_EDGE ( 'NONE', *, *, #9052, .F. ) ;
#22063=DIRECTION ( 'NONE',  ( -1.000000000000000000, 0.000000000000000000, 0.000000000000000000 ) ) ;
#22065=CARTESIAN_POINT ( 'NONE',  ( -499.9999999999998863, -109.0000000000000142, -162.9999999999999716 ) ) ;
#22068=ORIENTED_EDGE ( 'NONE', *, *, #6942, .F. ) ;
#22069=DIRECTION ( 'NONE',  ( -1.000000000000000000, 0.000000000000000000, 0.000000000000000000 ) ) ;
#22070=AXIS2_PLACEMENT_3D ( 'NONE', #15186, #34393, #32061 ) ;
#22072=ORIENTED_EDGE ( 'NONE', *, *, #13239, .T. ) ;
#22079=CARTESIAN_POINT ( 'NONE',  ( 11.99999999999999645, -115.0000000000000142, 159.0000000000000000 ) ) ;
#22080=( LENGTH_UNIT ( ) NAMED_UNIT ( * ) SI_UNIT ( .MILLI., .METRE. ) );
#22081=AXIS2_PLACEMENT_3D ( 'NONE', #3878, #4046, #14596 ) ;
#22088=VECTOR ( 'NONE', #22274, 1000.000000000000000 ) ;
#22091=EDGE_CURVE ( 'NONE', #26985, #31534, #29391, .T. ) ;
#22094=DIRECTION ( 'NONE',  ( 0.000000000000000000, 1.000000000000000000, 1.224646799147353207E-16 ) ) ;
#22098=EDGE_CURVE ( 'NONE', #27476, #8689, #33178, .T. ) ;
#22099=CARTESIAN_POINT ( 'NONE',  ( -365.0000000000000000, -125.0000000000000284, 168.9999999999999716 ) ) ;
#22100=DIRECTION ( 'NONE',  ( -1.232595164407830946E-32, 0.000000000000000000, -1.000000000000000000 ) ) ;
#22101=ORIENTED_EDGE ( 'NONE', *, *, #31094, .F. ) ;
#22103=CARTESIAN_POINT ( 'NONE',  ( -349.0000000000000000, 124.9999999999999432, 168.9999999999999716 ) ) ;
#22104=CARTESIAN_POINT ( 'NONE',  ( 19.99999999999998934, 144.9999999999999716, 187.0000000000000000 ) ) ;
#22105=EDGE_CURVE ( 'NONE', #8775, #16257, #5414, .T. ) ;
#22109=ORIENTED_EDGE ( 'NONE', *, *, #29776, .F. ) ;
#22111=FACE_OUTER_BOUND ( 'NONE', #7821, .T. ) ;
#22113=DIRECTION ( 'NONE',  ( 1.232595164407830946E-32, 0.000000000000000000, 1.000000000000000000 ) ) ;
#22115=LINE ( 'NONE', #3234, #33374 ) ;
#22116=( LENGTH_UNIT ( ) NAMED_UNIT ( * ) SI_UNIT ( .MILLI., .METRE. ) );
#22119=DIRECTION ( 'NONE',  ( -0.000000000000000000, 1.000000000000000000, -0.000000000000000000 ) ) ;
#22123=ORIENTED_EDGE ( 'NONE', *, *, #4109, .F. ) ;
#22126=AXIS2_PLACEMENT_3D ( 'NONE', #7495, #5001, #33733 ) ;
#22129=VECTOR ( 'NONE', #20578, 1000.000000000000000 ) ;
#22130=ORIENTED_EDGE ( 'NONE', *, *, #721, .F. ) ;
#22132=ORIENTED_EDGE ( 'NONE', *, *, #28452, .F. ) ;
#22138=VERTEX_POINT ( 'NONE', #16127 ) ;
#22140=CARTESIAN_POINT ( 'NONE',  ( -442.0000000000000000, -105.0000000000000142, 100.0000000000000000 ) ) ;
#22142=VERTEX_POINT ( 'NONE', #13978 ) ;
#22144=CARTESIAN_POINT ( 'NONE',  ( -12.00000000000001066, 112.9999999999999574, -175.0000000000000284 ) ) ;
#22147=LINE ( 'NONE', #11465, #6188 ) ;
#22148=DIRECTION ( 'NONE',  ( 0.000000000000000000, 1.000000000000000000, 0.000000000000000000 ) ) ;
#22150=DIRECTION ( 'NONE',  ( 0.000000000000000000, 0.000000000000000000, -1.000000000000000000 ) ) ;
#22152=EDGE_CURVE ( 'NONE', #11554, #10950, #16306, .T. ) ;
#22159=PLANE ( 'NONE',  #5804 ) ;
#22160=ORIENTED_EDGE ( 'NONE', *, *, #32103, .T. ) ;
#22164=ADVANCED_FACE ( 'NONE', ( #24280 ), #21982, .T. ) ;
#22165=ORIENTED_EDGE ( 'NONE', *, *, #25188, .T. ) ;
#22167=CYLINDRICAL_SURFACE ( 'NONE', #34795, 3.999999999999976019 ) ;
#22168=FACE_OUTER_BOUND ( 'NONE', #333, .T. ) ;
#22169=ORIENTED_EDGE ( 'NONE', *, *, #22676, .T. ) ;
#22170=ORIENTED_EDGE ( 'NONE', *, *, #4162, .T. ) ;
#22171=ADVANCED_FACE ( 'NONE', ( #8616 ), #19495, .T. ) ;
#22173=EDGE_LOOP ( 'NONE', ( #20309, #14722, #11139, #31642 ) ) ;
#22177=ORIENTED_EDGE ( 'NONE', *, *, #14218, .F. ) ;
#22179=VECTOR ( 'NONE', #6046, 1000.000000000000000 ) ;
#22180=CARTESIAN_POINT ( 'NONE',  ( -12.00000000000001066, 144.9999999999999716, 159.0000000000000000 ) ) ;
#22181=CARTESIAN_POINT ( 'NONE',  ( 12.00000000000001066, -64.99999999999997158, -175.0000000000000000 ) ) ;
#22190=EDGE_CURVE ( 'NONE', #31755, #17164, #23487, .T. ) ;
#22194=VERTEX_POINT ( 'NONE', #3970 ) ;
#22195=CARTESIAN_POINT ( 'NONE',  ( 11.99999999999999645, 124.9999999999999716, 159.0000000000000000 ) ) ;
#22196=DIRECTION ( 'NONE',  ( 0.000000000000000000, 1.000000000000000000, 1.224646799147353207E-16 ) ) ;
#22197=DIRECTION ( 'NONE',  ( 1.000000000000000000, 3.040835319149746090E-31, 1.232595164407830946E-32 ) ) ;
#22198=ORIENTED_EDGE ( 'NONE', *, *, #9196, .F. ) ;
#22199=CARTESIAN_POINT ( 'NONE',  ( -442.0000000000000000, -105.0000000000000142, -77.99999999999997158 ) ) ;
#22200=ORIENTED_EDGE ( 'NONE', *, *, #17386, .T. ) ;
#22203=PLANE ( 'NONE',  #26811 ) ;
#22204=VECTOR ( 'NONE', #31117, 1000.000000000000000 ) ;
#22205=VERTEX_POINT ( 'NONE', #12195 ) ;
#22207=LINE ( 'NONE', #33052, #6556 ) ;
#22208=DIRECTION ( 'NONE',  ( -0.000000000000000000, 1.000000000000000000, -0.000000000000000000 ) ) ;
#22209=EDGE_CURVE ( 'NONE', #27507, #18790, #5288, .T. ) ;
#22216=ORIENTED_EDGE ( 'NONE', *, *, #27878, .T. ) ;
#22221=CARTESIAN_POINT ( 'NONE',  ( -363.0000000000000000, -125.0000000000000284, 181.0000000000000000 ) ) ;
#22224=ORIENTED_EDGE ( 'NONE', *, *, #15512, .F. ) ;
#22225=ORIENTED_EDGE ( 'NONE', *, *, #34523, .F. ) ;
#22227=VECTOR ( 'NONE', #7369, 1000.000000000000000 ) ;
#22231=DIRECTION ( 'NONE',  ( 0.000000000000000000, 0.000000000000000000, 1.000000000000000000 ) ) ;
#22232=EDGE_CURVE ( 'NONE', #32595, #16498, #33147, .T. ) ;
#22238=DIRECTION ( 'NONE',  ( 0.000000000000000000, 0.000000000000000000, -1.000000000000000000 ) ) ;
#22241=PLANE ( 'NONE',  #8372 ) ;
#22247=AXIS2_PLACEMENT_3D ( 'NONE', #3763, #17668, #31177 ) ;
#22248=DIRECTION ( 'NONE',  ( 0.000000000000000000, 0.000000000000000000, 1.000000000000000000 ) ) ;
#22249=CARTESIAN_POINT ( 'NONE',  ( -499.9999999999999432, -137.0000000000000000, -190.9999999999999716 ) ) ;
#22250=FACE_BOUND ( 'NONE', #33364, .T. ) ;
#22251=CYLINDRICAL_SURFACE ( 'NONE', #33878, 3.999999999999976019 ) ;
#22252=CARTESIAN_POINT ( 'NONE',  ( -445.9999999999999432, -112.9999999999999858, -174.9999999999999716 ) ) ;
#22253=CARTESIAN_POINT ( 'NONE',  ( -20.00000000000007461, 144.9999999999999716, 187.0000000000000000 ) ) ;
#22254=AXIS2_PLACEMENT_3D ( 'NONE', #26203, #4137, #25866 ) ;
#22262=EDGE_LOOP ( 'NONE', ( #16395, #29188, #17613, #28904 ) ) ;
#22263=CARTESIAN_POINT ( 'NONE',  ( -361.0000000000000000, -135.0000000000000000, 113.9999999999999858 ) ) ;
#22266=AXIS2_PLACEMENT_3D ( 'NONE', #9208, #33583, #11717 ) ;
#22267=ORIENTED_EDGE ( 'NONE', *, *, #9714, .T. ) ;
#22268=VECTOR ( 'NONE', #29827, 1000.000000000000000 ) ;
#22269=AXIS2_PLACEMENT_3D ( 'NONE', #5989, #19545, #33043 ) ;
#22270=LINE ( 'NONE', #2691, #10522 ) ;
#22274=DIRECTION ( 'NONE',  ( 0.000000000000000000, 2.465190328815661892E-32, 1.000000000000000000 ) ) ;
#22276=ORIENTED_EDGE ( 'NONE', *, *, #18078, .T. ) ;
#22277=CARTESIAN_POINT ( 'NONE',  ( -500.0000000000000000, -137.0000000000000000, 155.0000000000000000 ) ) ;
#22279=CARTESIAN_POINT ( 'NONE',  ( 19.99999999999998934, 144.9999999999999716, 187.0000000000000000 ) ) ;
#22280=DIRECTION ( 'NONE',  ( 0.000000000000000000, 0.000000000000000000, -1.000000000000000000 ) ) ;
#22283=LINE ( 'NONE', #33314, #16967 ) ;
#22285=CARTESIAN_POINT ( 'NONE',  ( 19.99999999999998934, 75.55999999999990280, 177.7400000000000091 ) ) ;
#22287=ORIENTED_EDGE ( 'NONE', *, *, #16945, .F. ) ;
#22288=CARTESIAN_POINT ( 'NONE',  ( -418.0000000000000000, -105.0000000000000142, 135.9999999999999716 ) ) ;
#22289=PLANE ( 'NONE',  #22247 ) ;
#22291=VECTOR ( 'NONE', #4579, 1000.000000000000000 ) ;
#22292=DIRECTION ( 'NONE',  ( 0.000000000000000000, 0.000000000000000000, -1.000000000000000000 ) ) ;
#22295=AXIS2_PLACEMENT_3D ( 'NONE', #29480, #13290, #16317 ) ;
#22296=CARTESIAN_POINT ( 'NONE',  ( -418.0000000000000000, 109.0000000000000142, -155.0000000000000000 ) ) ;
#22297=ORIENTED_EDGE ( 'NONE', *, *, #9526, .F. ) ;
#22300=DIRECTION ( 'NONE',  ( 0.000000000000000000, 0.000000000000000000, -1.000000000000000000 ) ) ;
#22306=ORIENTED_EDGE ( 'NONE', *, *, #13583, .F. ) ;
#22313=CARTESIAN_POINT ( 'NONE',  ( 12.00000000000001066, -134.9999999999999716, 162.9999999999999716 ) ) ;
#22314=AXIS2_PLACEMENT_3D ( 'NONE', #2666, #13535, #24374 ) ;
#22316=ORIENTED_EDGE ( 'NONE', *, *, #4467, .F. ) ;
#22318=ORIENTED_EDGE ( 'NONE', *, *, #19936, .T. ) ;
#22329=DIRECTION ( 'NONE',  ( 1.000000000000000000, 0.000000000000000000, 0.000000000000000000 ) ) ;
#22330=DIRECTION ( 'NONE',  ( 0.000000000000000000, 0.000000000000000000, -1.000000000000000000 ) ) ;
#22333=ORIENTED_EDGE ( 'NONE', *, *, #3028, .T. ) ;
#22335=DIRECTION ( 'NONE',  ( 0.000000000000000000, -1.000000000000000000, 3.421138828918010427E-49 ) ) ;
#22338=AXIS2_PLACEMENT_3D ( 'NONE', #18630, #23602, #20933 ) ;
#22340=CIRCLE ( 'NONE', #17179, 4.000000000000003553 ) ;
#22346=EDGE_LOOP ( 'NONE', ( #15389, #11312, #22198, #22705 ) ) ;
#22347=EDGE_LOOP ( 'NONE', ( #22442, #14397, #16859, #228 ) ) ;
#22349=EDGE_CURVE ( 'NONE', #20441, #34661, #9847, .T. ) ;
#22350=VERTEX_POINT ( 'NONE', #7163 ) ;
#22351=CARTESIAN_POINT ( 'NONE',  ( 11.99999999999999645, -145.0000000000000000, 159.0000000000000000 ) ) ;
#22352=CARTESIAN_POINT ( 'NONE',  ( -418.0000000000000000, -105.0000000000000142, -174.9999999999999716 ) ) ;
#22353=EDGE_LOOP ( 'NONE', ( #27254, #32526, #4636, #28688 ) ) ;
#22358=CARTESIAN_POINT ( 'NONE',  ( -11.99999999999998224, -134.9999999999999716, 194.9999999999999716 ) ) ;
#22359=PLANE ( 'NONE',  #22771 ) ;
#22361=ORIENTED_EDGE ( 'NONE', *, *, #16645, .T. ) ;
#22364=CARTESIAN_POINT ( 'NONE',  ( -442.0000000000000000, 141.0000000000000000, -155.0000000000000000 ) ) ;
#22372=FACE_OUTER_BOUND ( 'NONE', #25191, .T. ) ;
#22374=CARTESIAN_POINT ( 'NONE',  ( -442.0000000000000000, -105.0000000000000142, 107.9999999999999858 ) ) ;
#22375=ORIENTED_EDGE ( 'NONE', *, *, #553, .T. ) ;
#22380=LINE ( 'NONE', #22564, #29609 ) ;
#22381=VECTOR ( 'NONE', #16718, 1000.000000000000000 ) ;
#22383=LINE ( 'NONE', #31105, #13177 ) ;
#22385=DIRECTION ( 'NONE',  ( 1.000000000000000000, 0.000000000000000000, 0.000000000000000000 ) ) ;
#22386=ADVANCED_FACE ( 'NONE', ( #18229 ), #10025, .F. ) ;
#22390=EDGE_CURVE ( 'NONE', #32869, #15141, #2014, .T. ) ;
#22391=EDGE_CURVE ( 'NONE', #30770, #23261, #4489, .T. ) ;
#22393=VECTOR ( 'NONE', #12537, 1000.000000000000000 ) ;
#22398=CARTESIAN_POINT ( 'NONE',  ( -499.9999999999999432, 136.9999999999999432, 187.0000000000000000 ) ) ;
#22402=ORIENTED_EDGE ( 'NONE', *, *, #6784, .T. ) ;
#22404=EDGE_CURVE ( 'NONE', #8601, #28875, #1891, .T. ) ;
#22409=VERTEX_POINT ( 'NONE', #18065 ) ;
#22412=ORIENTED_EDGE ( 'NONE', *, *, #4135, .F. ) ;
#22414=LINE ( 'NONE', #30603, #29992 ) ;
#22415=PLANE ( 'NONE',  #18291 ) ;
#22417=CARTESIAN_POINT ( 'NONE',  ( -12.00000000000001066, 124.9999999999999716, 194.9999999999999716 ) ) ;
#22419=EDGE_CURVE ( 'NONE', #20279, #25692, #16121, .T. ) ;
#22420=DIRECTION ( 'NONE',  ( 0.000000000000000000, 0.000000000000000000, 1.000000000000000000 ) ) ;
#22421=VECTOR ( 'NONE', #580, 1000.000000000000000 ) ;
#22425=CARTESIAN_POINT ( 'NONE',  ( 19.99999999999998934, -137.0000000000000000, -155.0000000000000284 ) ) ;
#22426=CARTESIAN_POINT ( 'NONE',  ( -442.0000000000000000, -112.9999999999999858, -155.0000000000000000 ) ) ;
#22428=EDGE_CURVE ( 'NONE', #8431, #13630, #1834, .T. ) ;
#22432=LINE ( 'NONE', #22253, #21877 ) ;
#22433=LINE ( 'NONE', #6037, #16101 ) ;
#22434=VERTEX_POINT ( 'NONE', #15549 ) ;
#22436=ORIENTED_EDGE ( 'NONE', *, *, #17400, .F. ) ;
#22439=EDGE_LOOP ( 'NONE', ( #19826, #32800, #27753, #18336 ) ) ;
#22441=VERTEX_POINT ( 'NONE', #12890 ) ;
#22442=ORIENTED_EDGE ( 'NONE', *, *, #15476, .F. ) ;
#22447=VECTOR ( 'NONE', #25792, 1000.000000000000000 ) ;
#22449=DIRECTION ( 'NONE',  ( 0.000000000000000000, -1.000000000000000000, 1.131431318426415506E-52 ) ) ;
#22461=CARTESIAN_POINT ( 'NONE',  ( -12.00000000000003908, -134.9999999999999716, -154.9999999999999716 ) ) ;
#22462=CARTESIAN_POINT ( 'NONE',  ( -355.0000000000000000, -119.0000000000000000, 128.0000000000000000 ) ) ;
#22463=ADVANCED_FACE ( 'NONE', ( #10201 ), #2353, .F. ) ;
#22466=EDGE_LOOP ( 'NONE', ( #21484, #13592, #25296, #17755 ) ) ;
#22467=CIRCLE ( 'NONE', #19631, 2.000000000000001776 ) ;
#22468=DIRECTION ( 'NONE',  ( 0.000000000000000000, 1.000000000000000000, 2.465190328815662439E-32 ) ) ;
#22470=FACE_OUTER_BOUND ( 'NONE', #31923, .T. ) ;
#22475=UNCERTAINTY_MEASURE_WITH_UNIT (LENGTH_MEASURE( 1.000000000000000082E-05 ), #21468, 'distance_accuracy_value', 'NONE');
#22476=CYLINDRICAL_SURFACE ( 'NONE', #24656, 3.999999999999976019 ) ;
#22477=ADVANCED_FACE ( 'NONE', ( #34946 ), #21231, .T. ) ;
#22479=DIRECTION ( 'NONE',  ( 1.000000000000000000, 3.469446951953834515E-18, 0.000000000000000000 ) ) ;
#22482=CLOSED_SHELL ( 'NONE', ( #5129, #14540, #21607, #9372, #13104, #21336, #31692, #21949, #6615, #17672, #14323, #27357, #12110, #10223, #25579, #4543, #22667, #31696 ) ) ;
#22484=ORIENTED_EDGE ( 'NONE', *, *, #11004, .T. ) ;
#22487=DIRECTION ( 'NONE',  ( 1.000000000000000000, 0.000000000000000000, 0.000000000000000000 ) ) ;
#22490=EDGE_CURVE ( 'NONE', #27476, #19038, #20536, .T. ) ;
#22492=VECTOR ( 'NONE', #10558, 1000.000000000000000 ) ;
#22493=EDGE_LOOP ( 'NONE', ( #2657, #3174, #25129, #4969 ) ) ;
#22494=LINE ( 'NONE', #33871, #34556 ) ;
#22495=CARTESIAN_POINT ( 'NONE',  ( 15.99999999999998579, -137.0000000000000000, 155.0000000000000000 ) ) ;
#22498=LINE ( 'NONE', #30319, #21947 ) ;
#22502=CARTESIAN_POINT ( 'NONE',  ( -20.00000000000007461, 136.9999999999999432, -162.9999999999999716 ) ) ;
#22504=FACE_BOUND ( 'NONE', #19046, .T. ) ;
#22506=EDGE_CURVE ( 'NONE', #23786, #33325, #19109, .T. ) ;
#22508=EDGE_CURVE ( 'NONE', #33799, #8677, #21752, .T. ) ;
#22509=CARTESIAN_POINT ( 'NONE',  ( -355.0000000000000000, 118.9999999999999716, 130.0000000000000000 ) ) ;
#22510=ORIENTED_EDGE ( 'NONE', *, *, #28807, .F. ) ;
#22519=ORIENTED_EDGE ( 'NONE', *, *, #5338, .F. ) ;
#22521=CARTESIAN_POINT ( 'NONE',  ( -410.0000000000000568, 113.0000000000000000, 154.9999999999999716 ) ) ;
#22522=CARTESIAN_POINT ( 'NONE',  ( -15.99999999999998579, 4.559999999999909015, -168.2400000000000091 ) ) ;
#22528=VECTOR ( 'NONE', #13025, 1000.000000000000000 ) ;
#22530=AXIS2_PLACEMENT_3D ( 'NONE', #7359, #18606, #5045 ) ;
#22531=EDGE_LOOP ( 'NONE', ( #3700, #2736, #11388, #17389 ) ) ;
#22532=LINE ( 'NONE', #28572, #17388 ) ;
#22534=ORIENTED_EDGE ( 'NONE', *, *, #26350, .T. ) ;
#22535=MANIFOLD_SOLID_BREP ( 'Boss-Extrude6[1]', #33827 ) ;
#22538=DIRECTION ( 'NONE',  ( -0.000000000000000000, 1.000000000000000000, -0.000000000000000000 ) ) ;
#22539=CARTESIAN_POINT ( 'NONE',  ( -449.9999999999999432, -112.9999999999999858, -155.0000000000000000 ) ) ;
#22542=ORIENTED_EDGE ( 'NONE', *, *, #4331, .F. ) ;
#22545=CARTESIAN_POINT ( 'NONE',  ( -499.9999999999999432, -113.0000000000000000, -194.9999999999999716 ) ) ;
#22547=CIRCLE ( 'NONE', #28235, 4.000000000000003553 ) ;
#22548=EDGE_CURVE ( 'NONE', #1095, #28119, #13931, .T. ) ;
#22549=DIRECTION ( 'NONE',  ( -1.000000000000000000, 0.000000000000000000, 1.232595164407831220E-32 ) ) ;
#22552=ADVANCED_FACE ( 'NONE', ( #3236 ), #14110, .T. ) ;
#22555=ADVANCED_FACE ( 'NONE', ( #32259 ), #7877, .F. ) ;
#22556=VECTOR ( 'NONE', #21240, 1000.000000000000000 ) ;
#22557=PLANE ( 'NONE',  #2607 ) ;
#22559=CARTESIAN_POINT ( 'NONE',  ( 11.99999999999999645, 144.9999999999999716, -162.9999999999999432 ) ) ;
#22560=ORIENTED_EDGE ( 'NONE', *, *, #8059, .T. ) ;
#22561=CARTESIAN_POINT ( 'NONE',  ( -500.0000000000000000, -104.9999999999999858, -194.9999999999999716 ) ) ;
#22564=CARTESIAN_POINT ( 'NONE',  ( 19.99999999999998934, 144.9999999999999716, -186.9999999999999432 ) ) ;
#22565=CIRCLE ( 'NONE', #26534, 4.000000000000003553 ) ;
#22566=EDGE_CURVE ( 'NONE', #21537, #30882, #6322, .T. ) ;
#22567=EDGE_CURVE ( 'NONE', #13666, #6283, #26222, .T. ) ;
#22572=DIRECTION ( 'NONE',  ( 0.000000000000000000, -1.000000000000000000, -1.224646799147353207E-16 ) ) ;
#22577=DIRECTION ( 'NONE',  ( -2.891205793294675368E-16, 0.000000000000000000, -1.000000000000000000 ) ) ;
#22581=VERTEX_POINT ( 'NONE', #14990 ) ;
#22584=LINE ( 'NONE', #24883, #29472 ) ;
#22585=( GEOMETRIC_REPRESENTATION_CONTEXT ( 3 ) GLOBAL_UNCERTAINTY_ASSIGNED_CONTEXT ( ( #8940 ) ) GLOBAL_UNIT_ASSIGNED_CONTEXT ( ( #8886, #709, #19931 ) ) REPRESENTATION_CONTEXT ( 'NONE', 'WORKASPACE' ) );
#22588=CIRCLE ( 'NONE', #7218, 7.999999999999979572 ) ;
#22590=DIRECTION ( 'NONE',  ( 0.000000000000000000, 1.310824597558155437E-49, 1.000000000000000000 ) ) ;
#22591=ORIENTED_EDGE ( 'NONE', *, *, #5243, .T. ) ;
#22593=DIRECTION ( 'NONE',  ( 0.000000000000000000, -1.000000000000000000, -2.465190328815662439E-32 ) ) ;
#22595=EDGE_CURVE ( 'NONE', #6108, #10763, #4095, .T. ) ;
#22596=DIRECTION ( 'NONE',  ( 0.000000000000000000, -1.000000000000000000, 6.123233995736766036E-17 ) ) ;
#22599=VERTEX_POINT ( 'NONE', #17322 ) ;
#22603=ADVANCED_FACE ( 'NONE', ( #33847 ), #6424, .T. ) ;
#22604=ADVANCED_FACE ( 'NONE', ( #3407 ), #22289, .T. ) ;
#22605=LINE ( 'NONE', #5670, #21193 ) ;
#22606=ORIENTED_EDGE ( 'NONE', *, *, #12230, .F. ) ;
#22609=LINE ( 'NONE', #25257, #18973 ) ;
#22610=LINE ( 'NONE', #9722, #3761 ) ;
#22611=CIRCLE ( 'NONE', #14071, 4.000000000000003553 ) ;
#22614=FACE_BOUND ( 'NONE', #32458, .T. ) ;
#22615=VERTEX_POINT ( 'NONE', #33135 ) ;
#22617=VECTOR ( 'NONE', #13927, 1000.000000000000000 ) ;
#22621=VERTEX_POINT ( 'NONE', #19633 ) ;
#22628=EDGE_LOOP ( 'NONE', ( #16192, #16188, #18731, #29928 ) ) ;
#22631=DIRECTION ( 'NONE',  ( -0.000000000000000000, 1.000000000000000000, -0.000000000000000000 ) ) ;
#22634=ORIENTED_EDGE ( 'NONE', *, *, #14142, .F. ) ;
#22635=ORIENTED_EDGE ( 'NONE', *, *, #12162, .F. ) ;
#22636=LINE ( 'NONE', #19962, #4323 ) ;
#22638=CARTESIAN_POINT ( 'NONE',  ( -12.00000000000001066, -56.99999999999997868, -154.9999999999999716 ) ) ;
#22639=DIRECTION ( 'NONE',  ( 1.000000000000000000, 0.000000000000000000, 0.000000000000000000 ) ) ;
#22642=CIRCLE ( 'NONE', #26613, 3.999999999999976019 ) ;
#22644=DIRECTION ( 'NONE',  ( -0.000000000000000000, -1.000000000000000000, -0.000000000000000000 ) ) ;
#22648=VERTEX_POINT ( 'NONE', #19974 ) ;
#22649=LINE ( 'NONE', #28153, #19195 ) ;
#22656=DIRECTION ( 'NONE',  ( -1.000000000000000000, 0.000000000000000000, 0.000000000000000000 ) ) ;
#22664=ORIENTED_EDGE ( 'NONE', *, *, #20612, .F. ) ;
#22667=ADVANCED_FACE ( 'NONE', ( #17502, #3927 ), #4977, .T. ) ;
#22669=CARTESIAN_POINT ( 'NONE',  ( 11.99999999999999645, -105.0000000000000142, 174.9999999999999432 ) ) ;
#22672=CARTESIAN_POINT ( 'NONE',  ( -430.0000000000000000, 134.9999999999999716, 113.9999999999999858 ) ) ;
#22674=AXIS2_PLACEMENT_3D ( 'NONE', #12056, #19887, #1181 ) ;
#22676=EDGE_CURVE ( 'NONE', #18132, #22985, #15164, .T. ) ;
#22678=FACE_OUTER_BOUND ( 'NONE', #6309, .T. ) ;
#22685=DIRECTION ( 'NONE',  ( 1.000000000000000000, 0.000000000000000000, 0.000000000000000000 ) ) ;
#22690=VECTOR ( 'NONE', #30726, 1000.000000000000000 ) ;
#22692=ORIENTED_EDGE ( 'NONE', *, *, #21057, .T. ) ;
#22696=DIRECTION ( 'NONE',  ( 0.000000000000000000, 0.000000000000000000, 1.000000000000000000 ) ) ;
#22700=ORIENTED_EDGE ( 'NONE', *, *, #22349, .F. ) ;
#22704=VECTOR ( 'NONE', #1535, 1000.000000000000000 ) ;
#22705=ORIENTED_EDGE ( 'NONE', *, *, #29800, .T. ) ;
#22706=FACE_OUTER_BOUND ( 'NONE', #8903, .T. ) ;
#22710=ADVANCED_FACE ( 'NONE', ( #7294 ), #18361, .F. ) ;
#22711=EDGE_CURVE ( 'NONE', #24869, #20130, #33025, .T. ) ;
#22712=CIRCLE ( 'NONE', #10760, 3.999999999999976019 ) ;
#22714=DIRECTION ( 'NONE',  ( 0.000000000000000000, -1.224646799147353207E-16, 1.000000000000000000 ) ) ;
#22717=MANIFOLD_SOLID_BREP ( 'Square tube 40 X 40 X 4(1)[11]', #2012 ) ;
#22720=DIRECTION ( 'NONE',  ( -1.000000000000000000, 0.000000000000000000, 1.232595164407831220E-32 ) ) ;
#22721=CARTESIAN_POINT ( 'NONE',  ( -499.9999999999999432, -137.0000000000000000, -194.9999999999999716 ) ) ;
#22722=EDGE_LOOP ( 'NONE', ( #22560, #5276, #13874, #29498 ) ) ;
#22723=ORIENTED_EDGE ( 'NONE', *, *, #29160, .F. ) ;
#22726=CARTESIAN_POINT ( 'NONE',  ( -365.0000000000000000, 124.9999999999999432, 181.0000000000000000 ) ) ;
#22732=ORIENTED_EDGE ( 'NONE', *, *, #1689, .F. ) ;
#22734=LINE ( 'NONE', #33570, #14331 ) ;
#22737=CARTESIAN_POINT ( 'NONE',  ( -345.0000000000000000, -125.0000000000000284, 181.0000000000000000 ) ) ;
#22738=EDGE_LOOP ( 'NONE', ( #33536, #10174, #15496, #15282 ) ) ;
#22741=CARTESIAN_POINT ( 'NONE',  ( -442.0000000000000000, 105.0000000000000000, 139.9999999999999716 ) ) ;
#22745=EDGE_CURVE ( 'NONE', #8531, #25754, #34014, .T. ) ;
#22754=( NAMED_UNIT ( * ) PLANE_ANGLE_UNIT ( ) SI_UNIT ( $, .RADIAN. ) );
#22755=CARTESIAN_POINT ( 'NONE',  ( -430.0000000000000000, 132.9999999999999716, 126.0000000000000000 ) ) ;
#22759=EDGE_LOOP ( 'NONE', ( #27310, #16822, #21567, #22200 ) ) ;
#22761=DIRECTION ( 'NONE',  ( -1.000000000000000000, 0.000000000000000000, -5.546364386991661285E-52 ) ) ;
#22763=DIRECTION ( 'NONE',  ( 1.000000000000000000, 3.040835319149746528E-31, 1.232595164407830946E-32 ) ) ;
#22765=DIRECTION ( 'NONE',  ( 0.000000000000000000, 1.131431318426415506E-52, 1.000000000000000000 ) ) ;
#22770=ORIENTED_EDGE ( 'NONE', *, *, #27125, .F. ) ;
#22771=AXIS2_PLACEMENT_3D ( 'NONE', #31077, #17399, #27688 ) ;
#22772=EDGE_LOOP ( 'NONE', ( #4913, #7279, #22375, #21320 ) ) ;
#22773=CYLINDRICAL_SURFACE ( 'NONE', #7216, 2.000000000000001776 ) ;
#22777=DIRECTION ( 'NONE',  ( -3.469446951953832974E-18, -1.000000000000000000, -7.888609052210116302E-31 ) ) ;
#22779=VECTOR ( 'NONE', #19080, 1000.000000000000000 ) ;
#22781=CARTESIAN_POINT ( 'NONE',  ( -442.0000000000000000, -105.0000000000000142, -109.9999999999999574 ) ) ;
#22782=ADVANCED_FACE ( 'NONE', ( #20670 ), #13708, .F. ) ;
#22783=ORIENTED_EDGE ( 'NONE', *, *, #22798, .F. ) ;
#22787=ADVANCED_FACE ( 'NONE', ( #35080 ), #8007, .F. ) ;
#22791=LINE ( 'NONE', #33820, #10721 ) ;
#22794=EDGE_CURVE ( 'NONE', #18049, #30159, #2333, .T. ) ;
#22795=ORIENTED_EDGE ( 'NONE', *, *, #2520, .T. ) ;
#22798=EDGE_CURVE ( 'NONE', #11163, #32869, #34176, .T. ) ;
#22807=CARTESIAN_POINT ( 'NONE',  ( -15.99999999999998579, -145.0000000000000000, 187.0000000000000000 ) ) ;
#22809=VERTEX_POINT ( 'NONE', #4 ) ;
#22810=DIRECTION ( 'NONE',  ( 0.000000000000000000, 1.224646799147353207E-16, -1.000000000000000000 ) ) ;
#22812=ORIENTED_EDGE ( 'NONE', *, *, #34790, .F. ) ;
#22816=AXIS2_PLACEMENT_3D ( 'NONE', #12557, #18093, #26593 ) ;
#22817=CARTESIAN_POINT ( 'NONE',  ( -12.00000000000001066, -124.9999999999999432, -154.9999999999999716 ) ) ;
#22818=PLANE ( 'NONE',  #21874 ) ;
#22820=DIRECTION ( 'NONE',  ( 0.000000000000000000, 0.000000000000000000, 1.000000000000000000 ) ) ;
#22822=ORIENTED_EDGE ( 'NONE', *, *, #27633, .T. ) ;
#22823=CARTESIAN_POINT ( 'NONE',  ( -15.99999999999998579, 4.559999999999908127, 168.2400000000000091 ) ) ;
#22824=( LENGTH_UNIT ( ) NAMED_UNIT ( * ) SI_UNIT ( .MILLI., .METRE. ) );
#22829=VECTOR ( 'NONE', #19595, 1000.000000000000000 ) ;
#22830=AXIS2_PLACEMENT_3D ( 'NONE', #35005, #18984, #5595 ) ;
#22832=EDGE_LOOP ( 'NONE', ( #63, #28843, #34293, #25905 ) ) ;
#22833=EDGE_CURVE ( 'NONE', #16547, #14949, #19464, .T. ) ;
#22835=ORIENTED_EDGE ( 'NONE', *, *, #8334, .F. ) ;
#22838=ORIENTED_EDGE ( 'NONE', *, *, #6889, .T. ) ;
#22841=VERTEX_POINT ( 'NONE', #32387 ) ;
#22843=DIRECTION ( 'NONE',  ( 0.000000000000000000, 1.000000000000000000, 1.131431318426415506E-52 ) ) ;
#22845=EDGE_LOOP ( 'NONE', ( #19971, #26481, #26792, #26616 ) ) ;
#22847=CARTESIAN_POINT ( 'NONE',  ( -442.0000000000000000, 105.0000000000000142, 162.9999999999999716 ) ) ;
#22849=LINE ( 'NONE', #1311, #6782 ) ;
#22850=DIRECTION ( 'NONE',  ( -0.000000000000000000, 6.123233995736766036E-17, 1.000000000000000000 ) ) ;
#22852=CARTESIAN_POINT ( 'NONE',  ( -365.0000000000000000, -125.0000000000000284, 181.0000000000000000 ) ) ;
#22857=DIRECTION ( 'NONE',  ( 0.000000000000000000, -2.465190328815661892E-32, -1.000000000000000000 ) ) ;
#22858=ORIENTED_EDGE ( 'NONE', *, *, #25915, .T. ) ;
#22871=VERTEX_POINT ( 'NONE', #8181 ) ;
#22873=CARTESIAN_POINT ( 'NONE',  ( -410.0000000000000568, -104.9999999999999716, -162.9999999999999716 ) ) ;
#22876=ORIENTED_EDGE ( 'NONE', *, *, #1438, .T. ) ;
#22882=STYLED_ITEM('',(#35254),#24685);
#22883=ORIENTED_EDGE ( 'NONE', *, *, #28209, .F. ) ;
#22887=DIRECTION ( 'NONE',  ( 0.000000000000000000, 1.000000000000000000, 5.053935297177146739E-49 ) ) ;
#22888=PLANE ( 'NONE',  #22126 ) ;
#22889=LINE ( 'NONE', #20051, #14591 ) ;
#22893=DIRECTION ( 'NONE',  ( -0.000000000000000000, 1.000000000000000000, -0.000000000000000000 ) ) ;
#22895=FACE_OUTER_BOUND ( 'NONE', #14360, .T. ) ;
#22896=DIRECTION ( 'NONE',  ( 1.000000000000000000, 3.469446951953834515E-18, 0.000000000000000000 ) ) ;
#22898=DIRECTION ( 'NONE',  ( -1.000000000000000000, 0.000000000000000000, 0.000000000000000000 ) ) ;
#22901=EDGE_CURVE ( 'NONE', #28106, #24475, #3014, .T. ) ;
#22903=FACE_OUTER_BOUND ( 'NONE', #10512, .T. ) ;
#22905=DIRECTION ( 'NONE',  ( -1.848892746611746419E-32, -6.842277657836020854E-49, 1.000000000000000000 ) ) ;
#22907=EDGE_CURVE ( 'NONE', #9255, #24623, #29557, .T. ) ;
#22912=LINE ( 'NONE', #33763, #14507 ) ;
#22913=CARTESIAN_POINT ( 'NONE',  ( -449.9999999999999432, 105.0000000000000142, 107.9999999999999858 ) ) ;
#22914=VERTEX_POINT ( 'NONE', #22954 ) ;
#22915=DIRECTION ( 'NONE',  ( -1.000000000000000000, 0.000000000000000000, 0.000000000000000000 ) ) ;
#22918=EDGE_LOOP ( 'NONE', ( #34396, #22929, #20934, #25668 ) ) ;
#22923=DIRECTION ( 'NONE',  ( 0.000000000000000000, -6.123233995736766036E-17, -1.000000000000000000 ) ) ;
#22925=CARTESIAN_POINT ( 'NONE',  ( 19.99999999999996092, -145.0000000000000000, 162.9999999999999716 ) ) ;
#22926=AXIS2_PLACEMENT_3D ( 'NONE', #27183, #13842, #11354 ) ;
#22927=CARTESIAN_POINT ( 'NONE',  ( -365.0000000000000000, 134.9999999999999716, 113.9999999999999858 ) ) ;
#22929=ORIENTED_EDGE ( 'NONE', *, *, #30669, .T. ) ;
#22930=EDGE_LOOP ( 'NONE', ( #15973, #22591, #23590, #28257 ) ) ;
#22931=VECTOR ( 'NONE', #33663, 1000.000000000000000 ) ;
#22937=DIRECTION ( 'NONE',  ( 0.000000000000000000, 1.000000000000000000, 1.224646799147353207E-16 ) ) ;
#22940=MANIFOLD_SOLID_BREP ( 'Boss-Extrude4[1]', #13220 ) ;
#22943=DIRECTION ( 'NONE',  ( -1.000000000000000000, 0.000000000000000000, 0.000000000000000000 ) ) ;
#22945=EDGE_CURVE ( 'NONE', #34809, #1848, #678, .T. ) ;
#22946=ORIENTED_EDGE ( 'NONE', *, *, #15825, .F. ) ;
#22947=DIRECTION ( 'NONE',  ( -0.000000000000000000, -0.000000000000000000, -1.000000000000000000 ) ) ;
#22948=EDGE_CURVE ( 'NONE', #20300, #1296, #20289, .T. ) ;
#22949=AXIS2_PLACEMENT_3D ( 'NONE', #17252, #27372, #11196 ) ;
#22954=CARTESIAN_POINT ( 'NONE',  ( -418.0000000000000568, 141.0000000000000000, 154.9999999999999716 ) ) ;
#22957=VECTOR ( 'NONE', #14699, 1000.000000000000000 ) ;
#22959=LINE ( 'NONE', #33808, #22829 ) ;
#22960=LINE ( 'NONE', #22781, #9942 ) ;
#22961=CARTESIAN_POINT ( 'NONE',  ( -12.00000000000001066, -64.99999999999997158, 154.9999999999999716 ) ) ;
#22965=ORIENTED_EDGE ( 'NONE', *, *, #26385, .T. ) ;
#22967=CIRCLE ( 'NONE', #7602, 7.999999999999979572 ) ;
#22970=FACE_OUTER_BOUND ( 'NONE', #16817, .T. ) ;
#22972=DIRECTION ( 'NONE',  ( 0.000000000000000000, -1.000000000000000000, -2.465190328815662439E-32 ) ) ;
#22974=LINE ( 'NONE', #25100, #32291 ) ;
#22975=VECTOR ( 'NONE', #22997, 1000.000000000000000 ) ;
#22976=ORIENTED_EDGE ( 'NONE', *, *, #9196, .T. ) ;
#22977=ORIENTED_EDGE ( 'NONE', *, *, #25463, .F. ) ;
#22978=AXIS2_PLACEMENT_3D ( 'NONE', #29520, #16358, #32704 ) ;
#22979=CARTESIAN_POINT ( 'NONE',  ( -499.9999999999999432, -137.0000000000000000, -162.9999999999999716 ) ) ;
#22983=CARTESIAN_POINT ( 'NONE',  ( -15.99999999999998579, 4.559999999999909015, 177.7400000000000091 ) ) ;
#22984=LINE ( 'NONE', #1783, #23926 ) ;
#22985=VERTEX_POINT ( 'NONE', #25434 ) ;
#22988=EDGE_LOOP ( 'NONE', ( #31788, #15504, #10625, #20575 ) ) ;
#22989=EDGE_CURVE ( 'NONE', #2726, #17921, #5199, .T. ) ;
#22990=DIRECTION ( 'NONE',  ( 1.000000000000000000, 3.469446951953834515E-18, 0.000000000000000000 ) ) ;
#22993=DIRECTION ( 'NONE',  ( 0.000000000000000000, 0.000000000000000000, -1.000000000000000000 ) ) ;
#22997=DIRECTION ( 'NONE',  ( 0.000000000000000000, 1.131431318426415506E-52, 1.000000000000000000 ) ) ;
#22998=CARTESIAN_POINT ( 'NONE',  ( 12.00000000000001066, -64.99999999999997158, -154.9999999999999716 ) ) ;
#23002=CIRCLE ( 'NONE', #20711, 3.999999999999982681 ) ;
#23003=EDGE_CURVE ( 'NONE', #1486, #34521, #1068, .T. ) ;
#23007=VERTEX_POINT ( 'NONE', #6567 ) ;
#23008=AXIS2_PLACEMENT_3D ( 'NONE', #26926, #32433, #27538 ) ;
#23014=EDGE_LOOP ( 'NONE', ( #19922, #27503, #23838, #2944 ) ) ;
#23019=VECTOR ( 'NONE', #10542, 1000.000000000000000 ) ;
#23021=CARTESIAN_POINT ( 'NONE',  ( -12.00000000000001066, 124.9999999999999716, 159.0000000000000000 ) ) ;
#23023=VERTEX_POINT ( 'NONE', #12109 ) ;
#23025=CARTESIAN_POINT ( 'NONE',  ( -19.99999999999998934, 75.55999999999990280, 172.9900000000000091 ) ) ;
#23027=AXIS2_PLACEMENT_3D ( 'NONE', #32503, #8125, #7951 ) ;
#23032=CARTESIAN_POINT ( 'NONE',  ( -12.00000000000003908, -145.0000000000000000, -154.9999999999999716 ) ) ;
#23033=CARTESIAN_POINT ( 'NONE',  ( 12.00000000000001066, -28.99999999999999645, -175.0000000000000000 ) ) ;
#23034=VECTOR ( 'NONE', #11974, 1000.000000000000000 ) ;
#23038=VERTEX_POINT ( 'NONE', #3195 ) ;
#23039=CIRCLE ( 'NONE', #20768, 2.000000000000001776 ) ;
#23040=CARTESIAN_POINT ( 'NONE',  ( -15.99999999999998579, -32.99999999999997158, -175.0000000000000000 ) ) ;
#23041=CARTESIAN_POINT ( 'NONE',  ( -19.99999999999998934, -137.0000000000000000, 162.9999999999999716 ) ) ;
#23044=DIRECTION ( 'NONE',  ( -0.000000000000000000, 1.000000000000000000, -0.000000000000000000 ) ) ;
#23046=EDGE_CURVE ( 'NONE', #21039, #26588, #10916, .T. ) ;
#23047=EDGE_CURVE ( 'NONE', #21471, #22985, #20631, .T. ) ;
#23049=ORIENTED_EDGE ( 'NONE', *, *, #14840, .F. ) ;
#23051=FACE_OUTER_BOUND ( 'NONE', #20622, .T. ) ;
#23053=VECTOR ( 'NONE', #2509, 1000.000000000000000 ) ;
#23054=ORIENTED_EDGE ( 'NONE', *, *, #18772, .T. ) ;
#23060=AXIS2_PLACEMENT_3D ( 'NONE', #19726, #16891, #6170 ) ;
#23064=VERTEX_POINT ( 'NONE', #20458 ) ;
#23067=VECTOR ( 'NONE', #21551, 1000.000000000000000 ) ;
#23070=EDGE_CURVE ( 'NONE', #22194, #31417, #1921, .T. ) ;
#23072=EDGE_CURVE ( 'NONE', #1486, #11417, #25784, .T. ) ;
#23073=DIRECTION ( 'NONE',  ( -1.000000000000000000, 0.000000000000000000, 0.000000000000000000 ) ) ;
#23078=LINE ( 'NONE', #28750, #7843 ) ;
#23081=DIRECTION ( 'NONE',  ( 0.000000000000000000, 0.000000000000000000, -1.000000000000000000 ) ) ;
#23084=CARTESIAN_POINT ( 'NONE',  ( -365.0000000000000000, 118.9999999999999858, 128.0000000000000000 ) ) ;
#23088=LINE ( 'NONE', #27879, #18322 ) ;
#23089=CARTESIAN_POINT ( 'NONE',  ( -442.0000000000000000, -105.0000000000000142, -174.9999999999999432 ) ) ;
#23091=ADVANCED_FACE ( 'NONE', ( #4061 ), #26134, .F. ) ;
#23093=PLANE ( 'NONE',  #13280 ) ;
#23095=CYLINDRICAL_SURFACE ( 'NONE', #20510, 4.000000000000003553 ) ;
#23098=AXIS2_PLACEMENT_3D ( 'NONE', #28227, #20399, #31242 ) ;
#23103=AXIS2_PLACEMENT_3D ( 'NONE', #2383, #29623, #34979 ) ;
#23108=FACE_OUTER_BOUND ( 'NONE', #15049, .T. ) ;
#23112=LINE ( 'NONE', #26115, #11069 ) ;
#23113=CARTESIAN_POINT ( 'NONE',  ( -442.0000000000000000, -105.0000000000000142, 194.9999999999999716 ) ) ;
#23115=EDGE_LOOP ( 'NONE', ( #8696, #10442, #2020, #15923, #2124, #34793, #10451, #5065, #5138, #31810 ) ) ;
#23117=ORIENTED_EDGE ( 'NONE', *, *, #31549, .T. ) ;
#23120=AXIS2_PLACEMENT_3D ( 'NONE', #28388, #3979, #3811 ) ;
#23123=CYLINDRICAL_SURFACE ( 'NONE', #28126, 7.999999999999979572 ) ;
#23125=CARTESIAN_POINT ( 'NONE',  ( -410.0000000000000568, 113.0000000000000000, -155.0000000000000000 ) ) ;
#23132=CIRCLE ( 'NONE', #24219, 2.000000000000001776 ) ;
#23133=CARTESIAN_POINT ( 'NONE',  ( 11.99999999999999645, 136.9999999999999716, -175.0000000000000284 ) ) ;
#23134=CARTESIAN_POINT ( 'NONE',  ( -414.0000000000000568, -125.0000000000000000, 187.0000000000000000 ) ) ;
#23137=DIRECTION ( 'NONE',  ( 0.000000000000000000, -3.374343856708137958E-53, 1.000000000000000000 ) ) ;
#23141=EDGE_CURVE ( 'NONE', #33356, #34959, #12975, .T. ) ;
#23142=CARTESIAN_POINT ( 'NONE',  ( 11.99999999999999645, 144.9999999999999716, 162.9999999999999716 ) ) ;
#23144=EDGE_LOOP ( 'NONE', ( #29606, #21698, #29089, #28064, #16199, #25127, #7020, #31409 ) ) ;
#23146=EDGE_LOOP ( 'NONE', ( #23462, #27353, #2940, #2916 ) ) ;
#23147=VECTOR ( 'NONE', #33617, 1000.000000000000000 ) ;
#23149=EDGE_CURVE ( 'NONE', #30081, #23628, #18841, .T. ) ;
#23150=CARTESIAN_POINT ( 'NONE',  ( -500.0000000000000000, -113.0000000000000000, 187.0000000000000000 ) ) ;
#23151=CIRCLE ( 'NONE', #18604, 7.999999999999952038 ) ;
#23158=CARTESIAN_POINT ( 'NONE',  ( -430.0000000000000000, -131.0000000000000000, 113.9999999999999858 ) ) ;
#23163=CARTESIAN_POINT ( 'NONE',  ( -365.0000000000000000, 130.9999999999999716, 113.9999999999999858 ) ) ;
#23166=DIRECTION ( 'NONE',  ( -1.300283923313630633E-47, 0.000000000000000000, -1.000000000000000000 ) ) ;
#23168=VERTEX_POINT ( 'NONE', #32516 ) ;
#23171=DIRECTION ( 'NONE',  ( -3.040835319149746528E-31, -1.000000000000000000, 0.000000000000000000 ) ) ;
#23175=CARTESIAN_POINT ( 'NONE',  ( -499.9999999999999432, -105.0000000000000142, -162.9999999999999716 ) ) ;
#23178=DIRECTION ( 'NONE',  ( 1.000000000000000000, 3.469446951953834515E-18, 0.000000000000000000 ) ) ;
#23182=ORIENTED_EDGE ( 'NONE', *, *, #2205, .F. ) ;
#23184=ADVANCED_FACE ( 'NONE', ( #2627 ), #13150, .T. ) ;
#23185=EDGE_CURVE ( 'NONE', #15934, #19179, #10475, .T. ) ;
#23191=EDGE_CURVE ( 'NONE', #30714, #27733, #27185, .T. ) ;
#23192=CARTESIAN_POINT ( 'NONE',  ( 12.00000000000001066, -134.9999999999999716, 194.9999999999999716 ) ) ;
#23196=CARTESIAN_POINT ( 'NONE',  ( -347.0000000000000000, -125.0000000000000284, 168.9999999999999716 ) ) ;
#23197=DIRECTION ( 'NONE',  ( -0.000000000000000000, -1.000000000000000000, -0.000000000000000000 ) ) ;
#23202=EDGE_CURVE ( 'NONE', #11184, #12833, #23982, .T. ) ;
#23206=EDGE_LOOP ( 'NONE', ( #23251, #8778, #2883, #33006 ) ) ;
#23209=LINE ( 'NONE', #12008, #33867 ) ;
#23210=DIRECTION ( 'NONE',  ( 0.000000000000000000, 1.000000000000000000, 0.000000000000000000 ) ) ;
#23214=CARTESIAN_POINT ( 'NONE',  ( -361.0000000000000000, 124.9999999999999432, 168.9999999999999716 ) ) ;
#23215=LINE ( 'NONE', #20715, #32564 ) ;
#23217=DIRECTION ( 'NONE',  ( 0.000000000000000000, 0.000000000000000000, 1.000000000000000000 ) ) ;
#23222=FACE_OUTER_BOUND ( 'NONE', #23014, .T. ) ;
#23223=PLANE ( 'NONE',  #27084 ) ;
#23224=AXIS2_PLACEMENT_3D ( 'NONE', #32499, #8121, #5447 ) ;
#23228=ORIENTED_EDGE ( 'NONE', *, *, #18618, .F. ) ;
#23229=ADVANCED_FACE ( 'NONE', ( #11357 ), #33231, .F. ) ;
#23233=ORIENTED_EDGE ( 'NONE', *, *, #23821, .F. ) ;
#23234=EDGE_LOOP ( 'NONE', ( #737, #11231, #26410, #3424 ) ) ;
#23237=EDGE_CURVE ( 'NONE', #21957, #12207, #17744, .T. ) ;
#23239=AXIS2_PLACEMENT_3D ( 'NONE', #19884, #5971, #2294 ) ;
#23242=ADVANCED_FACE ( 'NONE', ( #30572 ), #22203, .T. ) ;
#23247=PLANE ( 'NONE',  #28299 ) ;
#23250=DIRECTION ( 'NONE',  ( -1.000000000000000000, 0.000000000000000000, 0.000000000000000000 ) ) ;
#23251=ORIENTED_EDGE ( 'NONE', *, *, #14391, .F. ) ;
#23253=CYLINDRICAL_SURFACE ( 'NONE', #9957, 7.999999999999952038 ) ;
#23257=CARTESIAN_POINT ( 'NONE',  ( 0.000000000000000000, 144.9999999999999716, -154.9999999999999716 ) ) ;
#23260=FACE_OUTER_BOUND ( 'NONE', #13040, .T. ) ;
#23261=VERTEX_POINT ( 'NONE', #11532 ) ;
#23265=DIRECTION ( 'NONE',  ( 0.000000000000000000, 1.310824597558155437E-49, 1.000000000000000000 ) ) ;
#23269=ORIENTED_EDGE ( 'NONE', *, *, #29689, .F. ) ;
#23271=CARTESIAN_POINT ( 'NONE',  ( -499.9999999999999432, 136.9999999999999432, 155.0000000000000000 ) ) ;
#23273=VECTOR ( 'NONE', #3304, 1000.000000000000000 ) ;
#23278=ORIENTED_EDGE ( 'NONE', *, *, #20298, .F. ) ;
#23279=LINE ( 'NONE', #26111, #15609 ) ;
#23280=CARTESIAN_POINT ( 'NONE',  ( -500.0000000000000000, -115.0000000000000000, 155.0000000000000000 ) ) ;
#23283=EDGE_CURVE ( 'NONE', #11639, #11066, #22380, .T. ) ;
#23288=FACE_OUTER_BOUND ( 'NONE', #22439, .T. ) ;
#23290=LINE ( 'NONE', #23451, #17915 ) ;
#23296=CARTESIAN_POINT ( 'NONE',  ( -442.0000000000000000, 141.0000000000000000, 154.9999999999999716 ) ) ;
#23299=LINE ( 'NONE', #23134, #8102 ) ;
#23300=ORIENTED_EDGE ( 'NONE', *, *, #29206, .T. ) ;
#23303=PLANE ( 'NONE',  #15041 ) ;
#23305=EDGE_CURVE ( 'NONE', #28417, #15781, #14911, .T. ) ;
#23307=CARTESIAN_POINT ( 'NONE',  ( -442.0000000000000000, -125.0000000000000000, -101.9999999999999858 ) ) ;
#23308=CYLINDRICAL_SURFACE ( 'NONE', #2539, 7.999999999999979572 ) ;
#23309=ADVANCED_FACE ( 'NONE', ( #9723 ), #1545, .T. ) ;
#23315=DIRECTION ( 'NONE',  ( 1.000000000000000000, 0.000000000000000000, 0.000000000000000000 ) ) ;
#23316=EDGE_CURVE ( 'NONE', #30469, #4119, #30750, .T. ) ;
#23317=CARTESIAN_POINT ( 'NONE',  ( -442.0000000000000000, 113.0000000000000000, -175.0000000000000000 ) ) ;
#23318=VERTEX_POINT ( 'NONE', #22913 ) ;
#23319=DIRECTION ( 'NONE',  ( -1.232595164407830946E-32, -3.421138828918010427E-49, 1.000000000000000000 ) ) ;
#23324=ORIENTED_EDGE ( 'NONE', *, *, #25915, .F. ) ;
#23326=CARTESIAN_POINT ( 'NONE',  ( -410.0000000000000568, 105.0000000000000000, -77.99999999999997158 ) ) ;
#23331=EDGE_LOOP ( 'NONE', ( #4460, #22068, #33313, #8024 ) ) ;
#23336=PLANE ( 'NONE',  #6525 ) ;
#23340=DIRECTION ( 'NONE',  ( 0.000000000000000000, 1.000000000000000000, 0.000000000000000000 ) ) ;
#23342=AXIS2_PLACEMENT_3D ( 'NONE', #24846, #24481, #8481 ) ;
#23343=CIRCLE ( 'NONE', #6278, 3.999999999999976019 ) ;
#23347=CIRCLE ( 'NONE', #20506, 7.999999999999979572 ) ;
#23350=VECTOR ( 'NONE', #16311, 1000.000000000000000 ) ;
#23351=ORIENTED_EDGE ( 'NONE', *, *, #2723, .F. ) ;
#23353=LINE ( 'NONE', #1298, #8241 ) ;
#23355=ORIENTED_EDGE ( 'NONE', *, *, #3557, .F. ) ;
#23357=FACE_BOUND ( 'NONE', #29842, .T. ) ;
#23361=AXIS2_PLACEMENT_3D ( 'NONE', #12399, #28926, #15584 ) ;
#23364=DIRECTION ( 'NONE',  ( -0.000000000000000000, 1.000000000000000000, -0.000000000000000000 ) ) ;
#23365=DIRECTION ( 'NONE',  ( 1.000000000000000000, 0.000000000000000000, 0.000000000000000000 ) ) ;
#23367=AXIS2_PLACEMENT_3D ( 'NONE', #19303, #2902, #2380 ) ;
#23368=CARTESIAN_POINT ( 'NONE',  ( -500.0000000000000000, -145.0000000000000000, 162.9999999999999716 ) ) ;
#23369=CARTESIAN_POINT ( 'NONE',  ( -445.9999999999999432, -105.0000000000000142, 132.0000000000000000 ) ) ;
#23374=DIRECTION ( 'NONE',  ( 1.000000000000000000, 0.000000000000000000, 0.000000000000000000 ) ) ;
#23377=DIRECTION ( 'NONE',  ( 0.000000000000000000, -1.000000000000000000, 0.000000000000000000 ) ) ;
#23378=ADVANCED_FACE ( 'NONE', ( #23607 ), #7041, .F. ) ;
#23379=AXIS2_PLACEMENT_3D ( 'NONE', #17133, #30109, #27438 ) ;
#23380=AXIS2_PLACEMENT_3D ( 'NONE', #16578, #27410, #18721 ) ;
#23381=CARTESIAN_POINT ( 'NONE',  ( -20.00000000000007461, 140.9999999999999432, 187.0000000000000000 ) ) ;
#23385=MECHANICAL_DESIGN_GEOMETRIC_PRESENTATION_REPRESENTATION('',(#651),#29068);
#23386=CARTESIAN_POINT ( 'NONE',  ( -414.0000000000000568, 104.9999999999999858, -187.0000000000000000 ) ) ;
#23395=ORIENTED_EDGE ( 'NONE', *, *, #25479, .T. ) ;
#23396=CARTESIAN_POINT ( 'NONE',  ( -499.9999999999999432, -137.0000000000000000, -194.9999999999999716 ) ) ;
#23398=STYLED_ITEM('',(#35254),#34343);
#23399=CARTESIAN_POINT ( 'NONE',  ( -20.00000000000001776, -113.0000000000000000, 194.9999999999999716 ) ) ;
#23400=AXIS2_PLACEMENT_3D ( 'NONE', #8134, #16349, #16880 ) ;
#23403=ORIENTED_EDGE ( 'NONE', *, *, #12501, .F. ) ;
#23404=VERTEX_POINT ( 'NONE', #4535 ) ;
#23406=LINE ( 'NONE', #31419, #8833 ) ;
#23408=( GEOMETRIC_REPRESENTATION_CONTEXT ( 3 ) GLOBAL_UNCERTAINTY_ASSIGNED_CONTEXT ( ( #11808 ) ) GLOBAL_UNIT_ASSIGNED_CONTEXT ( ( #9432, #28113, #3371 ) ) REPRESENTATION_CONTEXT ( 'NONE', 'WORKASPACE' ) );
#23410=DIRECTION ( 'NONE',  ( 0.000000000000000000, -1.000000000000000000, -5.145227585319922065E-49 ) ) ;
#23414=CARTESIAN_POINT ( 'NONE',  ( -414.0000000000000568, -105.0000000000000142, 107.9999999999999858 ) ) ;
#23416=VERTEX_POINT ( 'NONE', #26266 ) ;
#23418=CARTESIAN_POINT ( 'NONE',  ( -499.9999999999999432, 136.9999999999999432, -194.9999999999999716 ) ) ;
#23420=AXIS2_PLACEMENT_3D ( 'NONE', #19352, #19529, #5790 ) ;
#23421=DIRECTION ( 'NONE',  ( -0.000000000000000000, 1.000000000000000000, -0.000000000000000000 ) ) ;
#23423=LINE ( 'NONE', #10073, #27491 ) ;
#23426=LINE ( 'NONE', #31264, #13704 ) ;
#23432=EDGE_CURVE ( 'NONE', #1235, #22809, #6698, .T. ) ;
#23433=LINE ( 'NONE', #4375, #5749 ) ;
#23440=ORIENTED_EDGE ( 'NONE', *, *, #31894, .F. ) ;
#23442=CARTESIAN_POINT ( 'NONE',  ( -19.99999999999998934, 75.55999999999990280, 172.9900000000000091 ) ) ;
#23443=CARTESIAN_POINT ( 'NONE',  ( 19.99999999999998934, -145.0000000000000000, -186.9999999999999716 ) ) ;
#23447=ORIENTED_EDGE ( 'NONE', *, *, #9673, .F. ) ;
#23451=CARTESIAN_POINT ( 'NONE',  ( 11.99999999999999645, -124.9999999999999432, -158.9999999999999716 ) ) ;
#23455=AXIS2_PLACEMENT_3D ( 'NONE', #22374, #8662, #21835 ) ;
#23456=DIRECTION ( 'NONE',  ( 0.000000000000000000, -1.000000000000000000, -2.465190328815662439E-32 ) ) ;
#23457=ORIENTED_EDGE ( 'NONE', *, *, #26797, .F. ) ;
#23462=ORIENTED_EDGE ( 'NONE', *, *, #34727, .F. ) ;
#23464=EDGE_CURVE ( 'NONE', #14949, #4850, #24457, .T. ) ;
#23465=FACE_OUTER_BOUND ( 'NONE', #24192, .T. ) ;
#23471=ORIENTED_EDGE ( 'NONE', *, *, #26865, .T. ) ;
#23474=VECTOR ( 'NONE', #19247, 1000.000000000000000 ) ;
#23479=CARTESIAN_POINT ( 'NONE',  ( 11.99999999999995559, -134.9999999999999716, -194.9999999999999432 ) ) ;
#23484=CARTESIAN_POINT ( 'NONE',  ( -430.0000000000000000, 114.9999999999999716, 126.0000000000000000 ) ) ;
#23485=ADVANCED_FACE ( 'NONE', ( #4896 ), #15789, .F. ) ;
#23487=CIRCLE ( 'NONE', #31996, 2.000000000000001776 ) ;
#23488=CARTESIAN_POINT ( 'NONE',  ( -441.9999999999999432, -141.0000000000000000, 154.9999999999999716 ) ) ;
#23491=VERTEX_POINT ( 'NONE', #10428 ) ;
#23492=CARTESIAN_POINT ( 'NONE',  ( 15.99999999999998579, 75.55999999999990280, -172.9900000000000091 ) ) ;
#23500=AXIS2_PLACEMENT_3D ( 'NONE', #19078, #8275, #30158 ) ;
#23501=CIRCLE ( 'NONE', #8153, 3.999999999999976019 ) ;
#23503=ORIENTED_EDGE ( 'NONE', *, *, #3948, .F. ) ;
#23505=DIRECTION ( 'NONE',  ( -1.232595164407830946E-32, -3.421138828918010427E-49, 1.000000000000000000 ) ) ;
#23509=EDGE_CURVE ( 'NONE', #20630, #22441, #32134, .T. ) ;
#23510=EDGE_CURVE ( 'NONE', #12627, #18640, #5424, .T. ) ;
#23516=MANIFOLD_SOLID_BREP ( 'Cut-Extrude1', #17395 ) ;
#23530=EDGE_CURVE ( 'NONE', #25265, #25155, #2756, .T. ) ;
#23533=CARTESIAN_POINT ( 'NONE',  ( 15.99999999999998579, -56.99999999999997868, -175.0000000000000000 ) ) ;
#23536=CARTESIAN_POINT ( 'NONE',  ( -414.0000000000000568, -105.0000000000000142, -101.9999999999999858 ) ) ;
#23541=ORIENTED_EDGE ( 'NONE', *, *, #20612, .T. ) ;
#23544=VECTOR ( 'NONE', #18992, 1000.000000000000000 ) ;
#23545=PLANE ( 'NONE',  #1673 ) ;
#23548=VECTOR ( 'NONE', #24924, 1000.000000000000000 ) ;
#23549=CARTESIAN_POINT ( 'NONE',  ( -12.00000000000001066, 134.9999999999999432, -186.9999999999999716 ) ) ;
#23552=LINE ( 'NONE', #12368, #21772 ) ;
#23555=AXIS2_PLACEMENT_3D ( 'NONE', #8936, #22119, #22292 ) ;
#23563=ORIENTED_EDGE ( 'NONE', *, *, #31868, .F. ) ;
#23566=ORIENTED_EDGE ( 'NONE', *, *, #1927, .T. ) ;
#23567=CIRCLE ( 'NONE', #29822, 7.999999999999979572 ) ;
#23568=ORIENTED_EDGE ( 'NONE', *, *, #21653, .F. ) ;
#23570=EDGE_LOOP ( 'NONE', ( #26955, #31863, #16027, #29474 ) ) ;
#23571=ORIENTED_EDGE ( 'NONE', *, *, #29136, .T. ) ;
#23573=AXIS2_PLACEMENT_3D ( 'NONE', #25238, #28094, #874 ) ;
#23580=DIRECTION ( 'NONE',  ( 0.000000000000000000, -3.374343856708137958E-53, 1.000000000000000000 ) ) ;
#23581=ORIENTED_EDGE ( 'NONE', *, *, #34960, .T. ) ;
#23583=CIRCLE ( 'NONE', #4813, 3.999999999999976019 ) ;
#23584=CARTESIAN_POINT ( 'NONE',  ( -363.0000000000000000, 134.9999999999999716, 126.0000000000000000 ) ) ;
#23586=DIRECTION ( 'NONE',  ( 0.000000000000000000, -1.000000000000000000, -0.000000000000000000 ) ) ;
#23589=FACE_OUTER_BOUND ( 'NONE', #1690, .T. ) ;
#23590=ORIENTED_EDGE ( 'NONE', *, *, #31366, .F. ) ;
#23596=CARTESIAN_POINT ( 'NONE',  ( -12.00000000000001066, -124.9999999999999432, -154.9999999999999716 ) ) ;
#23601=CIRCLE ( 'NONE', #3701, 3.999999999999976019 ) ;
#23602=DIRECTION ( 'NONE',  ( 0.000000000000000000, -1.000000000000000000, -5.145227585319922065E-49 ) ) ;
#23606=AXIS2_PLACEMENT_3D ( 'NONE', #31935, #34448, #13443 ) ;
#23607=FACE_OUTER_BOUND ( 'NONE', #19772, .T. ) ;
#23608=VERTEX_POINT ( 'NONE', #25309 ) ;
#23610=FACE_OUTER_BOUND ( 'NONE', #12088, .T. ) ;
#23613=CIRCLE ( 'NONE', #28716, 7.999999999999979572 ) ;
#23620=ORIENTED_EDGE ( 'NONE', *, *, #2668, .F. ) ;
#23623=DIRECTION ( 'NONE',  ( 1.000000000000000000, 0.000000000000000000, 0.000000000000000000 ) ) ;
#23624=VECTOR ( 'NONE', #25728, 1000.000000000000000 ) ;
#23627=FACE_OUTER_BOUND ( 'NONE', #26998, .T. ) ;
#23628=VERTEX_POINT ( 'NONE', #22998 ) ;
#23629=ORIENTED_EDGE ( 'NONE', *, *, #19818, .F. ) ;
#23632=PLANE ( 'NONE',  #2128 ) ;
#23634=DIRECTION ( 'NONE',  ( -1.000000000000000000, 0.000000000000000000, -0.000000000000000000 ) ) ;
#23636=FACE_BOUND ( 'NONE', #32709, .T. ) ;
#23642=CARTESIAN_POINT ( 'NONE',  ( 11.99999999999999645, 124.9999999999999716, 155.0000000000000000 ) ) ;
#23645=DIRECTION ( 'NONE',  ( 0.000000000000000000, 1.131431318426415506E-52, 1.000000000000000000 ) ) ;
#23648=DIRECTION ( 'NONE',  ( 1.000000000000000000, 0.000000000000000000, 0.000000000000000000 ) ) ;
#23649=VECTOR ( 'NONE', #8780, 1000.000000000000000 ) ;
#23650=LINE ( 'NONE', #31821, #34737 ) ;
#23651=CARTESIAN_POINT ( 'NONE',  ( -418.0000000000000000, 124.9999999999999432, -162.9999999999999716 ) ) ;
#23653=AXIS2_PLACEMENT_3D ( 'NONE', #15463, #33315, #14643 ) ;
#23663=ORIENTED_EDGE ( 'NONE', *, *, #27974, .T. ) ;
#23665=CARTESIAN_POINT ( 'NONE',  ( -349.0000000000000000, -125.0000000000000284, 164.9999999999999716 ) ) ;
#23666=EDGE_CURVE ( 'NONE', #23700, #17587, #9294, .T. ) ;
#23668=DIRECTION ( 'NONE',  ( 1.000000000000000000, 3.469446951953834515E-18, 0.000000000000000000 ) ) ;
#23678=CARTESIAN_POINT ( 'NONE',  ( -442.0000000000000000, -109.0000000000000142, 155.0000000000000000 ) ) ;
#23679=ORIENTED_EDGE ( 'NONE', *, *, #1394, .T. ) ;
#23680=DIRECTION ( 'NONE',  ( 1.000000000000000000, 0.000000000000000000, 0.000000000000000000 ) ) ;
#23682=VECTOR ( 'NONE', #22335, 1000.000000000000000 ) ;
#23683=DIRECTION ( 'NONE',  ( 0.000000000000000000, 0.000000000000000000, 1.000000000000000000 ) ) ;
#23688=DIRECTION ( 'NONE',  ( 0.000000000000000000, 1.000000000000000000, -3.374343856708137958E-53 ) ) ;
#23689=DIRECTION ( 'NONE',  ( 0.000000000000000000, 1.310824597558155437E-49, 1.000000000000000000 ) ) ;
#23690=CYLINDRICAL_SURFACE ( 'NONE', #27513, 7.999999999999979572 ) ;
#23693=FACE_OUTER_BOUND ( 'NONE', #32187, .T. ) ;
#23696=ADVANCED_FACE ( 'NONE', ( #18555 ), #4453, .F. ) ;
#23700=VERTEX_POINT ( 'NONE', #13197 ) ;
#23705=ORIENTED_EDGE ( 'NONE', *, *, #33723, .T. ) ;
#23706=LINE ( 'NONE', #21393, #24142 ) ;
#23709=CARTESIAN_POINT ( 'NONE',  ( -20.00000000000007461, 112.9999999999999574, 187.0000000000000000 ) ) ;
#23710=PLANE ( 'NONE',  #26230 ) ;
#23713=EDGE_CURVE ( 'NONE', #169, #27132, #34909, .T. ) ;
#23715=CARTESIAN_POINT ( 'NONE',  ( -12.00000000000001066, -32.99999999999997158, -175.0000000000000000 ) ) ;
#23720=LINE ( 'NONE', #5011, #6289 ) ;
#23724=AXIS2_PLACEMENT_3D ( 'NONE', #14196, #1142, #20193 ) ;
#23726=CARTESIAN_POINT ( 'NONE',  ( -365.0000000000000000, -131.0000000000000000, 109.9999999999999858 ) ) ;
#23730=DIRECTION ( 'NONE',  ( 0.000000000000000000, 0.000000000000000000, -1.000000000000000000 ) ) ;
#23733=CARTESIAN_POINT ( 'NONE',  ( -12.00000000000001066, -145.0000000000000000, -154.9999999999999716 ) ) ;
#23735=ORIENTED_EDGE ( 'NONE', *, *, #32382, .F. ) ;
#23736=LINE ( 'NONE', #1670, #22393 ) ;
#23737=PLANE ( 'NONE',  #2411 ) ;
#23738=LINE ( 'NONE', #17899, #9491 ) ;
#23739=EDGE_CURVE ( 'NONE', #22581, #14635, #24027, .T. ) ;
#23748=CIRCLE ( 'NONE', #24877, 7.999999999999979572 ) ;
#23749=EDGE_CURVE ( 'NONE', #24468, #14881, #10523, .T. ) ;
#23753=ORIENTED_EDGE ( 'NONE', *, *, #9771, .F. ) ;
#23754=ORIENTED_EDGE ( 'NONE', *, *, #19786, .F. ) ;
#23755=CARTESIAN_POINT ( 'NONE',  ( -449.9999999999999432, 104.9999999999999858, -175.0000000000000000 ) ) ;
#23757=DIRECTION ( 'NONE',  ( 1.000000000000000000, 0.000000000000000000, -0.000000000000000000 ) ) ;
#23758=CARTESIAN_POINT ( 'NONE',  ( -15.99999999999998579, 136.9999999999999716, 155.0000000000000000 ) ) ;
#23759=EDGE_LOOP ( 'NONE', ( #27690, #24267, #11087, #9025, #20849, #17728, #31594, #14474 ) ) ;
#23760=EDGE_LOOP ( 'NONE', ( #16735, #31472, #15326, #14344 ) ) ;
#23762=DIRECTION ( 'NONE',  ( 0.000000000000000000, -1.000000000000000000, 6.123233995736766036E-17 ) ) ;
#23764=DIRECTION ( 'NONE',  ( -1.000000000000000000, 0.000000000000000000, 0.000000000000000000 ) ) ;
#23766=LINE ( 'NONE', #28930, #871 ) ;
#23767=VECTOR ( 'NONE', #20864, 1000.000000000000000 ) ;
#23768=FACE_OUTER_BOUND ( 'NONE', #8640, .T. ) ;
#23773=ORIENTED_EDGE ( 'NONE', *, *, #20430, .T. ) ;
#23778=VECTOR ( 'NONE', #347, 1000.000000000000000 ) ;
#23782=DIRECTION ( 'NONE',  ( 0.000000000000000000, -1.000000000000000000, 6.842277657836020854E-49 ) ) ;
#23785=EDGE_CURVE ( 'NONE', #11116, #15497, #26706, .T. ) ;
#23786=VERTEX_POINT ( 'NONE', #28852 ) ;
#23787=LINE ( 'NONE', #1717, #26244 ) ;
#23789=ORIENTED_EDGE ( 'NONE', *, *, #23823, .T. ) ;
#23790=CIRCLE ( 'NONE', #7277, 7.999999999999979572 ) ;
#23792=ORIENTED_EDGE ( 'NONE', *, *, #31143, .T. ) ;
#23796=DIRECTION ( 'NONE',  ( 1.000000000000000000, 0.000000000000000000, 0.000000000000000000 ) ) ;
#23797=( GEOMETRIC_REPRESENTATION_CONTEXT ( 3 ) GLOBAL_UNCERTAINTY_ASSIGNED_CONTEXT ( ( #15585 ) ) GLOBAL_UNIT_ASSIGNED_CONTEXT ( ( #5257, #24133, #29318 ) ) REPRESENTATION_CONTEXT ( 'NONE', 'WORKASPACE' ) );
#23798=CARTESIAN_POINT ( 'NONE',  ( 11.99999999999999645, 134.9999999999998863, 155.0000000000000000 ) ) ;
#23801=ORIENTED_EDGE ( 'NONE', *, *, #15351, .F. ) ;
#23802=EDGE_LOOP ( 'NONE', ( #24659, #27806 ) ) ;
#23809=DIRECTION ( 'NONE',  ( 1.000000000000000000, -0.000000000000000000, -0.000000000000000000 ) ) ;
#23810=DIRECTION ( 'NONE',  ( 0.000000000000000000, -6.123233995736766036E-17, -1.000000000000000000 ) ) ;
#23815=DIRECTION ( 'NONE',  ( -1.000000000000000000, -3.469446951953834515E-18, 2.736911063134582149E-48 ) ) ;
#23819=ORIENTED_EDGE ( 'NONE', *, *, #23739, .F. ) ;
#23821=EDGE_CURVE ( 'NONE', #24518, #14045, #19245, .T. ) ;
#23823=EDGE_CURVE ( 'NONE', #27322, #33889, #29915, .T. ) ;
#23824=VERTEX_POINT ( 'NONE', #13373 ) ;
#23826=DIRECTION ( 'NONE',  ( 0.000000000000000000, 0.000000000000000000, -1.000000000000000000 ) ) ;
#23829=VERTEX_POINT ( 'NONE', #370 ) ;
#23833=DIRECTION ( 'NONE',  ( 0.000000000000000000, 0.000000000000000000, -1.000000000000000000 ) ) ;
#23835=AXIS2_PLACEMENT_3D ( 'NONE', #7685, #2178, #20702 ) ;
#23836=CARTESIAN_POINT ( 'NONE',  ( -365.0000000000000000, -131.0000000000000000, 113.9999999999999858 ) ) ;
#23838=ORIENTED_EDGE ( 'NONE', *, *, #18335, .T. ) ;
#23839=PLANE ( 'NONE',  #8499 ) ;
#23840=FACE_OUTER_BOUND ( 'NONE', #30839, .T. ) ;
#23845=ORIENTED_EDGE ( 'NONE', *, *, #29744, .T. ) ;
#23846=FACE_OUTER_BOUND ( 'NONE', #4631, .T. ) ;
#23848=ORIENTED_EDGE ( 'NONE', *, *, #17732, .T. ) ;
#23851=ORIENTED_EDGE ( 'NONE', *, *, #24709, .F. ) ;
#23854=CARTESIAN_POINT ( 'NONE',  ( -12.00000000000001066, -24.99999999999999289, 154.9999999999999716 ) ) ;
#23856=DIRECTION ( 'NONE',  ( 1.000000000000000000, 0.000000000000000000, -0.000000000000000000 ) ) ;
#23866=ORIENTED_EDGE ( 'NONE', *, *, #15312, .F. ) ;
#23867=ORIENTED_EDGE ( 'NONE', *, *, #11459, .F. ) ;
#23869=DIRECTION ( 'NONE',  ( 0.000000000000000000, -0.000000000000000000, -1.000000000000000000 ) ) ;
#23872=ORIENTED_EDGE ( 'NONE', *, *, #2644, .F. ) ;
#23877=VERTEX_POINT ( 'NONE', #3198 ) ;
#23885=DIRECTION ( 'NONE',  ( -0.000000000000000000, -1.000000000000000000, -0.000000000000000000 ) ) ;
#23887=DIRECTION ( 'NONE',  ( 1.000000000000000000, 0.000000000000000000, -1.232595164407831220E-32 ) ) ;
#23888=DIRECTION ( 'NONE',  ( 1.000000000000000000, 0.000000000000000000, 0.000000000000000000 ) ) ;
#23895=DIRECTION ( 'NONE',  ( 0.000000000000000000, -1.000000000000000000, -2.465190328815662439E-32 ) ) ;
#23897=CARTESIAN_POINT ( 'NONE',  ( -365.0000000000000000, 132.9999999999999716, 113.9999999999999858 ) ) ;
#23903=ORIENTED_EDGE ( 'NONE', *, *, #6002, .T. ) ;
#23904=ORIENTED_EDGE ( 'NONE', *, *, #28841, .F. ) ;
#23909=LINE ( 'NONE', #23755, #20177 ) ;
#23910=EDGE_CURVE ( 'NONE', #26015, #22194, #12594, .T. ) ;
#23911=AXIS2_PLACEMENT_3D ( 'NONE', #27474, #10399, #21258 ) ;
#23913=CYLINDRICAL_SURFACE ( 'NONE', #25621, 3.999999999999976019 ) ;
#23915=EDGE_LOOP ( 'NONE', ( #7228, #9818, #6482, #8118 ) ) ;
#23917=DIRECTION ( 'NONE',  ( 0.000000000000000000, 1.000000000000000000, -6.123233995736766036E-17 ) ) ;
#23919=EDGE_CURVE ( 'NONE', #2852, #34959, #10705, .T. ) ;
#23926=VECTOR ( 'NONE', #28838, 1000.000000000000000 ) ;
#23932=PLANE ( 'NONE',  #26240 ) ;
#23933=CARTESIAN_POINT ( 'NONE',  ( -410.0000000000000568, 124.9999999999999574, -187.0000000000000000 ) ) ;
#23937=CARTESIAN_POINT ( 'NONE',  ( -499.9999999999999432, -105.0000000000000142, -162.9999999999999716 ) ) ;
#23941=DIRECTION ( 'NONE',  ( 1.000000000000000000, 0.000000000000000000, 0.000000000000000000 ) ) ;
#23942=VECTOR ( 'NONE', #11914, 1000.000000000000000 ) ;
#23943=ORIENTED_EDGE ( 'NONE', *, *, #32382, .T. ) ;
#23944=ADVANCED_FACE ( 'NONE', ( #8895 ), #30616, .T. ) ;
#23946=LINE ( 'NONE', #34827, #22268 ) ;
#23955=DIRECTION ( 'NONE',  ( 1.000000000000000000, 3.469446951954617213E-18, -2.891205793294674875E-16 ) ) ;
#23966=EDGE_CURVE ( 'NONE', #16444, #11612, #14785, .T. ) ;
#23967=EDGE_CURVE ( 'NONE', #29489, #34521, #22959, .T. ) ;
#23980=ORIENTED_EDGE ( 'NONE', *, *, #28029, .T. ) ;
#23982=LINE ( 'NONE', #7785, #5780 ) ;
#23983=CARTESIAN_POINT ( 'NONE',  ( -499.9999999999999432, -137.0000000000000000, -162.9999999999999716 ) ) ;
#23984=ORIENTED_EDGE ( 'NONE', *, *, #4155, .T. ) ;
#23987=DIRECTION ( 'NONE',  ( 0.000000000000000000, -1.000000000000000000, -2.465190328815662439E-32 ) ) ;
#23991=EDGE_CURVE ( 'NONE', #21689, #995, #30440, .T. ) ;
#23993=CARTESIAN_POINT ( 'NONE',  ( -499.9999999999999432, 112.9999999999999574, -187.0000000000000000 ) ) ;
#24000=VECTOR ( 'NONE', #28421, 1000.000000000000000 ) ;
#24002=DIRECTION ( 'NONE',  ( 0.000000000000000000, 0.000000000000000000, 1.000000000000000000 ) ) ;
#24003=ADVANCED_FACE ( 'NONE', ( #6209 ), #3546, .F. ) ;
#24009=ORIENTED_EDGE ( 'NONE', *, *, #1952, .T. ) ;
#24011=ORIENTED_EDGE ( 'NONE', *, *, #2197, .F. ) ;
#24013=CARTESIAN_POINT ( 'NONE',  ( -365.0000000000000000, -114.9999999999999858, 126.0000000000000000 ) ) ;
#24014=ORIENTED_EDGE ( 'NONE', *, *, #13712, .T. ) ;
#24018=LINE ( 'NONE', #15695, #21491 ) ;
#24022=CYLINDRICAL_SURFACE ( 'NONE', #15088, 3.999999999999976019 ) ;
#24027=LINE ( 'NONE', #7474, #6318 ) ;
#24035=AXIS2_PLACEMENT_3D ( 'NONE', #34413, #20881, #31893 ) ;
#24040=CARTESIAN_POINT ( 'NONE',  ( -445.9999999999999432, -105.0000000000000142, -101.9999999999999858 ) ) ;
#24046=ORIENTED_EDGE ( 'NONE', *, *, #12425, .F. ) ;
#24047=ORIENTED_EDGE ( 'NONE', *, *, #19077, .T. ) ;
#24048=CIRCLE ( 'NONE', #8718, 7.999999999999979572 ) ;
#24049=DIRECTION ( 'NONE',  ( -0.000000000000000000, -0.000000000000000000, 1.000000000000000000 ) ) ;
#24053=LINE ( 'NONE', #34577, #17125 ) ;
#24054=CARTESIAN_POINT ( 'NONE',  ( -430.0000000000000000, 118.9999999999999716, 126.0000000000000000 ) ) ;
#24056=DIRECTION ( 'NONE',  ( 1.000000000000000000, 3.040835319149746090E-31, 1.232595164407830946E-32 ) ) ;
#24057=DIRECTION ( 'NONE',  ( 0.000000000000000000, 2.309213040847544338E-50, 1.000000000000000000 ) ) ;
#24058=CARTESIAN_POINT ( 'NONE',  ( -19.99999999999998934, -105.0000000000000142, 187.0000000000000000 ) ) ;
#24059=ADVANCED_FACE ( 'NONE', ( #26137 ), #10122, .F. ) ;
#24061=DIRECTION ( 'NONE',  ( 0.000000000000000000, 0.000000000000000000, -1.000000000000000000 ) ) ;
#24062=EDGE_CURVE ( 'NONE', #6872, #13784, #16569, .T. ) ;
#24066=DIRECTION ( 'NONE',  ( -3.040835319149746528E-31, -1.000000000000000000, 0.000000000000000000 ) ) ;
#24068=CARTESIAN_POINT ( 'NONE',  ( -12.00000000000001066, -124.9999999999999432, -154.9999999999999716 ) ) ;
#24069=ORIENTED_EDGE ( 'NONE', *, *, #32190, .T. ) ;
#24070=CYLINDRICAL_SURFACE ( 'NONE', #33184, 2.000000000000001776 ) ;
#24071=DIRECTION ( 'NONE',  ( 0.000000000000000000, 1.000000000000000000, 2.309213040847544338E-50 ) ) ;
#24075=VERTEX_POINT ( 'NONE', #4943 ) ;
#24077=FACE_OUTER_BOUND ( 'NONE', #24633, .T. ) ;
#24079=ORIENTED_EDGE ( 'NONE', *, *, #17597, .F. ) ;
#24082=ORIENTED_EDGE ( 'NONE', *, *, #5677, .T. ) ;
#24084=FACE_OUTER_BOUND ( 'NONE', #4868, .T. ) ;
#24085=AXIS2_PLACEMENT_3D ( 'NONE', #3821, #9869, #4340 ) ;
#24087=CARTESIAN_POINT ( 'NONE',  ( -418.0000000000000000, -124.9999999999999716, 132.0000000000000000 ) ) ;
#24095=VERTEX_POINT ( 'NONE', #20982 ) ;
#24109=DIRECTION ( 'NONE',  ( 1.000000000000000000, -0.000000000000000000, 0.000000000000000000 ) ) ;
#24119=FACE_OUTER_BOUND ( 'NONE', #22466, .T. ) ;
#24120=VECTOR ( 'NONE', #33259, 1000.000000000000000 ) ;
#24121=EDGE_CURVE ( 'NONE', #24780, #33691, #23650, .T. ) ;
#24122=ORIENTED_EDGE ( 'NONE', *, *, #29744, .F. ) ;
#24123=DIRECTION ( 'NONE',  ( 0.000000000000000000, 1.000000000000000000, 5.053935297177146739E-49 ) ) ;
#24133=( NAMED_UNIT ( * ) PLANE_ANGLE_UNIT ( ) SI_UNIT ( $, .RADIAN. ) );
#24135=FACE_OUTER_BOUND ( 'NONE', #2165, .T. ) ;
#24136=ORIENTED_EDGE ( 'NONE', *, *, #12983, .T. ) ;
#24138=ORIENTED_EDGE ( 'NONE', *, *, #23003, .F. ) ;
#24142=VECTOR ( 'NONE', #15898, 1000.000000000000000 ) ;
#24144=FACE_OUTER_BOUND ( 'NONE', #22832, .T. ) ;
#24145=EDGE_CURVE ( 'NONE', #980, #707, #35045, .T. ) ;
#24147=DIRECTION ( 'NONE',  ( -0.000000000000000000, -2.465190328815661892E-32, -1.000000000000000000 ) ) ;
#24148=CARTESIAN_POINT ( 'NONE',  ( -430.0000000000000000, -119.0000000000000000, 126.0000000000000000 ) ) ;
#24162=DIRECTION ( 'NONE',  ( -0.000000000000000000, 0.000000000000000000, 1.000000000000000000 ) ) ;
#24165=DIRECTION ( 'NONE',  ( 0.000000000000000000, 1.000000000000000000, -3.374343856708137958E-53 ) ) ;
#24169=EDGE_CURVE ( 'NONE', #19146, #34985, #21850, .T. ) ;
#24175=EDGE_LOOP ( 'NONE', ( #30351, #5621, #6789, #21712 ) ) ;
#24178=EDGE_CURVE ( 'NONE', #6460, #24468, #17184, .T. ) ;
#24184=ORIENTED_EDGE ( 'NONE', *, *, #24443, .F. ) ;
#24186=DIRECTION ( 'NONE',  ( 0.000000000000000000, 0.000000000000000000, -1.000000000000000000 ) ) ;
#24188=CARTESIAN_POINT ( 'NONE',  ( -442.0000000000000000, -125.0000000000000000, -105.9999999999999574 ) ) ;
#24189=VERTEX_POINT ( 'NONE', #8145 ) ;
#24192=EDGE_LOOP ( 'NONE', ( #25898, #28620, #6679, #31939 ) ) ;
#24198=FACE_OUTER_BOUND ( 'NONE', #29980, .T. ) ;
#24200=ADVANCED_FACE ( 'NONE', ( #2977 ), #13500, .T. ) ;
#24202=DIRECTION ( 'NONE',  ( 0.000000000000000000, -1.000000000000000000, 6.123233995736766036E-17 ) ) ;
#24210=EDGE_CURVE ( 'NONE', #9452, #6968, #33049, .T. ) ;
#24211=EDGE_CURVE ( 'NONE', #15708, #23824, #21674, .T. ) ;
#24212=ADVANCED_FACE ( 'NONE', ( #27192 ), #19203, .F. ) ;
#24217=ORIENTED_EDGE ( 'NONE', *, *, #30594, .T. ) ;
#24219=AXIS2_PLACEMENT_3D ( 'NONE', #22103, #5882, #27608 ) ;
#24224=VECTOR ( 'NONE', #32508, 1000.000000000000000 ) ;
#24225=DIRECTION ( 'NONE',  ( 1.000000000000000000, 0.000000000000000000, -0.000000000000000000 ) ) ;
#24232=AXIS2_PLACEMENT_3D ( 'NONE', #24421, #52, #10747 ) ;
#24234=DIRECTION ( 'NONE',  ( 0.000000000000000000, 0.000000000000000000, 1.000000000000000000 ) ) ;
#24235=DIRECTION ( 'NONE',  ( 1.000000000000000000, 0.000000000000000000, 1.300283923313630633E-47 ) ) ;
#24237=DIRECTION ( 'NONE',  ( 0.000000000000000000, 0.000000000000000000, -1.000000000000000000 ) ) ;
#24238=DIRECTION ( 'NONE',  ( -1.848892746611746419E-32, -6.842277657836020854E-49, 1.000000000000000000 ) ) ;
#24239=DIRECTION ( 'NONE',  ( 1.000000000000000000, 0.000000000000000000, 0.000000000000000000 ) ) ;
#24240=DIRECTION ( 'NONE',  ( 0.000000000000000000, 0.000000000000000000, -1.000000000000000000 ) ) ;
#24241=AXIS2_PLACEMENT_3D ( 'NONE', #25996, #7117, #28840 ) ;
#24242=DIRECTION ( 'NONE',  ( -3.469446951953832974E-18, -1.000000000000000000, 7.888609052210118054E-31 ) ) ;
#24243=DIRECTION ( 'NONE',  ( 0.000000000000000000, 0.000000000000000000, -1.000000000000000000 ) ) ;
#24246=AXIS2_PLACEMENT_3D ( 'NONE', #6727, #25595, #22765 ) ;
#24248=VERTEX_POINT ( 'NONE', #22034 ) ;
#24249=LINE ( 'NONE', #5721, #32082 ) ;
#24250=DIRECTION ( 'NONE',  ( 0.000000000000000000, 3.374343856708137958E-53, -1.000000000000000000 ) ) ;
#24251=EDGE_CURVE ( 'NONE', #25357, #28489, #3504, .T. ) ;
#24255=EDGE_CURVE ( 'NONE', #1478, #29515, #27363, .T. ) ;
#24256=VERTEX_POINT ( 'NONE', #30210 ) ;
#24259=ORIENTED_EDGE ( 'NONE', *, *, #21653, .T. ) ;
#24261=LINE ( 'NONE', #29790, #27533 ) ;
#24263=VECTOR ( 'NONE', #23810, 1000.000000000000000 ) ;
#24267=ORIENTED_EDGE ( 'NONE', *, *, #22391, .T. ) ;
#24272=DIRECTION ( 'NONE',  ( 0.000000000000000000, 1.000000000000000000, 5.145227585319922065E-49 ) ) ;
#24273=ORIENTED_EDGE ( 'NONE', *, *, #32454, .T. ) ;
#24274=VECTOR ( 'NONE', #6503, 1000.000000000000000 ) ;
#24279=FACE_OUTER_BOUND ( 'NONE', #16153, .T. ) ;
#24280=FACE_OUTER_BOUND ( 'NONE', #12134, .T. ) ;
#24284=ORIENTED_EDGE ( 'NONE', *, *, #31300, .F. ) ;
#24285=DIRECTION ( 'NONE',  ( 1.000000000000000000, 0.000000000000000000, -1.232595164407831220E-32 ) ) ;
#24287=DIRECTION ( 'NONE',  ( 0.000000000000000000, 0.000000000000000000, 1.000000000000000000 ) ) ;
#24288=EDGE_CURVE ( 'NONE', #26055, #15405, #16004, .T. ) ;
#24289=CIRCLE ( 'NONE', #3842, 4.750000000000004441 ) ;
#24292=ADVANCED_FACE ( 'NONE', ( #851 ), #6528, .F. ) ;
#24293=EDGE_CURVE ( 'NONE', #22621, #9284, #22383, .T. ) ;
#24294=ORIENTED_EDGE ( 'NONE', *, *, #19572, .T. ) ;
#24297=ADVANCED_FACE ( 'NONE', ( #11359 ), #6169, .T. ) ;
#24298=ORIENTED_EDGE ( 'NONE', *, *, #21552, .T. ) ;
#24301=ORIENTED_EDGE ( 'NONE', *, *, #11401, .F. ) ;
#24303=CARTESIAN_POINT ( 'NONE',  ( -365.0000000000000000, 130.9999999999999716, 113.9999999999999858 ) ) ;
#24305=CARTESIAN_POINT ( 'NONE',  ( -361.0000000000000000, -125.0000000000000284, 128.0000000000000000 ) ) ;
#24306=AXIS2_PLACEMENT_3D ( 'NONE', #23709, #4471, #26551 ) ;
#24312=DIRECTION ( 'NONE',  ( 0.000000000000000000, 0.000000000000000000, 1.000000000000000000 ) ) ;
#24316=VECTOR ( 'NONE', #18710, 1000.000000000000000 ) ;
#24318=DIRECTION ( 'NONE',  ( 0.000000000000000000, 0.000000000000000000, 1.000000000000000000 ) ) ;
#24320=DIRECTION ( 'NONE',  ( -1.000000000000000000, 0.000000000000000000, 0.000000000000000000 ) ) ;
#24322=ORIENTED_EDGE ( 'NONE', *, *, #13965, .F. ) ;
#24323=CARTESIAN_POINT ( 'NONE',  ( -20.00000000000004619, -124.9999999999999432, -162.9999999999999432 ) ) ;
#24325=VECTOR ( 'NONE', #1820, 1000.000000000000000 ) ;
#24326=DIRECTION ( 'NONE',  ( -1.000000000000000000, 0.000000000000000000, -1.292961597001347186E-16 ) ) ;
#24327=EDGE_LOOP ( 'NONE', ( #16807, #28955, #3132, #7960 ) ) ;
#24328=DIRECTION ( 'NONE',  ( 0.000000000000000000, 1.000000000000000000, 0.000000000000000000 ) ) ;
#24330=CARTESIAN_POINT ( 'NONE',  ( -499.9999999999999432, 136.9999999999999432, -187.0000000000000000 ) ) ;
#24331=AXIS2_PLACEMENT_3D ( 'NONE', #23163, #15329, #26159 ) ;
#24335=CARTESIAN_POINT ( 'NONE',  ( -12.00000000000001066, 144.9999999999999716, -162.9999999999999432 ) ) ;
#24338=ORIENTED_EDGE ( 'NONE', *, *, #21052, .F. ) ;
#24339=VECTOR ( 'NONE', #11368, 1000.000000000000000 ) ;
#24348=CIRCLE ( 'NONE', #18144, 4.000000000000003553 ) ;
#24349=DIRECTION ( 'NONE',  ( -0.000000000000000000, 1.000000000000000000, -0.000000000000000000 ) ) ;
#24350=DIRECTION ( 'NONE',  ( -1.000000000000000000, 0.000000000000000000, 0.000000000000000000 ) ) ;
#24354=ORIENTED_EDGE ( 'NONE', *, *, #5961, .T. ) ;
#24359=VECTOR ( 'NONE', #26080, 1000.000000000000000 ) ;
#24360=ORIENTED_EDGE ( 'NONE', *, *, #26865, .F. ) ;
#24363=ORIENTED_EDGE ( 'NONE', *, *, #9583, .F. ) ;
#24366=CARTESIAN_POINT ( 'NONE',  ( -445.9999999999999432, 105.0000000000000142, -101.9999999999999858 ) ) ;
#24368=EDGE_CURVE ( 'NONE', #20834, #14594, #34769, .T. ) ;
#24372=DIRECTION ( 'NONE',  ( 1.000000000000000000, 0.000000000000000000, 0.000000000000000000 ) ) ;
#24374=DIRECTION ( 'NONE',  ( 0.000000000000000000, 0.000000000000000000, -1.000000000000000000 ) ) ;
#24375=ORIENTED_EDGE ( 'NONE', *, *, #34154, .T. ) ;
#24379=CARTESIAN_POINT ( 'NONE',  ( 15.99999999999998579, -145.0000000000000000, 187.0000000000000000 ) ) ;
#24386=ORIENTED_EDGE ( 'NONE', *, *, #15048, .T. ) ;
#24387=CARTESIAN_POINT ( 'NONE',  ( -418.0000000000000000, -104.9999999999999858, -155.0000000000000000 ) ) ;
#24390=VERTEX_POINT ( 'NONE', #24866 ) ;
#24391=VECTOR ( 'NONE', #19520, 1000.000000000000000 ) ;
#24394=EDGE_LOOP ( 'NONE', ( #4537, #20552, #19833, #2338 ) ) ;
#24397=VECTOR ( 'NONE', #16897, 1000.000000000000000 ) ;
#24408=DIRECTION ( 'NONE',  ( 0.000000000000000000, -1.000000000000000000, -2.465190328815662439E-32 ) ) ;
#24409=CARTESIAN_POINT ( 'NONE',  ( -499.9999999999999432, 136.9999999999999432, 194.9999999999999716 ) ) ;
#24410=ADVANCED_FACE ( 'NONE', ( #30574 ), #17245, .F. ) ;
#24412=CIRCLE ( 'NONE', #2740, 2.000000000000001776 ) ;
#24413=CARTESIAN_POINT ( 'NONE',  ( -410.0000000000000568, -112.9999999999999858, -155.0000000000000000 ) ) ;
#24417=CARTESIAN_POINT ( 'NONE',  ( -15.99999999999998579, -145.0000000000000000, 162.9999999999999716 ) ) ;
#24419=CARTESIAN_POINT ( 'NONE',  ( -499.9999999999999432, 136.9999999999999432, 159.0000000000000000 ) ) ;
#24420=CARTESIAN_POINT ( 'NONE',  ( -499.9999999999999432, -113.0000000000000000, -162.9999999999999716 ) ) ;
#24421=CARTESIAN_POINT ( 'NONE',  ( -499.9999999999999432, 136.9999999999999432, -162.9999999999999716 ) ) ;
#24424=ORIENTED_EDGE ( 'NONE', *, *, #13519, .T. ) ;
#24429=VERTEX_POINT ( 'NONE', #22741 ) ;
#24430=CARTESIAN_POINT ( 'NONE',  ( -499.9999999999999432, 136.9999999999999432, 194.9999999999999716 ) ) ;
#24432=PLANE ( 'NONE',  #28477 ) ;
#24433=ORIENTED_EDGE ( 'NONE', *, *, #971, .F. ) ;
#24437=EDGE_CURVE ( 'NONE', #10330, #12319, #20424, .T. ) ;
#24443=EDGE_CURVE ( 'NONE', #19066, #4867, #34645, .T. ) ;
#24444=DIRECTION ( 'NONE',  ( 0.000000000000000000, 1.000000000000000000, -2.309213040847544338E-50 ) ) ;
#24445=ORIENTED_EDGE ( 'NONE', *, *, #23919, .T. ) ;
#24448=LINE ( 'NONE', #32989, #20592 ) ;
#24449=DIRECTION ( 'NONE',  ( 0.000000000000000000, 0.000000000000000000, -1.000000000000000000 ) ) ;
#24450=CARTESIAN_POINT ( 'NONE',  ( -20.00000000000007461, 104.9999999999999858, 162.9999999999999716 ) ) ;
#24451=ORIENTED_EDGE ( 'NONE', *, *, #23191, .T. ) ;
#24455=ORIENTED_EDGE ( 'NONE', *, *, #2391, .F. ) ;
#24457=LINE ( 'NONE', #18978, #2304 ) ;
#24462=ORIENTED_EDGE ( 'NONE', *, *, #367, .T. ) ;
#24463=VECTOR ( 'NONE', #6715, 1000.000000000000000 ) ;
#24465=LINE ( 'NONE', #106, #4971 ) ;
#24468=VERTEX_POINT ( 'NONE', #9729 ) ;
#24470=LINE ( 'NONE', #32152, #30664 ) ;
#24475=VERTEX_POINT ( 'NONE', #20941 ) ;
#24476=CARTESIAN_POINT ( 'NONE',  ( -19.99999999999998934, 134.9999999999998863, 187.0000000000000000 ) ) ;
#24477=DIRECTION ( 'NONE',  ( 0.000000000000000000, 0.000000000000000000, 1.000000000000000000 ) ) ;
#24480=ADVANCED_FACE ( 'NONE', ( #25933 ), #1550, .F. ) ;
#24481=DIRECTION ( 'NONE',  ( 0.000000000000000000, 2.309213040847544338E-50, 1.000000000000000000 ) ) ;
#24483=DIRECTION ( 'NONE',  ( 0.000000000000000000, 1.000000000000000000, 1.224646799147353207E-16 ) ) ;
#24487=ADVANCED_FACE ( 'NONE', ( #23610 ), #17763, .T. ) ;
#24490=AXIS2_PLACEMENT_3D ( 'NONE', #6497, #9178, #23073 ) ;
#24492=ORIENTED_EDGE ( 'NONE', *, *, #31257, .F. ) ;
#24497=EDGE_CURVE ( 'NONE', #33261, #8977, #23787, .T. ) ;
#24502=VECTOR ( 'NONE', #7967, 1000.000000000000000 ) ;
#24504=VECTOR ( 'NONE', #17382, 1000.000000000000000 ) ;
#24507=ORIENTED_EDGE ( 'NONE', *, *, #23316, .T. ) ;
#24513=DIRECTION ( 'NONE',  ( 1.000000000000000000, 0.000000000000000000, 5.546364386991661285E-52 ) ) ;
#24518=VERTEX_POINT ( 'NONE', #10083 ) ;
#24521=DIRECTION ( 'NONE',  ( -1.000000000000000000, 0.000000000000000000, -5.546364386991661285E-52 ) ) ;
#24525=VERTEX_POINT ( 'NONE', #31785 ) ;
#24531=VECTOR ( 'NONE', #28633, 1000.000000000000000 ) ;
#24534=CARTESIAN_POINT ( 'NONE',  ( -361.0000000000000000, 134.9999999999999716, 110.0000000000000000 ) ) ;
#24538=EDGE_CURVE ( 'NONE', #25895, #7844, #23433, .T. ) ;
#24539=ADVANCED_FACE ( 'NONE', ( #20766 ), #21110, .T. ) ;
#24540=DIRECTION ( 'NONE',  ( 0.000000000000000000, 1.000000000000000000, 5.053935297177146739E-49 ) ) ;
#24541=ORIENTED_EDGE ( 'NONE', *, *, #21204, .T. ) ;
#24544=LINE ( 'NONE', #21716, #768 ) ;
#24545=LINE ( 'NONE', #2148, #22528 ) ;
#24548=FACE_OUTER_BOUND ( 'NONE', #30929, .T. ) ;
#24549=ADVANCED_FACE ( 'NONE', ( #31957 ), #7220, .T. ) ;
#24555=AXIS2_PLACEMENT_3D ( 'NONE', #18499, #29337, #31641 ) ;
#24564=CARTESIAN_POINT ( 'NONE',  ( -11.99999999999998224, -134.9999999999999716, 155.0000000000000000 ) ) ;
#24573=FACE_OUTER_BOUND ( 'NONE', #21629, .T. ) ;
#24576=LINE ( 'NONE', #21928, #30919 ) ;
#24577=ORIENTED_EDGE ( 'NONE', *, *, #14292, .F. ) ;
#24582=VECTOR ( 'NONE', #4318, 1000.000000000000000 ) ;
#24584=EDGE_CURVE ( 'NONE', #24075, #8817, #16140, .T. ) ;
#24589=DIRECTION ( 'NONE',  ( 1.000000000000000000, 0.000000000000000000, 0.000000000000000000 ) ) ;
#24598=EDGE_LOOP ( 'NONE', ( #31200, #10221, #5987, #9630 ) ) ;
#24599=ADVANCED_FACE ( 'NONE', ( #18462 ), #7568, .F. ) ;
#24604=ORIENTED_EDGE ( 'NONE', *, *, #6017, .F. ) ;
#24605=PLANE ( 'NONE',  #5908 ) ;
#24610=DIRECTION ( 'NONE',  ( -1.232595164407830946E-32, 0.000000000000000000, -1.000000000000000000 ) ) ;
#24611=DIRECTION ( 'NONE',  ( -0.000000000000000000, 1.310824597558155437E-49, 1.000000000000000000 ) ) ;
#24612=EDGE_LOOP ( 'NONE', ( #23568, #31543, #10074, #24861, #242, #22109, #29073, #27549 ) ) ;
#24615=EDGE_CURVE ( 'NONE', #27476, #19297, #21147, .T. ) ;
#24619=ORIENTED_EDGE ( 'NONE', *, *, #3289, .T. ) ;
#24623=VERTEX_POINT ( 'NONE', #281 ) ;
#24628=CARTESIAN_POINT ( 'NONE',  ( -19.99999999999998934, 144.9999999999999716, 187.0000000000000000 ) ) ;
#24633=EDGE_LOOP ( 'NONE', ( #32939, #23117, #18182, #14775 ) ) ;
#24640=DIRECTION ( 'NONE',  ( 0.000000000000000000, 0.000000000000000000, -1.000000000000000000 ) ) ;
#24644=EDGE_LOOP ( 'NONE', ( #5567, #8973, #24338, #16519 ) ) ;
#24648=ORIENTED_EDGE ( 'NONE', *, *, #20187, .T. ) ;
#24653=DIRECTION ( 'NONE',  ( 0.000000000000000000, 1.000000000000000000, 1.224646799147353207E-16 ) ) ;
#24655=LINE ( 'NONE', #3128, #34062 ) ;
#24656=AXIS2_PLACEMENT_3D ( 'NONE', #25308, #11976, #9111 ) ;
#24659=ORIENTED_EDGE ( 'NONE', *, *, #10044, .T. ) ;
#24661=CIRCLE ( 'NONE', #7030, 3.999999999999976019 ) ;
#24662=CARTESIAN_POINT ( 'NONE',  ( -20.00000000000001776, -113.0000000000000000, 187.0000000000000000 ) ) ;
#24663=CARTESIAN_POINT ( 'NONE',  ( -418.0000000000000568, 104.9999999999999858, -159.0000000000000000 ) ) ;
#24664=LINE ( 'NONE', #18487, #11814 ) ;
#24666=DIRECTION ( 'NONE',  ( -1.000000000000000000, 0.000000000000000000, 0.000000000000000000 ) ) ;
#24673=CARTESIAN_POINT ( 'NONE',  ( 19.99999999999998934, 124.9999999999999716, 162.9999999999999716 ) ) ;
#24675=AXIS2_PLACEMENT_3D ( 'NONE', #31967, #10262, #21121 ) ;
#24683=EDGE_LOOP ( 'NONE', ( #23851, #727, #12843, #31424 ) ) ;
#24685=MANIFOLD_SOLID_BREP ( 'Trim/Extend3[2]', #20037 ) ;
#24686=DIRECTION ( 'NONE',  ( 0.000000000000000000, -1.000000000000000000, -5.145227585319922065E-49 ) ) ;
#24687=CARTESIAN_POINT ( 'NONE',  ( -365.0000000000000000, -119.0000000000000000, 111.9999999999999858 ) ) ;
#24690=ORIENTED_EDGE ( 'NONE', *, *, #9611, .F. ) ;
#24694=LINE ( 'NONE', #19037, #16143 ) ;
#24698=DIRECTION ( 'NONE',  ( 0.000000000000000000, -1.131431318426415506E-52, -1.000000000000000000 ) ) ;
#24700=VECTOR ( 'NONE', #10397, 1000.000000000000000 ) ;
#24706=ORIENTED_EDGE ( 'NONE', *, *, #1025, .T. ) ;
#24707=FACE_OUTER_BOUND ( 'NONE', #4338, .T. ) ;
#24709=EDGE_CURVE ( 'NONE', #5991, #5794, #6128, .T. ) ;
#24711=PLANE ( 'NONE',  #7068 ) ;
#24713=VECTOR ( 'NONE', #11356, 1000.000000000000000 ) ;
#24719=FACE_OUTER_BOUND ( 'NONE', #25234, .T. ) ;
#24720=DIRECTION ( 'NONE',  ( -1.000000000000000000, 0.000000000000000000, -1.292961597001347186E-16 ) ) ;
#24724=DIRECTION ( 'NONE',  ( -5.546364386991661285E-52, 0.000000000000000000, -1.000000000000000000 ) ) ;
#24727=DIRECTION ( 'NONE',  ( 0.000000000000000000, 1.000000000000000000, 1.224646799147353207E-16 ) ) ;
#24731=CIRCLE ( 'NONE', #33842, 7.999999999999979572 ) ;
#24733=CARTESIAN_POINT ( 'NONE',  ( -19.99999999999998934, 4.559999999999909015, -168.2400000000000091 ) ) ;
#24739=CIRCLE ( 'NONE', #9419, 7.999999999999986677 ) ;
#24743=ORIENTED_EDGE ( 'NONE', *, *, #4995, .T. ) ;
#24745=ORIENTED_EDGE ( 'NONE', *, *, #15158, .T. ) ;
#24746=EDGE_CURVE ( 'NONE', #20661, #11247, #1257, .T. ) ;
#24751=EDGE_LOOP ( 'NONE', ( #5772, #9179, #2050, #2276 ) ) ;
#24752=CARTESIAN_POINT ( 'NONE',  ( 15.99999999999998579, 144.9999999999999716, 187.0000000000000000 ) ) ;
#24753=CYLINDRICAL_SURFACE ( 'NONE', #27244, 7.999999999999979572 ) ;
#24756=DIRECTION ( 'NONE',  ( 1.000000000000000000, 3.040835319149746090E-31, -1.232595164407830946E-32 ) ) ;
#24757=VERTEX_POINT ( 'NONE', #27498 ) ;
#24764=ADVANCED_FACE ( 'NONE', ( #16849 ), #22167, .F. ) ;
#24768=CARTESIAN_POINT ( 'NONE',  ( -12.00000000000001066, 144.9999999999999716, -194.9999999999999432 ) ) ;
#24770=ORIENTED_EDGE ( 'NONE', *, *, #16300, .F. ) ;
#24773=DIRECTION ( 'NONE',  ( 0.000000000000000000, 1.131431318426415506E-52, 1.000000000000000000 ) ) ;
#24774=DIRECTION ( 'NONE',  ( 1.000000000000000000, 0.000000000000000000, 0.000000000000000000 ) ) ;
#24778=ADVANCED_FACE ( 'NONE', ( #15645 ), #29154, .T. ) ;
#24779=LINE ( 'NONE', #411, #18443 ) ;
#24780=VERTEX_POINT ( 'NONE', #7959 ) ;
#24785=ORIENTED_EDGE ( 'NONE', *, *, #8060, .F. ) ;
#24789=EDGE_CURVE ( 'NONE', #22615, #11675, #12143, .T. ) ;
#24791=CYLINDRICAL_SURFACE ( 'NONE', #25256, 7.999999999999979572 ) ;
#24792=ORIENTED_EDGE ( 'NONE', *, *, #21309, .F. ) ;
#24794=DIRECTION ( 'NONE',  ( 0.000000000000000000, 0.000000000000000000, -1.000000000000000000 ) ) ;
#24799=ORIENTED_EDGE ( 'NONE', *, *, #21557, .F. ) ;
#24801=CARTESIAN_POINT ( 'NONE',  ( -500.0000000000000000, -105.0000000000000142, 187.0000000000000000 ) ) ;
#24803=DIRECTION ( 'NONE',  ( -1.000000000000000000, 0.000000000000000000, 0.000000000000000000 ) ) ;
#24805=VECTOR ( 'NONE', #32767, 1000.000000000000000 ) ;
#24807=DIRECTION ( 'NONE',  ( 1.000000000000000000, 0.000000000000000000, 1.300283923313630633E-47 ) ) ;
#24808=ORIENTED_EDGE ( 'NONE', *, *, #9330, .F. ) ;
#24813=LINE ( 'NONE', #19675, #24828 ) ;
#24817=EDGE_CURVE ( 'NONE', #24914, #19693, #4570, .T. ) ;
#24819=VERTEX_POINT ( 'NONE', #29680 ) ;
#24820=FACE_OUTER_BOUND ( 'NONE', #23115, .T. ) ;
#24821=DIRECTION ( 'NONE',  ( -2.154935995002245207E-17, -0.000000000000000000, -1.000000000000000000 ) ) ;
#24825=VERTEX_POINT ( 'NONE', #34675 ) ;
#24828=VECTOR ( 'NONE', #14156, 1000.000000000000000 ) ;
#24829=EDGE_LOOP ( 'NONE', ( #31262, #34138, #9820, #11732 ) ) ;
#24831=AXIS2_PLACEMENT_3D ( 'NONE', #8161, #8346, #27212 ) ;
#24834=CARTESIAN_POINT ( 'NONE',  ( -70.00000000000000000, 75.55999999999990280, 172.9900000000000091 ) ) ;
#24839=CARTESIAN_POINT ( 'NONE',  ( 11.99999999999999645, 144.9999999999999716, 187.0000000000000000 ) ) ;
#24840=DIRECTION ( 'NONE',  ( -1.000000000000000000, 0.000000000000000000, -5.546364386991661285E-52 ) ) ;
#24841=VERTEX_POINT ( 'NONE', #21501 ) ;
#24842=ORIENTED_EDGE ( 'NONE', *, *, #1007, .T. ) ;
#24843=FACE_OUTER_BOUND ( 'NONE', #17222, .T. ) ;
#24844=CARTESIAN_POINT ( 'NONE',  ( 15.99999999999998579, 75.55999999999990280, 172.9900000000000091 ) ) ;
#24845=DIRECTION ( 'NONE',  ( 0.000000000000000000, 1.000000000000000000, 5.145227585319922065E-49 ) ) ;
#24846=CARTESIAN_POINT ( 'NONE',  ( -418.0000000000000000, -112.9999999999999858, 155.0000000000000000 ) ) ;
#24851=ORIENTED_EDGE ( 'NONE', *, *, #21412, .F. ) ;
#24852=DIRECTION ( 'NONE',  ( -0.000000000000000000, 1.000000000000000000, -0.000000000000000000 ) ) ;
#24856=ORIENTED_EDGE ( 'NONE', *, *, #4286, .T. ) ;
#24857=AXIS2_PLACEMENT_3D ( 'NONE', #1487, #18059, #15025 ) ;
#24859=EDGE_CURVE ( 'NONE', #24256, #4948, #31385, .T. ) ;
#24860=DIRECTION ( 'NONE',  ( 1.000000000000000000, 0.000000000000000000, 0.000000000000000000 ) ) ;
#24861=ORIENTED_EDGE ( 'NONE', *, *, #21204, .F. ) ;
#24862=CARTESIAN_POINT ( 'NONE',  ( -418.0000000000000000, 124.9999999999999574, -190.9999999999999716 ) ) ;
#24864=VECTOR ( 'NONE', #6721, 1000.000000000000000 ) ;
#24866=CARTESIAN_POINT ( 'NONE',  ( -410.0000000000000568, -105.0000000000000142, 187.0000000000000000 ) ) ;
#24867=CARTESIAN_POINT ( 'NONE',  ( -12.00000000000001066, 124.9999999999999716, 159.0000000000000000 ) ) ;
#24868=DIRECTION ( 'NONE',  ( 0.000000000000000000, 1.000000000000000000, -3.374343856708137958E-53 ) ) ;
#24869=VERTEX_POINT ( 'NONE', #21325 ) ;
#24870=VECTOR ( 'NONE', #9493, 1000.000000000000000 ) ;
#24874=LINE ( 'NONE', #862, #18986 ) ;
#24875=DIRECTION ( 'NONE',  ( -3.469446951953832974E-18, -1.000000000000000000, -7.888609052210116302E-31 ) ) ;
#24876=CIRCLE ( 'NONE', #8958, 2.000000000000001776 ) ;
#24877=AXIS2_PLACEMENT_3D ( 'NONE', #16927, #365, #2840 ) ;
#24883=CARTESIAN_POINT ( 'NONE',  ( -442.0000000000000000, -145.0000000000000000, -175.0000000000000000 ) ) ;
#24886=DIRECTION ( 'NONE',  ( -1.000000000000000000, 0.000000000000000000, -1.300283923313630633E-47 ) ) ;
#24890=EDGE_LOOP ( 'NONE', ( #9625, #21202, #4052, #8868, #22165, #21349, #4028, #17720 ) ) ;
#24891=ADVANCED_FACE ( 'NONE', ( #33841 ), #1916, .F. ) ;
#24892=DIRECTION ( 'NONE',  ( 0.000000000000000000, 0.000000000000000000, 1.000000000000000000 ) ) ;
#24893=DIRECTION ( 'NONE',  ( 0.000000000000000000, 0.000000000000000000, 1.000000000000000000 ) ) ;
#24895=ORIENTED_EDGE ( 'NONE', *, *, #22833, .T. ) ;
#24898=FACE_OUTER_BOUND ( 'NONE', #18379, .T. ) ;
#24899=ORIENTED_EDGE ( 'NONE', *, *, #21266, .T. ) ;
#24903=FACE_OUTER_BOUND ( 'NONE', #3419, .T. ) ;
#24904=CARTESIAN_POINT ( 'NONE',  ( -499.9999999999999432, -113.0000000000000000, -187.0000000000000000 ) ) ;
#24909=DIRECTION ( 'NONE',  ( 1.000000000000000000, 0.000000000000000000, 0.000000000000000000 ) ) ;
#24914=VERTEX_POINT ( 'NONE', #12802 ) ;
#24915=EDGE_LOOP ( 'NONE', ( #1583, #23571, #30834, #22838, #23233, #13031, #777, #17694 ) ) ;
#24920=ORIENTED_EDGE ( 'NONE', *, *, #11341, .F. ) ;
#24924=DIRECTION ( 'NONE',  ( 1.000000000000000000, 0.000000000000000000, 0.000000000000000000 ) ) ;
#24929=ADVANCED_FACE ( 'NONE', ( #21143, #31990 ), #20797, .T. ) ;
#24934=VECTOR ( 'NONE', #19711, 1000.000000000000000 ) ;
#24936=DIRECTION ( 'NONE',  ( 1.848892746611746966E-32, -6.842277657836020854E-49, 1.000000000000000000 ) ) ;
#24937=CARTESIAN_POINT ( 'NONE',  ( -365.0000000000000000, -131.0000000000000000, 130.0000000000000000 ) ) ;
#24939=EDGE_CURVE ( 'NONE', #30502, #6669, #4931, .T. ) ;
#24941=CARTESIAN_POINT ( 'NONE',  ( -355.0000000000000000, 130.9999999999999716, 113.9999999999999858 ) ) ;
#24946=AXIS2_PLACEMENT_3D ( 'NONE', #4002, #23410, #3661 ) ;
#24952=DIRECTION ( 'NONE',  ( 0.000000000000000000, 0.000000000000000000, -1.000000000000000000 ) ) ;
#24953=EDGE_CURVE ( 'NONE', #14854, #30600, #664, .T. ) ;
#24957=VERTEX_POINT ( 'NONE', #16522 ) ;
#24961=ORIENTED_EDGE ( 'NONE', *, *, #10492, .T. ) ;
#24962=ORIENTED_EDGE ( 'NONE', *, *, #7210, .F. ) ;
#24968=LINE ( 'NONE', #22140, #19420 ) ;
#24970=ORIENTED_EDGE ( 'NONE', *, *, #21600, .F. ) ;
#24974=DIRECTION ( 'NONE',  ( 0.000000000000000000, 0.000000000000000000, 1.000000000000000000 ) ) ;
#24975=DIRECTION ( 'NONE',  ( 0.000000000000000000, -0.000000000000000000, 1.000000000000000000 ) ) ;
#24982=CARTESIAN_POINT ( 'NONE',  ( -442.0000000000000000, -104.9999999999999716, -187.0000000000000000 ) ) ;
#24986=EDGE_CURVE ( 'NONE', #493, #591, #18368, .T. ) ;
#24988=CARTESIAN_POINT ( 'NONE',  ( -418.0000000000000000, -105.0000000000000142, 155.0000000000000000 ) ) ;
#24992=ORIENTED_EDGE ( 'NONE', *, *, #22059, .T. ) ;
#24997=ADVANCED_FACE ( 'NONE', ( #10989 ), #32695, .T. ) ;
#25000=DIRECTION ( 'NONE',  ( 1.000000000000000000, -0.000000000000000000, -0.000000000000000000 ) ) ;
#25002=ORIENTED_EDGE ( 'NONE', *, *, #20580, .F. ) ;
#25008=EDGE_CURVE ( 'NONE', #392, #5864, #16699, .T. ) ;
#25012=VERTEX_POINT ( 'NONE', #2965 ) ;
#25016=ADVANCED_FACE ( 'NONE', ( #13489 ), #22024, .T. ) ;
#25017=DIRECTION ( 'NONE',  ( 0.000000000000000000, 5.145227585319922065E-49, 1.000000000000000000 ) ) ;
#25018=CARTESIAN_POINT ( 'NONE',  ( -410.0000000000000568, 105.0000000000000000, 132.0000000000000000 ) ) ;
#25020=DIRECTION ( 'NONE',  ( -0.000000000000000000, 0.000000000000000000, 1.000000000000000000 ) ) ;
#25021=ORIENTED_EDGE ( 'NONE', *, *, #17689, .F. ) ;
#25022=DIRECTION ( 'NONE',  ( 1.000000000000000000, 0.000000000000000000, 0.000000000000000000 ) ) ;
#25025=ORIENTED_EDGE ( 'NONE', *, *, #33140, .F. ) ;
#25027=DIRECTION ( 'NONE',  ( 0.000000000000000000, -1.000000000000000000, -5.145227585319922065E-49 ) ) ;
#25030=CARTESIAN_POINT ( 'NONE',  ( -414.0000000000000568, -105.0000000000000142, -77.99999999999997158 ) ) ;
#25032=VECTOR ( 'NONE', #15628, 1000.000000000000000 ) ;
#25038=AXIS2_PLACEMENT_3D ( 'NONE', #6106, #33350, #8971 ) ;
#25043=ORIENTED_EDGE ( 'NONE', *, *, #11464, .T. ) ;
#25045=EDGE_CURVE ( 'NONE', #2161, #2852, #8491, .T. ) ;
#25047=FACE_BOUND ( 'NONE', #19848, .T. ) ;
#25057=ORIENTED_EDGE ( 'NONE', *, *, #17632, .F. ) ;
#25060=ORIENTED_EDGE ( 'NONE', *, *, #26759, .T. ) ;
#25061=EDGE_CURVE ( 'NONE', #13784, #31329, #20069, .T. ) ;
#25062=FACE_OUTER_BOUND ( 'NONE', #16582, .T. ) ;
#25065=ORIENTED_EDGE ( 'NONE', *, *, #28804, .T. ) ;
#25067=VECTOR ( 'NONE', #19401, 1000.000000000000000 ) ;
#25068=VECTOR ( 'NONE', #23340, 1000.000000000000000 ) ;
#25071=ORIENTED_EDGE ( 'NONE', *, *, #14727, .F. ) ;
#25072=VECTOR ( 'NONE', #24773, 1000.000000000000000 ) ;
#25073=DIRECTION ( 'NONE',  ( -0.000000000000000000, -1.000000000000000000, -0.000000000000000000 ) ) ;
#25078=DIRECTION ( 'NONE',  ( 0.000000000000000000, -1.000000000000000000, 6.123233995736766036E-17 ) ) ;
#25080=ADVANCED_FACE ( 'NONE', ( #17586 ), #9197, .F. ) ;
#25081=CARTESIAN_POINT ( 'NONE',  ( -445.9999999999999432, 105.0000000000000142, 187.0000000000000000 ) ) ;
#25087=ORIENTED_EDGE ( 'NONE', *, *, #26719, .T. ) ;
#25089=ADVANCED_FACE ( 'NONE', ( #1186 ), #9024, .F. ) ;
#25092=CIRCLE ( 'NONE', #34200, 7.999999999999979572 ) ;
#25095=ORIENTED_EDGE ( 'NONE', *, *, #8840, .T. ) ;
#25097=DIRECTION ( 'NONE',  ( 1.000000000000000000, 0.000000000000000000, 0.000000000000000000 ) ) ;
#25100=CARTESIAN_POINT ( 'NONE',  ( 19.99999999999998224, -115.0000000000000000, -158.9999999999999716 ) ) ;
#25101=VERTEX_POINT ( 'NONE', #14738 ) ;
#25102=VERTEX_POINT ( 'NONE', #12409 ) ;
#25104=CARTESIAN_POINT ( 'NONE',  ( -442.0000000000000000, 137.0000000000000000, -175.0000000000000000 ) ) ;
#25105=CARTESIAN_POINT ( 'NONE',  ( -499.9999999999999432, 144.9999999999999716, -187.0000000000000000 ) ) ;
#25108=AXIS2_PLACEMENT_3D ( 'NONE', #29140, #9750, #23634 ) ;
#25114=ORIENTED_EDGE ( 'NONE', *, *, #30669, .F. ) ;
#25116=CARTESIAN_POINT ( 'NONE',  ( -499.9999999999999432, 112.9999999999999574, 187.0000000000000000 ) ) ;
#25118=VECTOR ( 'NONE', #4065, 1000.000000000000000 ) ;
#25123=FACE_OUTER_BOUND ( 'NONE', #9517, .T. ) ;
#25126=DIRECTION ( 'NONE',  ( 1.000000000000000000, 0.000000000000000000, -1.232595164407831220E-32 ) ) ;
#25127=ORIENTED_EDGE ( 'NONE', *, *, #25267, .F. ) ;
#25128=ADVANCED_FACE ( 'NONE', ( #9380, #25560 ), #25924, .T. ) ;
#25129=ORIENTED_EDGE ( 'NONE', *, *, #32215, .F. ) ;
#25133=PLANE ( 'NONE',  #9344 ) ;
#25137=DIRECTION ( 'NONE',  ( 1.000000000000000000, 0.000000000000000000, -1.848892746611746966E-32 ) ) ;
#25141=ORIENTED_EDGE ( 'NONE', *, *, #17734, .F. ) ;
#25142=LINE ( 'NONE', #4641, #23767 ) ;
#25143=AXIS2_PLACEMENT_3D ( 'NONE', #6738, #28110, #31297 ) ;
#25144=LINE ( 'NONE', #19478, #12583 ) ;
#25146=AXIS2_PLACEMENT_3D ( 'NONE', #51, #10917, #32611 ) ;
#25148=VECTOR ( 'NONE', #31944, 1000.000000000000000 ) ;
#25151=ADVANCED_FACE ( 'NONE', ( #23260 ), #34099, .F. ) ;
#25154=CYLINDRICAL_SURFACE ( 'NONE', #9748, 4.000000000000003553 ) ;
#25155=VERTEX_POINT ( 'NONE', #11887 ) ;
#25156=EDGE_CURVE ( 'NONE', #34303, #12264, #30565, .T. ) ;
#25157=DIRECTION ( 'NONE',  ( 0.000000000000000000, 0.000000000000000000, 1.000000000000000000 ) ) ;
#25163=LINE ( 'NONE', #17546, #17263 ) ;
#25167=CARTESIAN_POINT ( 'NONE',  ( -15.99999999999998579, 4.559999999999908127, -177.7400000000000091 ) ) ;
#25168=FACE_OUTER_BOUND ( 'NONE', #4336, .T. ) ;
#25169=DIRECTION ( 'NONE',  ( -0.000000000000000000, 1.000000000000000000, -0.000000000000000000 ) ) ;
#25171=AXIS2_PLACEMENT_3D ( 'NONE', #30737, #21458, #29112 ) ;
#25172=VERTEX_POINT ( 'NONE', #14381 ) ;
#25174=AXIS2_PLACEMENT_3D ( 'NONE', #29425, #4846, #34237 ) ;
#25185=AXIS2_PLACEMENT_3D ( 'NONE', #9329, #1323, #25879 ) ;
#25187=DIRECTION ( 'NONE',  ( -1.848892746611746966E-32, 6.842277657836020854E-49, -1.000000000000000000 ) ) ;
#25188=EDGE_CURVE ( 'NONE', #20076, #20682, #28570, .T. ) ;
#25191=EDGE_LOOP ( 'NONE', ( #13247, #1953, #3292, #16726, #14127, #24014, #21539, #11604 ) ) ;
#25199=VECTOR ( 'NONE', #1329, 1000.000000000000000 ) ;
#25203=DIRECTION ( 'NONE',  ( 0.000000000000000000, 2.309213040847544338E-50, 1.000000000000000000 ) ) ;
#25204=CARTESIAN_POINT ( 'NONE',  ( -418.0000000000000000, 105.0000000000000142, 194.9999999999999716 ) ) ;
#25205=EDGE_CURVE ( 'NONE', #27282, #23416, #7381, .T. ) ;
#25207=ORIENTED_EDGE ( 'NONE', *, *, #25061, .F. ) ;
#25209=ORIENTED_EDGE ( 'NONE', *, *, #10348, .T. ) ;
#25210=DIRECTION ( 'NONE',  ( 1.000000000000000000, 3.040835319149746090E-31, 1.232595164407830946E-32 ) ) ;
#25211=DIRECTION ( 'NONE',  ( 1.000000000000000000, 0.000000000000000000, 0.000000000000000000 ) ) ;
#25219=EDGE_LOOP ( 'NONE', ( #665, #19253, #15979 ) ) ;
#25224=CARTESIAN_POINT ( 'NONE',  ( -418.0000000000000000, -125.0000000000000000, 107.9999999999999858 ) ) ;
#25227=CARTESIAN_POINT ( 'NONE',  ( 19.99999999999998934, 75.55999999999990280, -177.7400000000000091 ) ) ;
#25230=EDGE_CURVE ( 'NONE', #27211, #13630, #12575, .T. ) ;
#25233=ORIENTED_EDGE ( 'NONE', *, *, #11055, .F. ) ;
#25234=EDGE_LOOP ( 'NONE', ( #16965, #19513, #32451, #1141 ) ) ;
#25235=ADVANCED_FACE ( 'NONE', ( #29293, #20757, #31603 ), #18273, .T. ) ;
#25236=LINE ( 'NONE', #19746, #23942 ) ;
#25238=CARTESIAN_POINT ( 'NONE',  ( -355.0000000000000000, 118.9999999999999716, 113.9999999999999858 ) ) ;
#25241=ORIENTED_EDGE ( 'NONE', *, *, #24939, .F. ) ;
#25244=AXIS2_PLACEMENT_3D ( 'NONE', #734, #28138, #33472 ) ;
#25245=CARTESIAN_POINT ( 'NONE',  ( -442.0000000000000000, 141.0000000000000000, 154.9999999999999716 ) ) ;
#25248=ORIENTED_EDGE ( 'NONE', *, *, #15022, .F. ) ;
#25251=VECTOR ( 'NONE', #32566, 1000.000000000000000 ) ;
#25252=CARTESIAN_POINT ( 'NONE',  ( -414.0000000000000568, 105.0000000000000142, 107.9999999999999858 ) ) ;
#25256=AXIS2_PLACEMENT_3D ( 'NONE', #32620, #13598, #10925 ) ;
#25257=CARTESIAN_POINT ( 'NONE',  ( -418.0000000000000000, -124.9999999999999716, 135.9999999999999716 ) ) ;
#25258=EDGE_CURVE ( 'NONE', #14266, #7431, #34634, .T. ) ;
#25259=CARTESIAN_POINT ( 'NONE',  ( -442.0000000000000000, -112.9999999999999858, 155.0000000000000000 ) ) ;
#25260=EDGE_CURVE ( 'NONE', #20441, #14635, #13278, .T. ) ;
#25262=DIRECTION ( 'NONE',  ( -1.000000000000000000, -3.469446951953834515E-18, 0.000000000000000000 ) ) ;
#25263=CARTESIAN_POINT ( 'NONE',  ( -499.9999999999999432, 140.9999999999999716, -162.9999999999999716 ) ) ;
#25265=VERTEX_POINT ( 'NONE', #10071 ) ;
#25267=EDGE_CURVE ( 'NONE', #6559, #29898, #34993, .T. ) ;
#25271=ORIENTED_EDGE ( 'NONE', *, *, #5243, .F. ) ;
#25272=VECTOR ( 'NONE', #1397, 1000.000000000000000 ) ;
#25276=CIRCLE ( 'NONE', #1979, 7.999999999999979572 ) ;
#25278=VECTOR ( 'NONE', #32521, 1000.000000000000000 ) ;
#25282=DIRECTION ( 'NONE',  ( 0.000000000000000000, 1.131431318426415506E-52, 1.000000000000000000 ) ) ;
#25283=CARTESIAN_POINT ( 'NONE',  ( -499.9999999999999432, 112.9999999999999574, 159.0000000000000000 ) ) ;
#25285=ORIENTED_EDGE ( 'NONE', *, *, #626, .F. ) ;
#25286=CYLINDRICAL_SURFACE ( 'NONE', #33329, 7.999999999999979572 ) ;
#25288=CARTESIAN_POINT ( 'NONE',  ( 11.99999999999999645, 144.9999999999999716, 162.9999999999999716 ) ) ;
#25290=CARTESIAN_POINT ( 'NONE',  ( -418.0000000000000000, 113.0000000000000000, 154.9999999999999716 ) ) ;
#25294=LINE ( 'NONE', #927, #6634 ) ;
#25296=ORIENTED_EDGE ( 'NONE', *, *, #25258, .T. ) ;
#25304=DIRECTION ( 'NONE',  ( 0.000000000000000000, 1.000000000000000000, 1.224646799147353207E-16 ) ) ;
#25307=UNCERTAINTY_MEASURE_WITH_UNIT (LENGTH_MEASURE( 1.000000000000000082E-05 ), #22116, 'distance_accuracy_value', 'NONE');
#25308=CARTESIAN_POINT ( 'NONE',  ( -12.00000000000001066, -137.0000000000000000, 174.9999999999999432 ) ) ;
#25309=CARTESIAN_POINT ( 'NONE',  ( -345.0000000000000000, -135.0000000000000000, 113.9999999999999858 ) ) ;
#25310=ORIENTED_EDGE ( 'NONE', *, *, #13303, .F. ) ;
#25312=FACE_OUTER_BOUND ( 'NONE', #3721, .T. ) ;
#25315=ORIENTED_EDGE ( 'NONE', *, *, #23910, .F. ) ;
#25319=ORIENTED_EDGE ( 'NONE', *, *, #234, .T. ) ;
#25321=FACE_OUTER_BOUND ( 'NONE', #4295, .T. ) ;
#25329=LINE ( 'NONE', #32810, #18669 ) ;
#25330=AXIS2_PLACEMENT_3D ( 'NONE', #11804, #11434, #3930 ) ;
#25333=DIRECTION ( 'NONE',  ( -1.000000000000000000, 0.000000000000000000, -5.546364386991661285E-52 ) ) ;
#25335=FACE_OUTER_BOUND ( 'NONE', #15009, .T. ) ;
#25338=PLANE ( 'NONE',  #25892 ) ;
#25340=EDGE_CURVE ( 'NONE', #17624, #7371, #26091, .T. ) ;
#25343=CARTESIAN_POINT ( 'NONE',  ( 11.99999999999999645, 124.9999999999999716, 162.9999999999999716 ) ) ;
#25344=CIRCLE ( 'NONE', #23103, 3.999999999999989786 ) ;
#25346=DIRECTION ( 'NONE',  ( -1.000000000000000000, 0.000000000000000000, -0.000000000000000000 ) ) ;
#25354=LINE ( 'NONE', #17204, #24504 ) ;
#25355=VECTOR ( 'NONE', #7566, 1000.000000000000000 ) ;
#25356=EDGE_CURVE ( 'NONE', #22871, #5175, #32540, .T. ) ;
#25357=VERTEX_POINT ( 'NONE', #2923 ) ;
#25358=VERTEX_POINT ( 'NONE', #24628 ) ;
#25360=ORIENTED_EDGE ( 'NONE', *, *, #3910, .T. ) ;
#25361=LINE ( 'NONE', #993, #29307 ) ;
#25364=CARTESIAN_POINT ( 'NONE',  ( -430.0000000000000000, 114.9999999999999716, 126.0000000000000000 ) ) ;
#25366=LINE ( 'NONE', #27511, #2776 ) ;
#25370=ORIENTED_EDGE ( 'NONE', *, *, #17441, .F. ) ;
#25373=FACE_OUTER_BOUND ( 'NONE', #31487, .T. ) ;
#25376=CYLINDRICAL_SURFACE ( 'NONE', #5044, 7.999999999999979572 ) ;
#25377=DIRECTION ( 'NONE',  ( 0.000000000000000000, -1.000000000000000000, -2.465190328815662439E-32 ) ) ;
#25378=PLANE ( 'NONE',  #21899 ) ;
#25379=LINE ( 'NONE', #17230, #11886 ) ;
#25380=ORIENTED_EDGE ( 'NONE', *, *, #31080, .F. ) ;
#25381=FACE_OUTER_BOUND ( 'NONE', #3996, .T. ) ;
#25383=ADVANCED_FACE ( 'NONE', ( #2750 ), #22159, .F. ) ;
#25386=DIRECTION ( 'NONE',  ( -0.000000000000000000, 1.000000000000000000, -0.000000000000000000 ) ) ;
#25387=VERTEX_POINT ( 'NONE', #24450 ) ;
#25389=DIRECTION ( 'NONE',  ( 1.000000000000000000, 0.000000000000000000, 0.000000000000000000 ) ) ;
#25392=VECTOR ( 'NONE', #22937, 1000.000000000000000 ) ;
#25395=EDGE_CURVE ( 'NONE', #10505, #5999, #31985, .T. ) ;
#25396=CARTESIAN_POINT ( 'NONE',  ( -500.0000000000000000, -105.0000000000000142, 187.0000000000000000 ) ) ;
#25397=FACE_OUTER_BOUND ( 'NONE', #8898, .T. ) ;
#25398=PLANE ( 'NONE',  #14380 ) ;
#25399=EDGE_CURVE ( 'NONE', #18391, #25708, #30154, .T. ) ;
#25410=ORIENTED_EDGE ( 'NONE', *, *, #30215, .T. ) ;
#25411=VERTEX_POINT ( 'NONE', #16841 ) ;
#25412=VERTEX_POINT ( 'NONE', #18795 ) ;
#25417=DIRECTION ( 'NONE',  ( 5.546364386991661285E-52, 0.000000000000000000, -1.000000000000000000 ) ) ;
#25419=AXIS2_PLACEMENT_3D ( 'NONE', #9468, #20153, #25823 ) ;
#25420=DIRECTION ( 'NONE',  ( 0.000000000000000000, 1.000000000000000000, 5.145227585319922065E-49 ) ) ;
#25425=ORIENTED_EDGE ( 'NONE', *, *, #10650, .F. ) ;
#25431=DIRECTION ( 'NONE',  ( 0.000000000000000000, 1.131431318426415506E-52, 1.000000000000000000 ) ) ;
#25432=VERTEX_POINT ( 'NONE', #5757 ) ;
#25434=CARTESIAN_POINT ( 'NONE',  ( -430.0000000000000000, -131.0000000000000000, 130.0000000000000000 ) ) ;
#25436=CIRCLE ( 'NONE', #8950, 7.999999999999979572 ) ;
#25449=VECTOR ( 'NONE', #9370, 1000.000000000000000 ) ;
#25451=LINE ( 'NONE', #11776, #29002 ) ;
#25453=DIRECTION ( 'NONE',  ( 0.000000000000000000, -1.131431318426415506E-52, -1.000000000000000000 ) ) ;
#25460=ORIENTED_EDGE ( 'NONE', *, *, #17386, .F. ) ;
#25463=EDGE_CURVE ( 'NONE', #22350, #31793, #25163, .T. ) ;
#25464=LINE ( 'NONE', #12137, #14790 ) ;
#25466=CARTESIAN_POINT ( 'NONE',  ( -418.0000000000000000, 137.0000000000000000, -175.0000000000000000 ) ) ;
#25472=ORIENTED_EDGE ( 'NONE', *, *, #13945, .T. ) ;
#25475=DIRECTION ( 'NONE',  ( 0.000000000000000000, 0.000000000000000000, 1.000000000000000000 ) ) ;
#25477=LINE ( 'NONE', #12150, #262 ) ;
#25479=EDGE_CURVE ( 'NONE', #19022, #26110, #3577, .T. ) ;
#25480=FACE_OUTER_BOUND ( 'NONE', #10990, .T. ) ;
#25481=CARTESIAN_POINT ( 'NONE',  ( -361.0000000000000000, -135.0000000000000000, 110.0000000000000000 ) ) ;
#25482=EDGE_LOOP ( 'NONE', ( #32728, #15133, #31973, #5839 ) ) ;
#25486=AXIS2_PLACEMENT_3D ( 'NONE', #5495, #3186, #14058 ) ;
#25490=AXIS2_PLACEMENT_3D ( 'NONE', #18134, #7402, #26114 ) ;
#25494=ORIENTED_EDGE ( 'NONE', *, *, #25008, .T. ) ;
#25496=VECTOR ( 'NONE', #34490, 1000.000000000000000 ) ;
#25499=EDGE_CURVE ( 'NONE', #29646, #22648, #20205, .T. ) ;
#25503=ORIENTED_EDGE ( 'NONE', *, *, #20323, .F. ) ;
#25506=DIRECTION ( 'NONE',  ( 0.000000000000000000, 5.053935297177146739E-49, 1.000000000000000000 ) ) ;
#25507=CARTESIAN_POINT ( 'NONE',  ( -418.0000000000000000, -105.0000000000000142, 155.0000000000000568 ) ) ;
#25509=DIRECTION ( 'NONE',  ( 0.000000000000000000, 0.000000000000000000, 1.000000000000000000 ) ) ;
#25512=CARTESIAN_POINT ( 'NONE',  ( 11.99999999999999645, -124.9999999999999432, -190.9999999999999432 ) ) ;
#25513=CIRCLE ( 'NONE', #19846, 3.999999999999976019 ) ;
#25516=DIRECTION ( 'NONE',  ( 0.000000000000000000, -1.224646799147353207E-16, 1.000000000000000000 ) ) ;
#25517=CARTESIAN_POINT ( 'NONE',  ( -442.0000000000000000, 104.9999999999999858, 154.9999999999999716 ) ) ;
#25525=CARTESIAN_POINT ( 'NONE',  ( -19.99999999999998934, -145.0000000000000000, 187.0000000000000000 ) ) ;
#25527=DIRECTION ( 'NONE',  ( 0.000000000000000000, -0.000000000000000000, -1.000000000000000000 ) ) ;
#25534=ORIENTED_EDGE ( 'NONE', *, *, #19098, .F. ) ;
#25536=ORIENTED_EDGE ( 'NONE', *, *, #20015, .F. ) ;
#25539=EDGE_CURVE ( 'NONE', #18640, #2780, #8130, .T. ) ;
#25540=DIRECTION ( 'NONE',  ( -1.000000000000000000, 0.000000000000000000, 0.000000000000000000 ) ) ;
#25543=EDGE_CURVE ( 'NONE', #10892, #30842, #793, .T. ) ;
#25547=VERTEX_POINT ( 'NONE', #3803 ) ;
#25548=LINE ( 'NONE', #1174, #23624 ) ;
#25552=DIRECTION ( 'NONE',  ( 1.000000000000000000, 0.000000000000000000, 0.000000000000000000 ) ) ;
#25555=CARTESIAN_POINT ( 'NONE',  ( -19.99999999999998934, -112.9999999999999858, 174.9999999999999432 ) ) ;
#25559=DIRECTION ( 'NONE',  ( 1.232595164407830946E-32, 0.000000000000000000, 1.000000000000000000 ) ) ;
#25560=FACE_OUTER_BOUND ( 'NONE', #21438, .T. ) ;
#25561=VERTEX_POINT ( 'NONE', #30866 ) ;
#25562=AXIS2_PLACEMENT_3D ( 'NONE', #14982, #16961, #31169 ) ;
#25563=FACE_OUTER_BOUND ( 'NONE', #17033, .T. ) ;
#25565=CARTESIAN_POINT ( 'NONE',  ( -418.0000000000000000, 105.0000000000000000, 139.9999999999999716 ) ) ;
#25567=ORIENTED_EDGE ( 'NONE', *, *, #1927, .F. ) ;
#25568=CARTESIAN_POINT ( 'NONE',  ( 11.99999999999999645, -137.0000000000000000, -155.0000000000000284 ) ) ;
#25571=ORIENTED_EDGE ( 'NONE', *, *, #13240, .T. ) ;
#25572=AXIS2_PLACEMENT_3D ( 'NONE', #23317, #12825, #26681 ) ;
#25574=EDGE_CURVE ( 'NONE', #33545, #15936, #30290, .T. ) ;
#25576=ORIENTED_EDGE ( 'NONE', *, *, #22232, .T. ) ;
#25577=PLANE ( 'NONE',  #17882 ) ;
#25579=ADVANCED_FACE ( 'NONE', ( #3625 ), #977, .T. ) ;
#25590=DIRECTION ( 'NONE',  ( 0.000000000000000000, 7.888609052210118054E-31, 1.000000000000000000 ) ) ;
#25592=CARTESIAN_POINT ( 'NONE',  ( -500.0000000000000000, -137.0000000000000000, 187.0000000000000000 ) ) ;
#25595=DIRECTION ( 'NONE',  ( 0.000000000000000000, 1.000000000000000000, -1.131431318426415506E-52 ) ) ;
#25596=CARTESIAN_POINT ( 'NONE',  ( 15.99999999999998579, -56.99999999999997868, 154.9999999999999716 ) ) ;
#25599=ADVANCED_FACE ( 'NONE', ( #34414 ), #7514, .T. ) ;
#25602=EDGE_CURVE ( 'NONE', #16746, #20411, #14412, .T. ) ;
#25604=CARTESIAN_POINT ( 'NONE',  ( 11.99999999999999645, -137.0000000000000000, 174.9999999999999432 ) ) ;
#25605=DIRECTION ( 'NONE',  ( 0.000000000000000000, -1.000000000000000000, -5.145227585319922065E-49 ) ) ;
#25607=CARTESIAN_POINT ( 'NONE',  ( -19.99999999999998934, 144.9999999999999716, -162.9999999999999432 ) ) ;
#25609=DIRECTION ( 'NONE',  ( 2.891205793294675861E-16, 0.000000000000000000, -1.000000000000000000 ) ) ;
#25613=UNCERTAINTY_MEASURE_WITH_UNIT (LENGTH_MEASURE( 1.000000000000000082E-05 ), #8063, 'distance_accuracy_value', 'NONE');
#25614=CARTESIAN_POINT ( 'NONE',  ( 12.00000000000003730, -55.00000000000000711, -154.9999999999999716 ) ) ;
#25615=LINE ( 'NONE', #18850, #18319 ) ;
#25619=AXIS2_PLACEMENT_3D ( 'NONE', #30903, #33744, #4003 ) ;
#25620=ORIENTED_EDGE ( 'NONE', *, *, #30090, .F. ) ;
#25621=AXIS2_PLACEMENT_3D ( 'NONE', #16110, #34792, #19134 ) ;
#25626=PLANE ( 'NONE',  #3693 ) ;
#25628=EDGE_CURVE ( 'NONE', #14577, #26553, #23215, .T. ) ;
#25629=CARTESIAN_POINT ( 'NONE',  ( -365.0000000000000000, -119.0000000000000000, 126.0000000000000000 ) ) ;
#25634=EDGE_CURVE ( 'NONE', #11675, #24819, #3019, .T. ) ;
#25635=EDGE_CURVE ( 'NONE', #6283, #3779, #23552, .T. ) ;
#25637=VECTOR ( 'NONE', #1625, 1000.000000000000000 ) ;
#25638=AXIS2_PLACEMENT_3D ( 'NONE', #4195, #7388, #31607 ) ;
#25639=DIRECTION ( 'NONE',  ( 0.000000000000000000, 5.145227585319922065E-49, 1.000000000000000000 ) ) ;
#25641=ORIENTED_EDGE ( 'NONE', *, *, #603, .T. ) ;
#25642=CARTESIAN_POINT ( 'NONE',  ( 11.99999999999999645, -145.0000000000000000, 187.0000000000000000 ) ) ;
#25648=EDGE_CURVE ( 'NONE', #21251, #12415, #31391, .T. ) ;
#25652=LINE ( 'NONE', #17325, #17977 ) ;
#25655=VERTEX_POINT ( 'NONE', #28721 ) ;
#25662=EDGE_CURVE ( 'NONE', #16454, #9586, #18945, .T. ) ;
#25663=CIRCLE ( 'NONE', #4023, 7.999999999999979572 ) ;
#25665=AXIS2_PLACEMENT_3D ( 'NONE', #16669, #14170, #30166 ) ;
#25666=AXIS2_PLACEMENT_3D ( 'NONE', #25116, #6241, #3580 ) ;
#25667=EDGE_CURVE ( 'NONE', #6969, #6974, #27451, .T. ) ;
#25668=ORIENTED_EDGE ( 'NONE', *, *, #25156, .T. ) ;
#25672=ORIENTED_EDGE ( 'NONE', *, *, #34636, .T. ) ;
#25675=CARTESIAN_POINT ( 'NONE',  ( -15.99999999999998579, 144.9999999999999716, -186.9999999999999716 ) ) ;
#25682=CARTESIAN_POINT ( 'NONE',  ( -355.0000000000000000, -114.9999999999999858, 126.0000000000000000 ) ) ;
#25683=LINE ( 'NONE', #17175, #3379 ) ;
#25684=LINE ( 'NONE', #6636, #26755 ) ;
#25685=CARTESIAN_POINT ( 'NONE',  ( -349.0000000000000000, -125.0000000000000284, 113.9999999999999858 ) ) ;
#25688=PLANE ( 'NONE',  #24857 ) ;
#25690=VECTOR ( 'NONE', #15643, 1000.000000000000000 ) ;
#25692=VERTEX_POINT ( 'NONE', #11266 ) ;
#25693=AXIS2_PLACEMENT_3D ( 'NONE', #8626, #5947, #27851 ) ;
#25695=CARTESIAN_POINT ( 'NONE',  ( 11.99999999999999645, -28.99999999999999645, -154.9999999999999716 ) ) ;
#25701=CARTESIAN_POINT ( 'NONE',  ( -12.00000000000001066, -105.0000000000000142, 155.0000000000000000 ) ) ;
#25702=ORIENTED_EDGE ( 'NONE', *, *, #23530, .F. ) ;
#25703=DIRECTION ( 'NONE',  ( -1.000000000000000000, 0.000000000000000000, 0.000000000000000000 ) ) ;
#25704=CARTESIAN_POINT ( 'NONE',  ( -500.0000000000000000, -145.0000000000000000, 162.9999999999999716 ) ) ;
#25708=VERTEX_POINT ( 'NONE', #26918 ) ;
#25711=ADVANCED_FACE ( 'NONE', ( #5541 ), #21589, .F. ) ;
#25715=VECTOR ( 'NONE', #31397, 1000.000000000000000 ) ;
#25716=VECTOR ( 'NONE', #21796, 1000.000000000000000 ) ;
#25717=EDGE_CURVE ( 'NONE', #22621, #32005, #3059, .T. ) ;
#25718=EDGE_LOOP ( 'NONE', ( #4635, #22267, #26226, #4035 ) ) ;
#25719=LINE ( 'NONE', #9170, #31009 ) ;
#25723=CARTESIAN_POINT ( 'NONE',  ( -12.00000000000001066, -124.9999999999999432, -194.9999999999999432 ) ) ;
#25724=CARTESIAN_POINT ( 'NONE',  ( -449.9999999999999432, -104.9999999999999858, -162.9999999999999716 ) ) ;
#25728=DIRECTION ( 'NONE',  ( 0.000000000000000000, 1.000000000000000000, 0.000000000000000000 ) ) ;
#25729=LINE ( 'NONE', #22545, #19208 ) ;
#25732=DIRECTION ( 'NONE',  ( 0.000000000000000000, 1.000000000000000000, -3.374343856708137958E-53 ) ) ;
#25738=DIRECTION ( 'NONE',  ( -1.000000000000000000, 0.000000000000000000, 0.000000000000000000 ) ) ;
#25739=DIRECTION ( 'NONE',  ( 0.000000000000000000, 0.000000000000000000, 1.000000000000000000 ) ) ;
#25742=AXIS2_PLACEMENT_3D ( 'NONE', #31691, #15171, #7302 ) ;
#25743=VECTOR ( 'NONE', #23421, 1000.000000000000000 ) ;
#25744=FACE_BOUND ( 'NONE', #17800, .T. ) ;
#25749=EDGE_CURVE ( 'NONE', #27971, #1594, #5858, .T. ) ;
#25751=ORIENTED_EDGE ( 'NONE', *, *, #7535, .F. ) ;
#25753=LINE ( 'NONE', #23271, #4057 ) ;
#25754=VERTEX_POINT ( 'NONE', #34948 ) ;
#25758=VERTEX_POINT ( 'NONE', #29270 ) ;
#25759=CARTESIAN_POINT ( 'NONE',  ( -19.99999999999998934, 112.9999999999999574, 155.0000000000000000 ) ) ;
#25761=DIRECTION ( 'NONE',  ( -0.000000000000000000, 1.000000000000000000, -0.000000000000000000 ) ) ;
#25763=CARTESIAN_POINT ( 'NONE',  ( -442.0000000000000000, -124.9999999999999858, -69.99999999999998579 ) ) ;
#25767=AXIS2_PLACEMENT_3D ( 'NONE', #28552, #14515, #28199 ) ;
#25771=DIRECTION ( 'NONE',  ( 0.000000000000000000, 1.000000000000000000, -6.123233995736766036E-17 ) ) ;
#25773=DIRECTION ( 'NONE',  ( 0.000000000000000000, 0.000000000000000000, 1.000000000000000000 ) ) ;
#25778=DIRECTION ( 'NONE',  ( 0.000000000000000000, 1.000000000000000000, 1.224646799147353207E-16 ) ) ;
#25779=CIRCLE ( 'NONE', #30329, 3.999999999999976019 ) ;
#25784=LINE ( 'NONE', #31140, #32491 ) ;
#25785=EDGE_CURVE ( 'NONE', #32015, #10470, #8575, .T. ) ;
#25786=PLANE ( 'NONE',  #10480 ) ;
#25788=EDGE_CURVE ( 'NONE', #15103, #25895, #4131, .T. ) ;
#25792=DIRECTION ( 'NONE',  ( 0.000000000000000000, -3.374343856708137958E-53, 1.000000000000000000 ) ) ;
#25793=FACE_OUTER_BOUND ( 'NONE', #29638, .T. ) ;
#25795=ORIENTED_EDGE ( 'NONE', *, *, #24497, .T. ) ;
#25800=EDGE_LOOP ( 'NONE', ( #1859, #34785, #34337, #20690 ) ) ;
#25801=ADVANCED_FACE ( 'NONE', ( #21414 ), #753, .F. ) ;
#25804=CARTESIAN_POINT ( 'NONE',  ( -15.99999999999998579, -112.9999999999999858, 174.9999999999999432 ) ) ;
#25811=FACE_OUTER_BOUND ( 'NONE', #19879, .T. ) ;
#25812=VECTOR ( 'NONE', #18369, 1000.000000000000000 ) ;
#25818=FACE_OUTER_BOUND ( 'NONE', #28385, .T. ) ;
#25823=DIRECTION ( 'NONE',  ( 0.000000000000000000, 0.000000000000000000, -1.000000000000000000 ) ) ;
#25827=CARTESIAN_POINT ( 'NONE',  ( 11.99999999999999645, -145.0000000000000000, 187.0000000000000000 ) ) ;
#25829=AXIS2_PLACEMENT_3D ( 'NONE', #13601, #13958, #24794 ) ;
#25835=EDGE_CURVE ( 'NONE', #196, #20661, #6071, .T. ) ;
#25836=CIRCLE ( 'NONE', #32074, 7.999999999999979572 ) ;
#25838=CIRCLE ( 'NONE', #19802, 7.999999999999979572 ) ;
#25843=VECTOR ( 'NONE', #229, 1000.000000000000000 ) ;
#25846=VECTOR ( 'NONE', #4386, 1000.000000000000000 ) ;
#25851=ORIENTED_EDGE ( 'NONE', *, *, #17871, .F. ) ;
#25852=CARTESIAN_POINT ( 'NONE',  ( -442.0000000000000000, 104.9999999999999858, -159.0000000000000000 ) ) ;
#25854=AXIS2_PLACEMENT_3D ( 'NONE', #5870, #27600, #3216 ) ;
#25857=CARTESIAN_POINT ( 'NONE',  ( 11.99999999999999645, 124.9999999999999716, 155.0000000000000000 ) ) ;
#25859=ORIENTED_EDGE ( 'NONE', *, *, #33547, .T. ) ;
#25860=ORIENTED_EDGE ( 'NONE', *, *, #6464, .T. ) ;
#25864=FACE_BOUND ( 'NONE', #4382, .T. ) ;
#25866=DIRECTION ( 'NONE',  ( 1.000000000000000000, 0.000000000000000000, 0.000000000000000000 ) ) ;
#25870=DIRECTION ( 'NONE',  ( 1.232595164407831220E-32, -3.421138828918010427E-49, 1.000000000000000000 ) ) ;
#25873=VECTOR ( 'NONE', #19074, 1000.000000000000000 ) ;
#25874=LINE ( 'NONE', #12362, #285 ) ;
#25876=MECHANICAL_DESIGN_GEOMETRIC_PRESENTATION_REPRESENTATION('',(#5405),#9964);
#25879=DIRECTION ( 'NONE',  ( 0.000000000000000000, 0.000000000000000000, 1.000000000000000000 ) ) ;
#25880=DIRECTION ( 'NONE',  ( 1.000000000000000000, 0.000000000000000000, 1.300283923313630633E-47 ) ) ;
#25881=DIRECTION ( 'NONE',  ( 1.000000000000000000, 0.000000000000000000, 0.000000000000000000 ) ) ;
#25883=CARTESIAN_POINT ( 'NONE',  ( -499.9999999999999432, 144.9999999999999716, -187.0000000000000000 ) ) ;
#25888=VECTOR ( 'NONE', #15239, 1000.000000000000000 ) ;
#25892=AXIS2_PLACEMENT_3D ( 'NONE', #23040, #9510, #1492 ) ;
#25894=VECTOR ( 'NONE', #10980, 1000.000000000000000 ) ;
#25895=VERTEX_POINT ( 'NONE', #577 ) ;
#25897=DIRECTION ( 'NONE',  ( 0.000000000000000000, 2.465190328815661892E-32, 1.000000000000000000 ) ) ;
#25898=ORIENTED_EDGE ( 'NONE', *, *, #19256, .F. ) ;
#25899=VERTEX_POINT ( 'NONE', #9108 ) ;
#25901=VECTOR ( 'NONE', #33139, 1000.000000000000000 ) ;
#25903=DIRECTION ( 'NONE',  ( -3.040835319149746528E-31, -1.000000000000000000, 0.000000000000000000 ) ) ;
#25904=CARTESIAN_POINT ( 'NONE',  ( -410.0000000000000568, -124.9999999999999858, -77.99999999999997158 ) ) ;
#25905=ORIENTED_EDGE ( 'NONE', *, *, #15122, .T. ) ;
#25906=EDGE_LOOP ( 'NONE', ( #17707, #31418, #29612, #16466 ) ) ;
#25911=CARTESIAN_POINT ( 'NONE',  ( -20.00000000000004619, -141.0000000000000000, -187.0000000000000000 ) ) ;
#25915=EDGE_CURVE ( 'NONE', #8469, #2370, #30339, .T. ) ;
#25916=VECTOR ( 'NONE', #33518, 1000.000000000000000 ) ;
#25918=DIRECTION ( 'NONE',  ( -0.000000000000000000, -0.000000000000000000, 1.000000000000000000 ) ) ;
#25919=EDGE_LOOP ( 'NONE', ( #24301, #6172, #3069, #34256 ) ) ;
#25920=CIRCLE ( 'NONE', #2583, 4.000000000000003553 ) ;
#25923=DIRECTION ( 'NONE',  ( 0.000000000000000000, -1.000000000000000000, -2.465190328815662439E-32 ) ) ;
#25924=PLANE ( 'NONE',  #4677 ) ;
#25929=CARTESIAN_POINT ( 'NONE',  ( -12.00000000000001066, -105.0000000000000142, 155.0000000000000000 ) ) ;
#25933=FACE_OUTER_BOUND ( 'NONE', #22347, .T. ) ;
#25934=FACE_OUTER_BOUND ( 'NONE', #9113, .T. ) ;
#25936=ORIENTED_EDGE ( 'NONE', *, *, #2767, .F. ) ;
#25937=AXIS2_PLACEMENT_3D ( 'NONE', #17830, #15150, #25990 ) ;
#25941=AXIS2_PLACEMENT_3D ( 'NONE', #8043, #32947, #11258 ) ;
#25946=ORIENTED_EDGE ( 'NONE', *, *, #33747, .T. ) ;
#25950=VECTOR ( 'NONE', #5201, 1000.000000000000000 ) ;
#25951=FACE_OUTER_BOUND ( 'NONE', #17869, .T. ) ;
#25954=FACE_OUTER_BOUND ( 'NONE', #23331, .T. ) ;
#25956=CARTESIAN_POINT ( 'NONE',  ( -442.0000000000000000, -125.0000000000000000, 187.0000000000000000 ) ) ;
#25957=DIRECTION ( 'NONE',  ( 1.000000000000000000, 0.000000000000000000, 1.300283923313630633E-47 ) ) ;
#25960=VECTOR ( 'NONE', #18544, 1000.000000000000000 ) ;
#25962=ORIENTED_EDGE ( 'NONE', *, *, #13519, .F. ) ;
#25965=VERTEX_POINT ( 'NONE', #26168 ) ;
#25966=DIRECTION ( 'NONE',  ( -1.000000000000000000, 0.000000000000000000, -5.546364386991661285E-52 ) ) ;
#25969=DIRECTION ( 'NONE',  ( 0.000000000000000000, 0.000000000000000000, -1.000000000000000000 ) ) ;
#25970=DIRECTION ( 'NONE',  ( 0.000000000000000000, 1.000000000000000000, 0.000000000000000000 ) ) ;
#25975=AXIS2_PLACEMENT_3D ( 'NONE', #6383, #17095, #3719 ) ;
#25984=AXIS2_PLACEMENT_3D ( 'NONE', #22013, #30555, #829 ) ;
#25990=DIRECTION ( 'NONE',  ( 0.000000000000000000, 0.000000000000000000, -1.000000000000000000 ) ) ;
#25991=VECTOR ( 'NONE', #27160, 1000.000000000000000 ) ;
#25995=ORIENTED_EDGE ( 'NONE', *, *, #2911, .T. ) ;
#25996=CARTESIAN_POINT ( 'NONE',  ( -361.0000000000000000, -125.0000000000000284, 181.0000000000000000 ) ) ;
#25997=VECTOR ( 'NONE', #11747, 1000.000000000000000 ) ;
#25999=AXIS2_PLACEMENT_3D ( 'NONE', #10053, #23757, #13259 ) ;
#26002=DIRECTION ( 'NONE',  ( 0.000000000000000000, -1.000000000000000000, 0.000000000000000000 ) ) ;
#26004=FACE_BOUND ( 'NONE', #34335, .T. ) ;
#26006=VECTOR ( 'NONE', #4923, 1000.000000000000000 ) ;
#26009=CARTESIAN_POINT ( 'NONE',  ( -12.00000000000001066, -137.0000000000000000, 174.9999999999999432 ) ) ;
#26012=LINE ( 'NONE', #29024, #14329 ) ;
#26015=VERTEX_POINT ( 'NONE', #4448 ) ;
#26017=AXIS2_PLACEMENT_3D ( 'NONE', #19476, #33160, #249 ) ;
#26018=DIRECTION ( 'NONE',  ( 1.000000000000000000, 0.000000000000000000, -0.000000000000000000 ) ) ;
#26019=VERTEX_POINT ( 'NONE', #23854 ) ;
#26032=FACE_OUTER_BOUND ( 'NONE', #5006, .T. ) ;
#26034=EDGE_CURVE ( 'NONE', #1780, #31407, #4277, .T. ) ;
#26036=DIRECTION ( 'NONE',  ( -0.000000000000000000, -1.000000000000000000, -0.000000000000000000 ) ) ;
#26037=LINE ( 'NONE', #14852, #3449 ) ;
#26041=PLANE ( 'NONE',  #8373 ) ;
#26042=LINE ( 'NONE', #23033, #27029 ) ;
#26044=DIRECTION ( 'NONE',  ( 1.000000000000000000, 0.000000000000000000, 0.000000000000000000 ) ) ;
#26045=ORIENTED_EDGE ( 'NONE', *, *, #17948, .T. ) ;
#26046=DIRECTION ( 'NONE',  ( 0.000000000000000000, -6.123233995736766036E-17, -1.000000000000000000 ) ) ;
#26047=DIRECTION ( 'NONE',  ( 1.000000000000000000, 0.000000000000000000, -1.848892746611746966E-32 ) ) ;
#26051=CARTESIAN_POINT ( 'NONE',  ( 12.00000000000001066, -32.99999999999997158, 154.9999999999999716 ) ) ;
#26055=VERTEX_POINT ( 'NONE', #6947 ) ;
#26058=LINE ( 'NONE', #29070, #2091 ) ;
#26060=ORIENTED_EDGE ( 'NONE', *, *, #25356, .T. ) ;
#26065=AXIS2_PLACEMENT_3D ( 'NONE', #14769, #28283, #21924 ) ;
#26076=CARTESIAN_POINT ( 'NONE',  ( -12.00000000000001066, 108.9999999999999858, 155.0000000000000000 ) ) ;
#26078=PLANE ( 'NONE',  #33381 ) ;
#26080=DIRECTION ( 'NONE',  ( -3.469446951953832974E-18, -1.000000000000000000, -7.888609052210116302E-31 ) ) ;
#26084=DIRECTION ( 'NONE',  ( -0.000000000000000000, -0.000000000000000000, -1.000000000000000000 ) ) ;
#26086=EDGE_CURVE ( 'NONE', #24757, #17376, #3045, .T. ) ;
#26087=CARTESIAN_POINT ( 'NONE',  ( -15.99999999999998579, -56.99999999999997868, -154.9999999999999716 ) ) ;
#26088=ORIENTED_EDGE ( 'NONE', *, *, #418, .T. ) ;
#26091=LINE ( 'NONE', #15424, #25743 ) ;
#26092=ORIENTED_EDGE ( 'NONE', *, *, #31883, .T. ) ;
#26094=VERTEX_POINT ( 'NONE', #10333 ) ;
#26098=EDGE_CURVE ( 'NONE', #30076, #7133, #21244, .T. ) ;
#26100=ORIENTED_EDGE ( 'NONE', *, *, #34140, .F. ) ;
#26101=DIRECTION ( 'NONE',  ( 0.000000000000000000, 0.000000000000000000, 1.000000000000000000 ) ) ;
#26108=VERTEX_POINT ( 'NONE', #18362 ) ;
#26110=VERTEX_POINT ( 'NONE', #34015 ) ;
#26111=CARTESIAN_POINT ( 'NONE',  ( -365.0000000000000000, -135.0000000000000000, 113.9999999999999858 ) ) ;
#26112=ADVANCED_FACE ( 'NONE', ( #9636 ), #17842, .F. ) ;
#26114=DIRECTION ( 'NONE',  ( 0.000000000000000000, 0.000000000000000000, -1.000000000000000000 ) ) ;
#26115=CARTESIAN_POINT ( 'NONE',  ( 19.99999999999996092, -134.9999999999999716, 187.0000000000000000 ) ) ;
#26116=DIRECTION ( 'NONE',  ( 0.000000000000000000, 1.000000000000000000, -3.374343856708137958E-53 ) ) ;
#26119=ORIENTED_EDGE ( 'NONE', *, *, #10434, .T. ) ;
#26120=CARTESIAN_POINT ( 'NONE',  ( -355.0000000000000000, -119.0000000000000000, 109.9999999999999858 ) ) ;
#26123=CIRCLE ( 'NONE', #28971, 4.000000000000003553 ) ;
#26124=CARTESIAN_POINT ( 'NONE',  ( -11.99999999999998224, -134.9999999999999716, 155.0000000000000000 ) ) ;
#26127=DIRECTION ( 'NONE',  ( 0.000000000000000000, -1.310824597558155437E-49, -1.000000000000000000 ) ) ;
#26128=ORIENTED_EDGE ( 'NONE', *, *, #27551, .F. ) ;
#26130=CARTESIAN_POINT ( 'NONE',  ( -442.0000000000000000, -125.0000000000000000, 100.0000000000000000 ) ) ;
#26132=LINE ( 'NONE', #17461, #18922 ) ;
#26133=EDGE_LOOP ( 'NONE', ( #23355, #14130, #33574, #22130 ) ) ;
#26134=PLANE ( 'NONE',  #10343 ) ;
#26137=FACE_OUTER_BOUND ( 'NONE', #13972, .T. ) ;
#26139=CARTESIAN_POINT ( 'NONE',  ( -500.0000000000000000, -113.0000000000000000, 187.0000000000000000 ) ) ;
#26142=EDGE_CURVE ( 'NONE', #8847, #19179, #10519, .T. ) ;
#26143=VERTEX_POINT ( 'NONE', #21376 ) ;
#26146=LINE ( 'NONE', #23479, #9577 ) ;
#26148=PLANE ( 'NONE',  #7372 ) ;
#26149=ORIENTED_EDGE ( 'NONE', *, *, #19572, .F. ) ;
#26150=EDGE_CURVE ( 'NONE', #30004, #28861, #21550, .T. ) ;
#26152=VECTOR ( 'NONE', #5128, 1000.000000000000000 ) ;
#26154=CARTESIAN_POINT ( 'NONE',  ( -20.00000000000004619, 112.9999999999999574, 194.9999999999999716 ) ) ;
#26157=DIRECTION ( 'NONE',  ( 0.000000000000000000, 5.145227585319922065E-49, 1.000000000000000000 ) ) ;
#26159=DIRECTION ( 'NONE',  ( 0.000000000000000000, 0.000000000000000000, -1.000000000000000000 ) ) ;
#26162=CARTESIAN_POINT ( 'NONE',  ( -12.00000000000001066, -56.99999999999997868, -175.0000000000000000 ) ) ;
#26163=VECTOR ( 'NONE', #28796, 1000.000000000000000 ) ;
#26166=DIRECTION ( 'NONE',  ( 0.000000000000000000, 0.000000000000000000, -1.000000000000000000 ) ) ;
#26168=CARTESIAN_POINT ( 'NONE',  ( -12.00000000000001066, -145.0000000000000000, 194.9999999999999716 ) ) ;
#26170=FACE_OUTER_BOUND ( 'NONE', #8300, .T. ) ;
#26174=VECTOR ( 'NONE', #28369, 1000.000000000000000 ) ;
#26178=EDGE_CURVE ( 'NONE', #15752, #21251, #24544, .T. ) ;
#26179=EDGE_CURVE ( 'NONE', #30076, #32798, #29728, .T. ) ;
#26196=ORIENTED_EDGE ( 'NONE', *, *, #17590, .F. ) ;
#26199=CARTESIAN_POINT ( 'NONE',  ( -442.0000000000000000, -137.0000000000000000, -155.0000000000000000 ) ) ;
#26202=DIRECTION ( 'NONE',  ( -1.000000000000000000, 0.000000000000000000, 0.000000000000000000 ) ) ;
#26203=CARTESIAN_POINT ( 'NONE',  ( 11.99999999999999645, 112.9999999999999574, 155.0000000000000000 ) ) ;
#26204=ORIENTED_EDGE ( 'NONE', *, *, #18517, .F. ) ;
#26208=DIRECTION ( 'NONE',  ( 0.000000000000000000, 0.000000000000000000, 1.000000000000000000 ) ) ;
#26214=CARTESIAN_POINT ( 'NONE',  ( -430.0000000000000000, 132.9999999999999716, 113.9999999999999858 ) ) ;
#26216=AXIS2_PLACEMENT_3D ( 'NONE', #15658, #28812, #29348 ) ;
#26217=EDGE_CURVE ( 'NONE', #12516, #1340, #19069, .T. ) ;
#26219=AXIS2_PLACEMENT_3D ( 'NONE', #5341, #11052, #29740 ) ;
#26222=CIRCLE ( 'NONE', #25666, 7.999999999999979572 ) ;
#26225=EDGE_CURVE ( 'NONE', #11787, #28629, #368, .T. ) ;
#26226=ORIENTED_EDGE ( 'NONE', *, *, #14075, .T. ) ;
#26230=AXIS2_PLACEMENT_3D ( 'NONE', #9658, #6977, #1996 ) ;
#26238=CIRCLE ( 'NONE', #13201, 7.999999999999979572 ) ;
#26240=AXIS2_PLACEMENT_3D ( 'NONE', #23596, #31602, #20924 ) ;
#26241=FACE_OUTER_BOUND ( 'NONE', #23760, .T. ) ;
#26242=ORIENTED_EDGE ( 'NONE', *, *, #34966, .T. ) ;
#26244=VECTOR ( 'NONE', #12585, 1000.000000000000000 ) ;
#26246=FACE_OUTER_BOUND ( 'NONE', #31259, .T. ) ;
#26248=VECTOR ( 'NONE', #25966, 1000.000000000000000 ) ;
#26252=ORIENTED_EDGE ( 'NONE', *, *, #4286, .F. ) ;
#26253=ORIENTED_EDGE ( 'NONE', *, *, #31961, .F. ) ;
#26254=CARTESIAN_POINT ( 'NONE',  ( -19.99999999999998934, -124.9999999999999432, -154.9999999999999716 ) ) ;
#26257=DIRECTION ( 'NONE',  ( 0.000000000000000000, 1.000000000000000000, -6.123233995736766036E-17 ) ) ;
#26259=DIRECTION ( 'NONE',  ( -1.292961597001347186E-16, -0.000000000000000000, 1.000000000000000000 ) ) ;
#26262=DIRECTION ( 'NONE',  ( 0.000000000000000000, 0.000000000000000000, -1.000000000000000000 ) ) ;
#26266=CARTESIAN_POINT ( 'NONE',  ( 11.99999999999999645, -115.0000000000000000, 162.9999999999999716 ) ) ;
#26268=AXIS2_PLACEMENT_3D ( 'NONE', #29608, #2889, #5203 ) ;
#26269=VECTOR ( 'NONE', #2227, 1000.000000000000000 ) ;
#26274=EDGE_CURVE ( 'NONE', #8875, #34985, #22609, .T. ) ;
#26276=ORIENTED_EDGE ( 'NONE', *, *, #15048, .F. ) ;
#26277=EDGE_CURVE ( 'NONE', #392, #9284, #24048, .T. ) ;
#26278=EDGE_CURVE ( 'NONE', #1290, #18216, #23501, .T. ) ;
#26280=ORIENTED_EDGE ( 'NONE', *, *, #26746, .T. ) ;
#26282=ORIENTED_EDGE ( 'NONE', *, *, #26278, .F. ) ;
#26284=DIRECTION ( 'NONE',  ( 1.300283923313630633E-47, 0.000000000000000000, 1.000000000000000000 ) ) ;
#26286=CARTESIAN_POINT ( 'NONE',  ( -355.0000000000000000, 118.9999999999999858, 128.0000000000000000 ) ) ;
#26292=EDGE_CURVE ( 'NONE', #30412, #5400, #17283, .T. ) ;
#26293=DIRECTION ( 'NONE',  ( -3.040835319149746090E-31, -1.000000000000000000, 0.000000000000000000 ) ) ;
#26295=LINE ( 'NONE', #17786, #11085 ) ;
#26296=DIRECTION ( 'NONE',  ( -0.000000000000000000, -1.000000000000000000, -0.000000000000000000 ) ) ;
#26302=ORIENTED_EDGE ( 'NONE', *, *, #16795, .F. ) ;
#26303=DIRECTION ( 'NONE',  ( 1.000000000000000000, 0.000000000000000000, -1.848892746611746966E-32 ) ) ;
#26304=CARTESIAN_POINT ( 'NONE',  ( 11.99999999999999645, -145.0000000000000000, -194.9999999999999432 ) ) ;
#26310=ORIENTED_EDGE ( 'NONE', *, *, #30444, .T. ) ;
#26311=CARTESIAN_POINT ( 'NONE',  ( -442.0000000000000000, -105.0000000000000142, -174.9999999999999716 ) ) ;
#26315=VERTEX_POINT ( 'NONE', #14251 ) ;
#26317=ORIENTED_EDGE ( 'NONE', *, *, #10010, .F. ) ;
#26319=EDGE_CURVE ( 'NONE', #17362, #9284, #11576, .T. ) ;
#26322=AXIS2_PLACEMENT_3D ( 'NONE', #1496, #26568, #9676 ) ;
#26323=ORIENTED_EDGE ( 'NONE', *, *, #7584, .F. ) ;
#26326=CARTESIAN_POINT ( 'NONE',  ( -355.0000000000000000, -131.0000000000000000, 130.0000000000000000 ) ) ;
#26327=DIRECTION ( 'NONE',  ( -1.000000000000000000, 0.000000000000000000, 0.000000000000000000 ) ) ;
#26331=VECTOR ( 'NONE', #5540, 1000.000000000000000 ) ;
#26334=ORIENTED_EDGE ( 'NONE', *, *, #6303, .T. ) ;
#26335=ORIENTED_EDGE ( 'NONE', *, *, #28216, .F. ) ;
#26338=DIRECTION ( 'NONE',  ( 1.000000000000000000, 0.000000000000000000, 1.300283923313630633E-47 ) ) ;
#26339=DIRECTION ( 'NONE',  ( 0.000000000000000000, 0.000000000000000000, 1.000000000000000000 ) ) ;
#26340=ORIENTED_EDGE ( 'NONE', *, *, #4485, .F. ) ;
#26341=ADVANCED_FACE ( 'NONE', ( #11391, #22250, #6388 ), #14783, .T. ) ;
#26344=FACE_OUTER_BOUND ( 'NONE', #8230, .T. ) ;
#26345=VECTOR ( 'NONE', #27935, 1000.000000000000000 ) ;
#26347=ORIENTED_EDGE ( 'NONE', *, *, #8059, .F. ) ;
#26349=CARTESIAN_POINT ( 'NONE',  ( -349.0000000000000000, -125.0000000000000284, 181.0000000000000000 ) ) ;
#26350=EDGE_CURVE ( 'NONE', #19234, #19763, #14430, .T. ) ;
#26352=CARTESIAN_POINT ( 'NONE',  ( -441.9999999999999432, 104.9999999999999858, -190.9999999999999716 ) ) ;
#26358=LINE ( 'NONE', #34196, #16182 ) ;
#26361=VERTEX_POINT ( 'NONE', #20115 ) ;
#26363=ORIENTED_EDGE ( 'NONE', *, *, #6464, .F. ) ;
#26368=VECTOR ( 'NONE', #21335, 1000.000000000000000 ) ;
#26370=ORIENTED_EDGE ( 'NONE', *, *, #3463, .T. ) ;
#26371=EDGE_LOOP ( 'NONE', ( #21384, #21294, #9213, #15756 ) ) ;
#26373=AXIS2_PLACEMENT_3D ( 'NONE', #26326, #4779, #18862 ) ;
#26377=VERTEX_POINT ( 'NONE', #16929 ) ;
#26381=CARTESIAN_POINT ( 'NONE',  ( -410.0000000000000568, -105.0000000000000142, 162.9999999999999716 ) ) ;
#26385=EDGE_CURVE ( 'NONE', #16134, #34303, #5881, .T. ) ;
#26386=CARTESIAN_POINT ( 'NONE',  ( 19.99999999999998934, 124.9999999999999716, 187.0000000000000000 ) ) ;
#26388=ADVANCED_FACE ( 'NONE', ( #24903 ), #540, .T. ) ;
#26389=VECTOR ( 'NONE', #17959, 1000.000000000000000 ) ;
#26391=DIRECTION ( 'NONE',  ( 0.000000000000000000, 1.000000000000000000, 1.224646799147353207E-16 ) ) ;
#26399=LINE ( 'NONE', #15214, #30338 ) ;
#26409=DIRECTION ( 'NONE',  ( 0.000000000000000000, 0.000000000000000000, -1.000000000000000000 ) ) ;
#26410=ORIENTED_EDGE ( 'NONE', *, *, #3211, .F. ) ;
#26413=CIRCLE ( 'NONE', #15086, 4.000000000000003553 ) ;
#26416=PLANE ( 'NONE',  #7700 ) ;
#26417=CARTESIAN_POINT ( 'NONE',  ( -414.0000000000000568, -125.0000000000000000, 187.0000000000000000 ) ) ;
#26418=VERTEX_POINT ( 'NONE', #4410 ) ;
#26421=DIRECTION ( 'NONE',  ( 0.000000000000000000, -1.000000000000000000, -1.310824597558155437E-49 ) ) ;
#26422=DIRECTION ( 'NONE',  ( -1.000000000000000000, 0.000000000000000000, -0.000000000000000000 ) ) ;
#26424=DIRECTION ( 'NONE',  ( -3.469446951953832974E-18, -1.000000000000000000, -7.888609052210116302E-31 ) ) ;
#26425=DIRECTION ( 'NONE',  ( 0.000000000000000000, 0.000000000000000000, 1.000000000000000000 ) ) ;
#26427=ORIENTED_EDGE ( 'NONE', *, *, #26098, .T. ) ;
#26429=EDGE_CURVE ( 'NONE', #8179, #11374, #21273, .T. ) ;
#26432=ADVANCED_FACE ( 'NONE', ( #20979, #18328 ), #12811, .T. ) ;
#26433=CARTESIAN_POINT ( 'NONE',  ( -441.9999999999999432, 109.0000000000000142, 154.9999999999999716 ) ) ;
#26434=LINE ( 'NONE', #5060, #26269 ) ;
#26436=ORIENTED_EDGE ( 'NONE', *, *, #1248, .F. ) ;
#26439=CIRCLE ( 'NONE', #3137, 3.999999999999976019 ) ;
#26456=CARTESIAN_POINT ( 'NONE',  ( 11.99999999999999645, -141.0000000000000000, 155.0000000000000000 ) ) ;
#26458=PLANE ( 'NONE',  #29214 ) ;
#26459=DIRECTION ( 'NONE',  ( 0.000000000000000000, 2.309213040847544338E-50, 1.000000000000000000 ) ) ;
#26460=CARTESIAN_POINT ( 'NONE',  ( -12.00000000000001066, 112.9999999999999574, 155.0000000000000000 ) ) ;
#26470=DIRECTION ( 'NONE',  ( 0.000000000000000000, 0.000000000000000000, 1.000000000000000000 ) ) ;
#26475=EDGE_CURVE ( 'NONE', #5041, #17164, #28464, .T. ) ;
#26481=ORIENTED_EDGE ( 'NONE', *, *, #28166, .F. ) ;
#26482=AXIS2_PLACEMENT_3D ( 'NONE', #1350, #34083, #6840 ) ;
#26486=ORIENTED_EDGE ( 'NONE', *, *, #17131, .F. ) ;
#26488=ADVANCED_FACE ( 'NONE', ( #23465 ), #23303, .T. ) ;
#26492=DIRECTION ( 'NONE',  ( 3.469446951953832974E-18, 1.000000000000000000, 7.888609052210116302E-31 ) ) ;
#26493=FACE_OUTER_BOUND ( 'NONE', #12355, .T. ) ;
#26497=ORIENTED_EDGE ( 'NONE', *, *, #32697, .T. ) ;
#26502=DIRECTION ( 'NONE',  ( -3.469446951953832974E-18, -1.000000000000000000, -7.888609052210116302E-31 ) ) ;
#26511=VERTEX_POINT ( 'NONE', #17802 ) ;
#26515=VECTOR ( 'NONE', #16654, 1000.000000000000000 ) ;
#26521=EDGE_CURVE ( 'NONE', #28106, #19565, #26933, .T. ) ;
#26527=DIRECTION ( 'NONE',  ( 0.000000000000000000, 0.000000000000000000, 1.000000000000000000 ) ) ;
#26528=CARTESIAN_POINT ( 'NONE',  ( -445.9999999999999432, -105.0000000000000142, 107.9999999999999858 ) ) ;
#26529=CARTESIAN_POINT ( 'NONE',  ( -441.9999999999999432, 105.0000000000000000, -73.99999999999998579 ) ) ;
#26534=AXIS2_PLACEMENT_3D ( 'NONE', #34182, #9801, #18188 ) ;
#26535=ADVANCED_FACE ( 'NONE', ( #12287, #31301 ), #25786, .F. ) ;
#26536=AXIS2_PLACEMENT_3D ( 'NONE', #13527, #172, #11026 ) ;
#26537=ORIENTED_EDGE ( 'NONE', *, *, #22567, .T. ) ;
#26541=ORIENTED_EDGE ( 'NONE', *, *, #12162, .T. ) ;
#26542=EDGE_CURVE ( 'NONE', #11811, #20392, #1928, .T. ) ;
#26544=DIRECTION ( 'NONE',  ( 0.000000000000000000, 7.888609052210118054E-31, 1.000000000000000000 ) ) ;
#26550=ADVANCED_FACE ( 'NONE', ( #2273 ), #13664, .F. ) ;
#26551=DIRECTION ( 'NONE',  ( 0.000000000000000000, 0.000000000000000000, -1.000000000000000000 ) ) ;
#26552=LINE ( 'NONE', #11022, #33037 ) ;
#26553=VERTEX_POINT ( 'NONE', #7607 ) ;
#26556=LINE ( 'NONE', #10894, #26621 ) ;
#26561=DIRECTION ( 'NONE',  ( 0.000000000000000000, 1.131431318426415506E-52, 1.000000000000000000 ) ) ;
#26564=LINE ( 'NONE', #12709, #22492 ) ;
#26565=ADVANCED_FACE ( 'NONE', ( #10290 ), #21152, .T. ) ;
#26567=DIRECTION ( 'NONE',  ( 0.000000000000000000, 0.000000000000000000, 1.000000000000000000 ) ) ;
#26568=DIRECTION ( 'NONE',  ( 1.000000000000000000, 3.469446951953834515E-18, 0.000000000000000000 ) ) ;
#26571=FACE_OUTER_BOUND ( 'NONE', #23570, .T. ) ;
#26573=ORIENTED_EDGE ( 'NONE', *, *, #18712, .F. ) ;
#26574=DIRECTION ( 'NONE',  ( 0.000000000000000000, 0.000000000000000000, 1.000000000000000000 ) ) ;
#26579=CARTESIAN_POINT ( 'NONE',  ( 0.000000000000000000, 0.000000000000000000, 0.000000000000000000 ) ) ;
#26586=ORIENTED_EDGE ( 'NONE', *, *, #31544, .T. ) ;
#26588=VERTEX_POINT ( 'NONE', #19200 ) ;
#26589=EDGE_LOOP ( 'NONE', ( #18272, #25065, #910, #3690 ) ) ;
#26590=CARTESIAN_POINT ( 'NONE',  ( -445.9999999999999432, -104.9999999999999858, -162.9999999999999716 ) ) ;
#26593=DIRECTION ( 'NONE',  ( 0.000000000000000000, 0.000000000000000000, -1.000000000000000000 ) ) ;
#26594=EDGE_LOOP ( 'NONE', ( #1885, #9817, #2696, #30347 ) ) ;
#26596=LINE ( 'NONE', #34618, #9455 ) ;
#26600=DIRECTION ( 'NONE',  ( 0.000000000000000000, -5.053935297177146739E-49, -1.000000000000000000 ) ) ;
#26601=UNCERTAINTY_MEASURE_WITH_UNIT (LENGTH_MEASURE( 1.000000000000000082E-05 ), #14230, 'distance_accuracy_value', 'NONE');
#26603=LINE ( 'NONE', #22417, #3703 ) ;
#26608=CARTESIAN_POINT ( 'NONE',  ( 12.00000000000001066, -60.99999999999997158, -154.9999999999999716 ) ) ;
#26613=AXIS2_PLACEMENT_3D ( 'NONE', #17645, #28478, #9616 ) ;
#26614=( GEOMETRIC_REPRESENTATION_CONTEXT ( 3 ) GLOBAL_UNCERTAINTY_ASSIGNED_CONTEXT ( ( #26601 ) ) GLOBAL_UNIT_ASSIGNED_CONTEXT ( ( #14230, #12091, #33787 ) ) REPRESENTATION_CONTEXT ( 'NONE', 'WORKASPACE' ) );
#26615=DIRECTION ( 'NONE',  ( 0.000000000000000000, -1.000000000000000000, -2.465190328815662439E-32 ) ) ;
#26616=ORIENTED_EDGE ( 'NONE', *, *, #11341, .T. ) ;
#26617=EDGE_CURVE ( 'NONE', #22809, #9452, #7964, .T. ) ;
#26618=LINE ( 'NONE', #16135, #14278 ) ;
#26619=CARTESIAN_POINT ( 'NONE',  ( 19.99999999999998934, -55.00000000000000711, 162.9999999999999716 ) ) ;
#26621=VECTOR ( 'NONE', #29411, 1000.000000000000000 ) ;
#26624=CARTESIAN_POINT ( 'NONE',  ( -12.00000000000001066, 108.9999999999999858, 155.0000000000000000 ) ) ;
#26625=ADVANCED_FACE ( 'NONE', ( #16000 ), #18842, .T. ) ;
#26628=ADVANCED_FACE ( 'NONE', ( #2448 ), #13330, .T. ) ;
#26635=ORIENTED_EDGE ( 'NONE', *, *, #23149, .T. ) ;
#26637=DIRECTION ( 'NONE',  ( 0.000000000000000000, 2.309213040847544338E-50, 1.000000000000000000 ) ) ;
#26640=LINE ( 'NONE', #15102, #19367 ) ;
#26648=CARTESIAN_POINT ( 'NONE',  ( 11.99999999999995559, -145.0000000000000000, -194.9999999999999432 ) ) ;
#26650=PLANE ( 'NONE',  #15667 ) ;
#26651=FACE_OUTER_BOUND ( 'NONE', #13118, .T. ) ;
#26653=LINE ( 'NONE', #9755, #12822 ) ;
#26654=ORIENTED_EDGE ( 'NONE', *, *, #15255, .F. ) ;
#26655=DIRECTION ( 'NONE',  ( -3.040835319149746090E-31, -1.000000000000000000, 0.000000000000000000 ) ) ;
#26657=CARTESIAN_POINT ( 'NONE',  ( -20.00000000000004619, -134.9999999999999716, -162.9999999999999432 ) ) ;
#26664=VECTOR ( 'NONE', #5693, 1000.000000000000000 ) ;
#26668=CARTESIAN_POINT ( 'NONE',  ( -414.0000000000000568, -125.0000000000000000, 162.9999999999999716 ) ) ;
#26669=LINE ( 'NONE', #15482, #27385 ) ;
#26681=DIRECTION ( 'NONE',  ( 1.000000000000000000, 0.000000000000000000, 0.000000000000000000 ) ) ;
#26685=CYLINDRICAL_SURFACE ( 'NONE', #21519, 3.999999999999976019 ) ;
#26694=DIRECTION ( 'NONE',  ( 0.000000000000000000, 1.000000000000000000, 1.131431318426415506E-52 ) ) ;
#26697=AXIS2_PLACEMENT_3D ( 'NONE', #25224, #30928, #12080 ) ;
#26698=CARTESIAN_POINT ( 'NONE',  ( -20.00000000000007461, 140.9999999999999432, -162.9999999999999716 ) ) ;
#26702=CARTESIAN_POINT ( 'NONE',  ( -442.0000000000000000, -125.0000000000000000, 107.9999999999999858 ) ) ;
#26705=DIRECTION ( 'NONE',  ( -1.300283923313630633E-47, 0.000000000000000000, -1.000000000000000000 ) ) ;
#26706=LINE ( 'NONE', #21381, #25637 ) ;
#26708=DIRECTION ( 'NONE',  ( -1.292961597001347186E-16, -0.000000000000000000, 1.000000000000000000 ) ) ;
#26710=CARTESIAN_POINT ( 'NONE',  ( -499.9999999999998863, -109.0000000000000142, -187.0000000000000000 ) ) ;
#26714=VERTEX_POINT ( 'NONE', #17377 ) ;
#26718=CARTESIAN_POINT ( 'NONE',  ( -430.0000000000000000, 130.9999999999999716, 109.9999999999999858 ) ) ;
#26719=EDGE_CURVE ( 'NONE', #31417, #18709, #24661, .T. ) ;
#26721=ORIENTED_EDGE ( 'NONE', *, *, #12707, .T. ) ;
#26723=CARTESIAN_POINT ( 'NONE',  ( -12.00000000000001066, -32.99999999999997158, -154.9999999999999716 ) ) ;
#26724=DIRECTION ( 'NONE',  ( 0.000000000000000000, 1.000000000000000000, 1.224646799147353207E-16 ) ) ;
#26725=ORIENTED_EDGE ( 'NONE', *, *, #26277, .T. ) ;
#26734=ORIENTED_EDGE ( 'NONE', *, *, #17735, .T. ) ;
#26735=FACE_OUTER_BOUND ( 'NONE', #13493, .T. ) ;
#26736=CARTESIAN_POINT ( 'NONE',  ( -499.9999999999999432, -141.0000000000000000, -187.0000000000000000 ) ) ;
#26737=CARTESIAN_POINT ( 'NONE',  ( 19.99999999999998224, 134.9999999999999432, -162.9999999999999432 ) ) ;
#26743=CARTESIAN_POINT ( 'NONE',  ( -345.0000000000000000, -125.0000000000000284, 181.0000000000000000 ) ) ;
#26746=EDGE_CURVE ( 'NONE', #29991, #4421, #18444, .T. ) ;
#26749=ORIENTED_EDGE ( 'NONE', *, *, #22506, .F. ) ;
#26753=ADVANCED_FACE ( 'NONE', ( #9341 ), #17197, .T. ) ;
#26754=VERTEX_POINT ( 'NONE', #25525 ) ;
#26755=VECTOR ( 'NONE', #31208, 1000.000000000000000 ) ;
#26759=EDGE_CURVE ( 'NONE', #9246, #15148, #17024, .T. ) ;
#26761=ORIENTED_EDGE ( 'NONE', *, *, #18464, .F. ) ;
#26763=ORIENTED_EDGE ( 'NONE', *, *, #26319, .F. ) ;
#26766=FACE_OUTER_BOUND ( 'NONE', #15811, .T. ) ;
#26770=ORIENTED_EDGE ( 'NONE', *, *, #5338, .T. ) ;
#26771=VERTEX_POINT ( 'NONE', #25167 ) ;
#26772=CARTESIAN_POINT ( 'NONE',  ( 19.99999999999998934, 136.9999999999999716, -155.0000000000000000 ) ) ;
#26773=CARTESIAN_POINT ( 'NONE',  ( -355.0000000000000000, -119.0000000000000000, 126.0000000000000000 ) ) ;
#26775=EDGE_LOOP ( 'NONE', ( #11530, #9127, #8534, #21626 ) ) ;
#26777=VECTOR ( 'NONE', #21541, 1000.000000000000000 ) ;
#26780=VECTOR ( 'NONE', #13026, 1000.000000000000000 ) ;
#26783=FACE_OUTER_BOUND ( 'NONE', #19450, .T. ) ;
#26787=EDGE_CURVE ( 'NONE', #13518, #30135, #11671, .T. ) ;
#26788=DIRECTION ( 'NONE',  ( 1.000000000000000000, 0.000000000000000000, 0.000000000000000000 ) ) ;
#26790=ADVANCED_FACE ( 'NONE', ( #34420 ), #24070, .F. ) ;
#26792=ORIENTED_EDGE ( 'NONE', *, *, #2719, .F. ) ;
#26796=CARTESIAN_POINT ( 'NONE',  ( -418.0000000000000000, 104.9999999999999858, -194.9999999999999716 ) ) ;
#26797=EDGE_CURVE ( 'NONE', #14082, #10047, #15386, .T. ) ;
#26798=AXIS2_PLACEMENT_3D ( 'NONE', #28873, #14845, #34215 ) ;
#26803=EDGE_LOOP ( 'NONE', ( #26749, #28284, #25114, #17302, #31339, #26282, #16328, #30969 ) ) ;
#26804=VECTOR ( 'NONE', #10817, 1000.000000000000000 ) ;
#26808=EDGE_LOOP ( 'NONE', ( #5260, #20691, #4643, #18304 ) ) ;
#26810=VERTEX_POINT ( 'NONE', #34773 ) ;
#26811=AXIS2_PLACEMENT_3D ( 'NONE', #14024, #3152, #9203 ) ;
#26816=VERTEX_POINT ( 'NONE', #4326 ) ;
#26819=EDGE_CURVE ( 'NONE', #1154, #32678, #23736, .T. ) ;
#26822=LINE ( 'NONE', #2429, #3433 ) ;
#26824=CYLINDRICAL_SURFACE ( 'NONE', #13762, 4.750000000000004441 ) ;
#26827=ORIENTED_EDGE ( 'NONE', *, *, #6734, .T. ) ;
#26830=LINE ( 'NONE', #4930, #25690 ) ;
#26831=ADVANCED_FACE ( 'NONE', ( #31904 ), #2193, .F. ) ;
#26832=VECTOR ( 'NONE', #22385, 1000.000000000000000 ) ;
#26833=DIRECTION ( 'NONE',  ( 0.000000000000000000, 1.000000000000000000, 2.309213040847544338E-50 ) ) ;
#26838=ORIENTED_EDGE ( 'NONE', *, *, #12854, .F. ) ;
#26840=DIRECTION ( 'NONE',  ( 0.000000000000000000, 0.000000000000000000, -1.000000000000000000 ) ) ;
#26842=CARTESIAN_POINT ( 'NONE',  ( -430.0000000000000000, -114.9999999999999858, 113.9999999999999858 ) ) ;
#26843=CARTESIAN_POINT ( 'NONE',  ( -442.0000000000000000, 105.0000000000000000, -77.99999999999997158 ) ) ;
#26844=CARTESIAN_POINT ( 'NONE',  ( -449.9999999999999432, 124.9999999999999574, -187.0000000000000000 ) ) ;
#26845=ORIENTED_EDGE ( 'NONE', *, *, #32618, .T. ) ;
#26850=CARTESIAN_POINT ( 'NONE',  ( -418.0000000000000000, 104.9999999999999858, -155.0000000000000000 ) ) ;
#26851=LINE ( 'NONE', #13165, #33422 ) ;
#26853=DIRECTION ( 'NONE',  ( 1.000000000000000000, 0.000000000000000000, 0.000000000000000000 ) ) ;
#26862=VERTEX_POINT ( 'NONE', #5547 ) ;
#26865=EDGE_CURVE ( 'NONE', #33296, #13606, #8056, .T. ) ;
#26866=ORIENTED_EDGE ( 'NONE', *, *, #30914, .T. ) ;
#26868=CARTESIAN_POINT ( 'NONE',  ( -499.9999999999999432, -113.0000000000000000, -187.0000000000000000 ) ) ;
#26871=CARTESIAN_POINT ( 'NONE',  ( -361.0000000000000000, -125.0000000000000284, 110.0000000000000000 ) ) ;
#26874=ORIENTED_EDGE ( 'NONE', *, *, #18810, .T. ) ;
#26875=ADVANCED_FACE ( 'NONE', ( #32265 ), #19463, .T. ) ;
#26876=CARTESIAN_POINT ( 'NONE',  ( -349.0000000000000000, -135.0000000000000000, 113.9999999999999858 ) ) ;
#26878=DIRECTION ( 'NONE',  ( -0.000000000000000000, 1.000000000000000000, -0.000000000000000000 ) ) ;
#26880=CIRCLE ( 'NONE', #9829, 3.999999999999948042 ) ;
#26881=VECTOR ( 'NONE', #26708, 1000.000000000000000 ) ;
#26883=DIRECTION ( 'NONE',  ( -0.000000000000000000, 1.000000000000000000, -0.000000000000000000 ) ) ;
#26884=DIRECTION ( 'NONE',  ( 0.000000000000000000, 5.053935297177146739E-49, 1.000000000000000000 ) ) ;
#26891=ORIENTED_EDGE ( 'NONE', *, *, #7167, .T. ) ;
#26893=DIRECTION ( 'NONE',  ( 0.000000000000000000, -0.000000000000000000, 1.000000000000000000 ) ) ;
#26895=ORIENTED_EDGE ( 'NONE', *, *, #26617, .T. ) ;
#26896=CARTESIAN_POINT ( 'NONE',  ( 11.99999999999999645, 124.9999999999999716, 155.0000000000000000 ) ) ;
#26901=ORIENTED_EDGE ( 'NONE', *, *, #13240, .F. ) ;
#26906=EDGE_CURVE ( 'NONE', #3592, #1944, #30123, .T. ) ;
#26910=ORIENTED_EDGE ( 'NONE', *, *, #24288, .T. ) ;
#26911=DIRECTION ( 'NONE',  ( 1.000000000000000000, 0.000000000000000000, 0.000000000000000000 ) ) ;
#26913=DIRECTION ( 'NONE',  ( 0.000000000000000000, 0.000000000000000000, -1.000000000000000000 ) ) ;
#26914=EDGE_CURVE ( 'NONE', #16221, #31232, #21942, .T. ) ;
#26917=EDGE_CURVE ( 'NONE', #34661, #16142, #24249, .T. ) ;
#26918=CARTESIAN_POINT ( 'NONE',  ( -11.99999999999998224, -145.0000000000000000, 155.0000000000000000 ) ) ;
#26922=ADVANCED_FACE ( 'NONE', ( #5902 ), #32790, .T. ) ;
#26926=CARTESIAN_POINT ( 'NONE',  ( -11.99999999999998224, -134.9999999999999716, 187.0000000000000000 ) ) ;
#26928=CARTESIAN_POINT ( 'NONE',  ( -499.9999999999999432, 144.9999999999999716, -162.9999999999999716 ) ) ;
#26931=VECTOR ( 'NONE', #21420, 1000.000000000000000 ) ;
#26932=VERTEX_POINT ( 'NONE', #13589 ) ;
#26933=CIRCLE ( 'NONE', #16155, 3.999999999999976019 ) ;
#26934=CYLINDRICAL_SURFACE ( 'NONE', #1849, 7.999999999999979572 ) ;
#26940=FACE_OUTER_BOUND ( 'NONE', #265, .T. ) ;
#26943=LINE ( 'NONE', #26590, #9382 ) ;
#26944=CIRCLE ( 'NONE', #29241, 7.999999999999979572 ) ;
#26947=EDGE_LOOP ( 'NONE', ( #33132, #19233, #11749, #28332 ) ) ;
#26951=AXIS2_PLACEMENT_3D ( 'NONE', #27040, #29541, #35066 ) ;
#26953=DIRECTION ( 'NONE',  ( -0.000000000000000000, -2.465190328815661892E-32, -1.000000000000000000 ) ) ;
#26955=ORIENTED_EDGE ( 'NONE', *, *, #31303, .F. ) ;
#26956=CARTESIAN_POINT ( 'NONE',  ( -345.0000000000000000, -125.0000000000000284, 181.0000000000000000 ) ) ;
#26957=CIRCLE ( 'NONE', #4206, 7.999999999999979572 ) ;
#26958=VECTOR ( 'NONE', #28853, 1000.000000000000000 ) ;
#26961=AXIS2_PLACEMENT_3D ( 'NONE', #23836, #34693, #10306 ) ;
#26963=CARTESIAN_POINT ( 'NONE',  ( -418.0000000000000000, 124.9999999999999574, -187.0000000000000000 ) ) ;
#26967=ORIENTED_EDGE ( 'NONE', *, *, #2125, .F. ) ;
#26968=EDGE_CURVE ( 'NONE', #23318, #18383, #3065, .T. ) ;
#26969=ADVANCED_FACE ( 'NONE', ( #27276 ), #2884, .F. ) ;
#26970=DIRECTION ( 'NONE',  ( 1.000000000000000000, -0.000000000000000000, -0.000000000000000000 ) ) ;
#26973=( NAMED_UNIT ( * ) SI_UNIT ( $, .STERADIAN. ) SOLID_ANGLE_UNIT ( ) );
#26979=AXIS2_PLACEMENT_3D ( 'NONE', #32019, #7635, #29896 ) ;
#26982=AXIS2_PLACEMENT_3D ( 'NONE', #11829, #9657, #6267 ) ;
#26984=CIRCLE ( 'NONE', #13938, 2.000000000000001776 ) ;
#26985=VERTEX_POINT ( 'NONE', #16090 ) ;
#26988=ORIENTED_EDGE ( 'NONE', *, *, #17544, .F. ) ;
#26989=DIRECTION ( 'NONE',  ( 0.000000000000000000, 0.000000000000000000, -1.000000000000000000 ) ) ;
#26992=ADVANCED_FACE ( 'NONE', ( #1287 ), #3936, .T. ) ;
#26995=CYLINDRICAL_SURFACE ( 'NONE', #16529, 2.000000000000001776 ) ;
#26996=VERTEX_POINT ( 'NONE', #11627 ) ;
#26998=EDGE_LOOP ( 'NONE', ( #16648, #32288, #31617, #18274 ) ) ;
#27000=CARTESIAN_POINT ( 'NONE',  ( -19.99999999999998934, 144.9999999999999716, -186.9999999999999716 ) ) ;
#27004=DIRECTION ( 'NONE',  ( 0.000000000000000000, 2.309213040847544338E-50, 1.000000000000000000 ) ) ;
#27006=DIRECTION ( 'NONE',  ( -1.000000000000000000, 0.000000000000000000, 0.000000000000000000 ) ) ;
#27007=FACE_OUTER_BOUND ( 'NONE', #1933, .T. ) ;
#27008=VERTEX_POINT ( 'NONE', #14824 ) ;
#27012=VERTEX_POINT ( 'NONE', #22823 ) ;
#27014=LINE ( 'NONE', #13326, #27446 ) ;
#27015=ORIENTED_EDGE ( 'NONE', *, *, #4135, .T. ) ;
#27017=CLOSED_SHELL ( 'NONE', ( #31600, #5277, #29977, #33700, #1322, #22710, #34194, #10041, #8318, #22787, #22604, #24292, #3734, #18672, #7384, #21946, #2280, #4771 ) ) ;
#27019=VERTEX_POINT ( 'NONE', #3588 ) ;
#27020=DIRECTION ( 'NONE',  ( 0.000000000000000000, 0.000000000000000000, -1.000000000000000000 ) ) ;
#27022=LINE ( 'NONE', #28989, #22291 ) ;
#27029=VECTOR ( 'NONE', #33885, 1000.000000000000000 ) ;
#27030=DIRECTION ( 'NONE',  ( -0.000000000000000000, 1.000000000000000000, -0.000000000000000000 ) ) ;
#27031=EDGE_CURVE ( 'NONE', #6498, #13611, #33144, .T. ) ;
#27032=DIRECTION ( 'NONE',  ( 0.000000000000000000, 0.000000000000000000, -1.000000000000000000 ) ) ;
#27038=CARTESIAN_POINT ( 'NONE',  ( -418.0000000000000000, 113.0000000000000000, -175.0000000000000000 ) ) ;
#27039=AXIS2_PLACEMENT_3D ( 'NONE', #17671, #17844, #15167 ) ;
#27040=CARTESIAN_POINT ( 'NONE',  ( 11.99999999999995559, -134.9999999999999716, -186.9999999999999716 ) ) ;
#27044=DIRECTION ( 'NONE',  ( 0.000000000000000000, 1.000000000000000000, -3.374343856708137958E-53 ) ) ;
#27047=CARTESIAN_POINT ( 'NONE',  ( -445.9999999999999432, 105.0000000000000142, 162.9999999999999716 ) ) ;
#27051=DIRECTION ( 'NONE',  ( 0.000000000000000000, 0.000000000000000000, 1.000000000000000000 ) ) ;
#27052=CYLINDRICAL_SURFACE ( 'NONE', #22314, 7.999999999999979572 ) ;
#27054=VECTOR ( 'NONE', #37, 1000.000000000000000 ) ;
#27058=PLANE ( 'NONE',  #32750 ) ;
#27060=DIRECTION ( 'NONE',  ( -1.000000000000000000, 0.000000000000000000, 0.000000000000000000 ) ) ;
#27063=ORIENTED_EDGE ( 'NONE', *, *, #29689, .T. ) ;
#27071=EDGE_CURVE ( 'NONE', #2032, #34687, #14299, .T. ) ;
#27073=ORIENTED_EDGE ( 'NONE', *, *, #23046, .F. ) ;
#27074=EDGE_CURVE ( 'NONE', #5234, #5838, #1410, .T. ) ;
#27076=CIRCLE ( 'NONE', #2000, 7.999999999999979572 ) ;
#27079=DIRECTION ( 'NONE',  ( 0.000000000000000000, 0.000000000000000000, -1.000000000000000000 ) ) ;
#27081=ORIENTED_EDGE ( 'NONE', *, *, #28887, .T. ) ;
#27082=LINE ( 'NONE', #32245, #10598 ) ;
#27084=AXIS2_PLACEMENT_3D ( 'NONE', #13069, #18239, #5030 ) ;
#27085=DIRECTION ( 'NONE',  ( 1.232595164407830946E-32, 3.421138828918010427E-49, -1.000000000000000000 ) ) ;
#27088=ORIENTED_EDGE ( 'NONE', *, *, #32175, .F. ) ;
#27089=PLANE ( 'NONE',  #10703 ) ;
#27097=CARTESIAN_POINT ( 'NONE',  ( -365.0000000000000000, -131.0000000000000000, 128.0000000000000000 ) ) ;
#27098=AXIS2_PLACEMENT_3D ( 'NONE', #23492, #7820, #13176 ) ;
#27101=CARTESIAN_POINT ( 'NONE',  ( -12.00000000000001066, 136.9999999999999716, -175.0000000000000284 ) ) ;
#27102=CARTESIAN_POINT ( 'NONE',  ( -414.0000000000000568, -137.0000000000000000, 154.9999999999999716 ) ) ;
#27104=EDGE_LOOP ( 'NONE', ( #27635, #22822, #26635, #32507 ) ) ;
#27105=DIRECTION ( 'NONE',  ( 0.000000000000000000, -0.000000000000000000, -1.000000000000000000 ) ) ;
#27106=VECTOR ( 'NONE', #10264, 1000.000000000000000 ) ;
#27110=FACE_OUTER_BOUND ( 'NONE', #33377, .T. ) ;
#27112=VERTEX_POINT ( 'NONE', #6787 ) ;
#27115=AXIS2_PLACEMENT_3D ( 'NONE', #13275, #31773, #10417 ) ;
#27119=FACE_BOUND ( 'NONE', #34957, .T. ) ;
#27122=VERTEX_POINT ( 'NONE', #759 ) ;
#27124=CARTESIAN_POINT ( 'NONE',  ( -442.0000000000000000, -105.0000000000000142, 100.0000000000000000 ) ) ;
#27125=EDGE_CURVE ( 'NONE', #32109, #6108, #12775, .T. ) ;
#27132=VERTEX_POINT ( 'NONE', #30662 ) ;
#27133=LINE ( 'NONE', #10777, #309 ) ;
#27135=CARTESIAN_POINT ( 'NONE',  ( 11.99999999999999645, -124.9999999999999432, -154.9999999999999716 ) ) ;
#27138=AXIS2_PLACEMENT_3D ( 'NONE', #12561, #21084, #26422 ) ;
#27139=CARTESIAN_POINT ( 'NONE',  ( -414.0000000000000568, 105.0000000000000000, -77.99999999999997158 ) ) ;
#27144=AXIS2_PLACEMENT_3D ( 'NONE', #24844, #22012, #24477 ) ;
#27150=AXIS2_PLACEMENT_3D ( 'NONE', #33921, #17924, #6682 ) ;
#27154=ORIENTED_EDGE ( 'NONE', *, *, #25045, .T. ) ;
#27156=CARTESIAN_POINT ( 'NONE',  ( -365.0000000000000000, -125.0000000000000284, 168.9999999999999716 ) ) ;
#27157=EDGE_CURVE ( 'NONE', #10776, #22434, #12851, .T. ) ;
#27159=CIRCLE ( 'NONE', #20920, 7.999999999999979572 ) ;
#27160=DIRECTION ( 'NONE',  ( -3.040835319149746090E-31, -1.000000000000000000, 0.000000000000000000 ) ) ;
#27165=ORIENTED_EDGE ( 'NONE', *, *, #18226, .T. ) ;
#27166=DIRECTION ( 'NONE',  ( -1.000000000000000000, 0.000000000000000000, 1.232595164407831220E-32 ) ) ;
#27167=DIRECTION ( 'NONE',  ( 1.000000000000000000, 0.000000000000000000, 0.000000000000000000 ) ) ;
#27171=AXIS2_PLACEMENT_3D ( 'NONE', #19214, #24349, #29533 ) ;
#27174=CARTESIAN_POINT ( 'NONE',  ( -418.0000000000000000, -141.0000000000000000, -175.0000000000000000 ) ) ;
#27175=DIRECTION ( 'NONE',  ( 0.000000000000000000, 2.309213040847544338E-50, 1.000000000000000000 ) ) ;
#27176=ORIENTED_EDGE ( 'NONE', *, *, #33503, .T. ) ;
#27177=CARTESIAN_POINT ( 'NONE',  ( -499.9999999999999432, 112.9999999999999574, -190.9999999999999716 ) ) ;
#27178=CARTESIAN_POINT ( 'NONE',  ( -20.00000000000004619, -134.9999999999999716, -186.9999999999999716 ) ) ;
#27183=CARTESIAN_POINT ( 'NONE',  ( -12.00000000000001066, -32.99999999999997158, 154.9999999999999716 ) ) ;
#27185=LINE ( 'NONE', #21151, #31928 ) ;
#27187=CIRCLE ( 'NONE', #25486, 3.999999999999976019 ) ;
#27190=CIRCLE ( 'NONE', #28347, 4.000000000000003553 ) ;
#27192=FACE_OUTER_BOUND ( 'NONE', #32586, .T. ) ;
#27194=CARTESIAN_POINT ( 'NONE',  ( -445.9999999999999432, -125.0000000000000000, 187.0000000000000000 ) ) ;
#27196=ORIENTED_EDGE ( 'NONE', *, *, #28997, .T. ) ;
#27197=AXIS2_PLACEMENT_3D ( 'NONE', #9918, #25761, #9404 ) ;
#27202=CARTESIAN_POINT ( 'NONE',  ( -499.9999999999999432, 136.9999999999999432, 187.0000000000000000 ) ) ;
#27204=CYLINDRICAL_SURFACE ( 'NONE', #34032, 3.999999999999982681 ) ;
#27207=EDGE_CURVE ( 'NONE', #18201, #4999, #21298, .T. ) ;
#27208=ORIENTED_EDGE ( 'NONE', *, *, #14829, .F. ) ;
#27209=EDGE_CURVE ( 'NONE', #707, #16352, #26358, .T. ) ;
#27210=ORIENTED_EDGE ( 'NONE', *, *, #10587, .F. ) ;
#27211=VERTEX_POINT ( 'NONE', #20676 ) ;
#27212=DIRECTION ( 'NONE',  ( 0.000000000000000000, 0.000000000000000000, -1.000000000000000000 ) ) ;
#27213=LINE ( 'NONE', #11375, #96 ) ;
#27218=CARTESIAN_POINT ( 'NONE',  ( -442.0000000000000000, -105.0000000000000142, 187.0000000000000000 ) ) ;
#27221=CARTESIAN_POINT ( 'NONE',  ( -355.0000000000000000, -131.0000000000000000, 113.9999999999999858 ) ) ;
#27222=VERTEX_POINT ( 'NONE', #18371 ) ;
#27224=VERTEX_POINT ( 'NONE', #9814 ) ;
#27227=EDGE_LOOP ( 'NONE', ( #18296, #30599 ) ) ;
#27228=DIRECTION ( 'NONE',  ( 1.000000000000000000, 0.000000000000000000, 0.000000000000000000 ) ) ;
#27234=EDGE_CURVE ( 'NONE', #16703, #18132, #20844, .T. ) ;
#27235=CARTESIAN_POINT ( 'NONE',  ( -20.00000000000001776, -113.0000000000000000, 194.9999999999999716 ) ) ;
#27236=CARTESIAN_POINT ( 'NONE',  ( -449.9999999999999432, -105.0000000000000142, -174.9999999999999432 ) ) ;
#27237=DIRECTION ( 'NONE',  ( 0.000000000000000000, 0.000000000000000000, 1.000000000000000000 ) ) ;
#27239=EDGE_LOOP ( 'NONE', ( #31997, #31069, #34110, #5596 ) ) ;
#27243=ORIENTED_EDGE ( 'NONE', *, *, #26098, .F. ) ;
#27244=AXIS2_PLACEMENT_3D ( 'NONE', #8028, #22094, #16773 ) ;
#27245=CARTESIAN_POINT ( 'NONE',  ( -418.0000000000000000, -105.0000000000000142, 107.9999999999999858 ) ) ;
#27246=ORIENTED_EDGE ( 'NONE', *, *, #20276, .F. ) ;
#27252=LINE ( 'NONE', #2859, #17331 ) ;
#27253=CARTESIAN_POINT ( 'NONE',  ( -365.0000000000000000, 130.9999999999999716, 109.9999999999999858 ) ) ;
#27254=ORIENTED_EDGE ( 'NONE', *, *, #17299, .F. ) ;
#27255=ORIENTED_EDGE ( 'NONE', *, *, #11174, .T. ) ;
#27257=CARTESIAN_POINT ( 'NONE',  ( -418.0000000000000000, 104.9999999999999858, 155.0000000000000000 ) ) ;
#27260=DIRECTION ( 'NONE',  ( 1.000000000000000000, 3.469446951953834515E-18, 0.000000000000000000 ) ) ;
#27265=CARTESIAN_POINT ( 'NONE',  ( -70.00000000000000000, 75.55999999999990280, -172.9900000000000091 ) ) ;
#27270=EDGE_CURVE ( 'NONE', #11365, #18155, #21197, .T. ) ;
#27271=PLANE ( 'NONE',  #20718 ) ;
#27274=PLANE ( 'NONE',  #8763 ) ;
#27276=FACE_OUTER_BOUND ( 'NONE', #15616, .T. ) ;
#27281=ORIENTED_EDGE ( 'NONE', *, *, #15886, .F. ) ;
#27282=VERTEX_POINT ( 'NONE', #22079 ) ;
#27283=DIRECTION ( 'NONE',  ( 0.000000000000000000, 5.053935297177146739E-49, 1.000000000000000000 ) ) ;
#27286=CARTESIAN_POINT ( 'NONE',  ( -349.0000000000000000, -125.0000000000000284, 181.0000000000000000 ) ) ;
#27288=DIRECTION ( 'NONE',  ( -1.000000000000000000, 0.000000000000000000, 0.000000000000000000 ) ) ;
#27289=ORIENTED_EDGE ( 'NONE', *, *, #11004, .F. ) ;
#27293=DIRECTION ( 'NONE',  ( 0.000000000000000000, 1.000000000000000000, -3.374343856708137958E-53 ) ) ;
#27294=DIRECTION ( 'NONE',  ( 0.000000000000000000, 1.000000000000000000, 1.224646799147353207E-16 ) ) ;
#27295=ORIENTED_EDGE ( 'NONE', *, *, #34705, .T. ) ;
#27296=AXIS2_PLACEMENT_3D ( 'NONE', #33252, #9408, #1212 ) ;
#27300=EDGE_CURVE ( 'NONE', #25547, #27889, #8541, .T. ) ;
#27306=ORIENTED_EDGE ( 'NONE', *, *, #1342, .T. ) ;
#27310=ORIENTED_EDGE ( 'NONE', *, *, #33489, .F. ) ;
#27316=DIRECTION ( 'NONE',  ( -0.000000000000000000, 1.000000000000000000, -0.000000000000000000 ) ) ;
#27322=VERTEX_POINT ( 'NONE', #24733 ) ;
#27323=ORIENTED_EDGE ( 'NONE', *, *, #2367, .T. ) ;
#27326=ORIENTED_EDGE ( 'NONE', *, *, #20341, .F. ) ;
#27328=DIRECTION ( 'NONE',  ( -1.000000000000000000, -3.469446951953834515E-18, 0.000000000000000000 ) ) ;
#27329=DIRECTION ( 'NONE',  ( -1.000000000000000000, 0.000000000000000000, -1.300283923313630633E-47 ) ) ;
#27331=VECTOR ( 'NONE', #29759, 1000.000000000000000 ) ;
#27332=FACE_OUTER_BOUND ( 'NONE', #23206, .T. ) ;
#27334=ORIENTED_EDGE ( 'NONE', *, *, #5797, .F. ) ;
#27335=AXIS2_PLACEMENT_3D ( 'NONE', #4413, #2111, #6911 ) ;
#27336=CARTESIAN_POINT ( 'NONE',  ( -20.00000000000007461, 140.9999999999999716, -162.9999999999999716 ) ) ;
#27338=AXIS2_PLACEMENT_3D ( 'NONE', #28206, #11313, #6295 ) ;
#27344=VERTEX_POINT ( 'NONE', #29916 ) ;
#27345=VECTOR ( 'NONE', #3270, 1000.000000000000000 ) ;
#27347=CYLINDRICAL_SURFACE ( 'NONE', #4627, 7.999999999999979572 ) ;
#27348=VECTOR ( 'NONE', #22843, 1000.000000000000000 ) ;
#27351=APPLICATION_CONTEXT ( 'automotive_design' ) ;
#27352=DIRECTION ( 'NONE',  ( 0.000000000000000000, 1.000000000000000000, -5.145227585319922065E-49 ) ) ;
#27353=ORIENTED_EDGE ( 'NONE', *, *, #25399, .F. ) ;
#27357=ADVANCED_FACE ( 'NONE', ( #13894 ), #13714, .F. ) ;
#27359=VERTEX_POINT ( 'NONE', #21896 ) ;
#27363=LINE ( 'NONE', #13848, #21702 ) ;
#27368=ORIENTED_EDGE ( 'NONE', *, *, #31697, .T. ) ;
#27372=DIRECTION ( 'NONE',  ( -0.000000000000000000, -1.310824597558155437E-49, -1.000000000000000000 ) ) ;
#27373=EDGE_CURVE ( 'NONE', #20130, #16547, #10, .T. ) ;
#27375=FACE_OUTER_BOUND ( 'NONE', #3086, .T. ) ;
#27380=ORIENTED_EDGE ( 'NONE', *, *, #27386, .F. ) ;
#27381=ORIENTED_EDGE ( 'NONE', *, *, #12105, .F. ) ;
#27384=DIRECTION ( 'NONE',  ( 0.000000000000000000, 0.000000000000000000, -1.000000000000000000 ) ) ;
#27385=VECTOR ( 'NONE', #7609, 1000.000000000000000 ) ;
#27386=EDGE_CURVE ( 'NONE', #2370, #8469, #17365, .T. ) ;
#27388=ADVANCED_FACE ( 'NONE', ( #5860 ), #29735, .F. ) ;
#27395=VECTOR ( 'NONE', #32179, 1000.000000000000000 ) ;
#27397=FACE_OUTER_BOUND ( 'NONE', #22722, .T. ) ;
#27398=VERTEX_POINT ( 'NONE', #5336 ) ;
#27400=DIRECTION ( 'NONE',  ( 0.000000000000000000, 0.000000000000000000, 1.000000000000000000 ) ) ;
#27405=DIRECTION ( 'NONE',  ( 0.000000000000000000, 1.000000000000000000, 5.145227585319922065E-49 ) ) ;
#27406=DIRECTION ( 'NONE',  ( 0.000000000000000000, 1.000000000000000000, 5.053935297177146739E-49 ) ) ;
#27408=EDGE_CURVE ( 'NONE', #25387, #29898, #30420, .T. ) ;
#27410=DIRECTION ( 'NONE',  ( -1.000000000000000000, -3.040835319149746528E-31, -1.232595164407830946E-32 ) ) ;
#27412=DIRECTION ( 'NONE',  ( 0.000000000000000000, 1.310824597558155437E-49, 1.000000000000000000 ) ) ;
#27413=EDGE_CURVE ( 'NONE', #19034, #8292, #21382, .T. ) ;
#27414=ORIENTED_EDGE ( 'NONE', *, *, #24211, .F. ) ;
#27415=CIRCLE ( 'NONE', #12095, 7.999999999999979572 ) ;
#27416=VECTOR ( 'NONE', #3108, 1000.000000000000000 ) ;
#27421=ORIENTED_EDGE ( 'NONE', *, *, #34960, .F. ) ;
#27424=DIRECTION ( 'NONE',  ( 0.000000000000000000, 0.000000000000000000, -1.000000000000000000 ) ) ;
#27425=CARTESIAN_POINT ( 'NONE',  ( 19.99999999999998934, 75.55999999999990280, -172.9900000000000091 ) ) ;
#27427=ADVANCED_FACE ( 'NONE', ( #14436 ), #14073, .F. ) ;
#27429=EDGE_CURVE ( 'NONE', #24623, #4681, #23583, .T. ) ;
#27430=DIRECTION ( 'NONE',  ( 0.000000000000000000, -1.000000000000000000, -2.465190328815662439E-32 ) ) ;
#27433=ORIENTED_EDGE ( 'NONE', *, *, #2681, .T. ) ;
#27436=EDGE_CURVE ( 'NONE', #29137, #11246, #22432, .T. ) ;
#27438=DIRECTION ( 'NONE',  ( 0.000000000000000000, 0.000000000000000000, -1.000000000000000000 ) ) ;
#27439=PLANE ( 'NONE',  #16014 ) ;
#27440=PRODUCT_DEFINITION_CONTEXT ( 'detailed design', #1679, 'design' ) ;
#27441=ORIENTED_EDGE ( 'NONE', *, *, #18464, .T. ) ;
#27444=DIRECTION ( 'NONE',  ( 0.000000000000000000, 1.131431318426415506E-52, 1.000000000000000000 ) ) ;
#27446=VECTOR ( 'NONE', #23645, 1000.000000000000000 ) ;
#27451=LINE ( 'NONE', #26743, #10984 ) ;
#27453=DIRECTION ( 'NONE',  ( -1.000000000000000000, 0.000000000000000000, 0.000000000000000000 ) ) ;
#27455=LINE ( 'NONE', #11094, #17309 ) ;
#27462=ORIENTED_EDGE ( 'NONE', *, *, #1689, .T. ) ;
#27465=ORIENTED_EDGE ( 'NONE', *, *, #4798, .T. ) ;
#27466=DIRECTION ( 'NONE',  ( 0.000000000000000000, 1.000000000000000000, 5.145227585319922065E-49 ) ) ;
#27468=ORIENTED_EDGE ( 'NONE', *, *, #4798, .F. ) ;
#27472=EDGE_CURVE ( 'NONE', #9737, #20411, #16933, .T. ) ;
#27473=CARTESIAN_POINT ( 'NONE',  ( -410.0000000000000568, -125.0000000000000000, 107.9999999999999858 ) ) ;
#27474=CARTESIAN_POINT ( 'NONE',  ( 11.99999999999999645, -145.0000000000000000, -186.9999999999999716 ) ) ;
#27476=VERTEX_POINT ( 'NONE', #25614 ) ;
#27480=CARTESIAN_POINT ( 'NONE',  ( -15.99999999999998579, -56.99999999999997868, 154.9999999999999716 ) ) ;
#27483=DIRECTION ( 'NONE',  ( -1.232595164407830946E-32, 0.000000000000000000, -1.000000000000000000 ) ) ;
#27486=CARTESIAN_POINT ( 'NONE',  ( -12.00000000000001066, 104.9999999999999858, -175.0000000000000284 ) ) ;
#27490=ORIENTED_EDGE ( 'NONE', *, *, #23967, .T. ) ;
#27491=VECTOR ( 'NONE', #13799, 1000.000000000000000 ) ;
#27498=CARTESIAN_POINT ( 'NONE',  ( -361.0000000000000000, 124.9999999999999432, 183.0000000000000000 ) ) ;
#27502=VECTOR ( 'NONE', #2945, 1000.000000000000000 ) ;
#27503=ORIENTED_EDGE ( 'NONE', *, *, #9771, .T. ) ;
#27507=VERTEX_POINT ( 'NONE', #9252 ) ;
#27509=EDGE_CURVE ( 'NONE', #14780, #16444, #32110, .T. ) ;
#27511=CARTESIAN_POINT ( 'NONE',  ( -355.0000000000000000, 118.9999999999999858, 111.9999999999999858 ) ) ;
#27512=ADVANCED_FACE ( 'NONE', ( #33810 ), #33455, .T. ) ;
#27513=AXIS2_PLACEMENT_3D ( 'NONE', #26009, #28851, #9812 ) ;
#27514=CARTESIAN_POINT ( 'NONE',  ( -418.0000000000000000, -105.0000000000000142, 190.9999999999999716 ) ) ;
#27515=CARTESIAN_POINT ( 'NONE',  ( -20.00000000000007461, 112.9999999999999574, -190.9999999999999716 ) ) ;
#27516=VERTEX_POINT ( 'NONE', #14615 ) ;
#27518=VECTOR ( 'NONE', #15477, 1000.000000000000000 ) ;
#27519=DIRECTION ( 'NONE',  ( 0.000000000000000000, 5.053935297177146739E-49, 1.000000000000000000 ) ) ;
#27520=LINE ( 'NONE', #28312, #16405 ) ;
#27522=CARTESIAN_POINT ( 'NONE',  ( -349.0000000000000000, 124.9999999999999432, 183.0000000000000000 ) ) ;
#27525=DIRECTION ( 'NONE',  ( 1.000000000000000000, 3.469446951953834515E-18, 0.000000000000000000 ) ) ;
#27533=VECTOR ( 'NONE', #13082, 1000.000000000000000 ) ;
#27536=CARTESIAN_POINT ( 'NONE',  ( -418.0000000000000000, 113.0000000000000000, -175.0000000000000000 ) ) ;
#27538=DIRECTION ( 'NONE',  ( 0.000000000000000000, 0.000000000000000000, -1.000000000000000000 ) ) ;
#27544=LINE ( 'NONE', #3508, #34227 ) ;
#27545=CIRCLE ( 'NONE', #32674, 3.999999999999982681 ) ;
#27549=ORIENTED_EDGE ( 'NONE', *, *, #16240, .F. ) ;
#27550=CARTESIAN_POINT ( 'NONE',  ( -361.0000000000000000, 124.9999999999999432, 166.9999999999999716 ) ) ;
#27551=EDGE_CURVE ( 'NONE', #13276, #30004, #22960, .T. ) ;
#27559=EDGE_CURVE ( 'NONE', #16257, #11365, #33630, .T. ) ;
#27561=AXIS2_PLACEMENT_3D ( 'NONE', #19395, #11915, #6187 ) ;
#27565=CIRCLE ( 'NONE', #9391, 4.000000000000003553 ) ;
#27566=ORIENTED_EDGE ( 'NONE', *, *, #25785, .T. ) ;
#27569=EDGE_CURVE ( 'NONE', #20636, #9157, #27938, .T. ) ;
#27570=CARTESIAN_POINT ( 'NONE',  ( -365.0000000000000000, 118.9999999999999716, 111.9999999999999858 ) ) ;
#27577=EDGE_LOOP ( 'NONE', ( #19389, #17317, #1784, #867, #19399, #11851, #27073, #30989 ) ) ;
#27579=CARTESIAN_POINT ( 'NONE',  ( -442.0000000000000000, 105.0000000000000142, 107.9999999999999858 ) ) ;
#27584=AXIS2_PLACEMENT_3D ( 'NONE', #21312, #13312, #19181 ) ;
#27585=VECTOR ( 'NONE', #29057, 1000.000000000000000 ) ;
#27594=AXIS2_PLACEMENT_3D ( 'NONE', #6824, #21056, #2189 ) ;
#27600=DIRECTION ( 'NONE',  ( 0.000000000000000000, 1.000000000000000000, 5.145227585319922065E-49 ) ) ;
#27601=ADVANCED_FACE ( 'NONE', ( #28639 ), #34506, .F. ) ;
#27602=CARTESIAN_POINT ( 'NONE',  ( -349.0000000000000000, -125.0000000000000284, 111.9999999999999858 ) ) ;
#27605=ORIENTED_EDGE ( 'NONE', *, *, #20531, .T. ) ;
#27608=DIRECTION ( 'NONE',  ( 1.000000000000000000, 0.000000000000000000, 0.000000000000000000 ) ) ;
#27611=CYLINDRICAL_SURFACE ( 'NONE', #23379, 4.750000000000004441 ) ;
#27614=DIRECTION ( 'NONE',  ( 1.000000000000000000, 0.000000000000000000, 0.000000000000000000 ) ) ;
#27619=VECTOR ( 'NONE', #8894, 1000.000000000000000 ) ;
#27625=PLANE ( 'NONE',  #8286 ) ;
#27627=LINE ( 'NONE', #10567, #1381 ) ;
#27630=DIRECTION ( 'NONE',  ( 0.000000000000000000, -1.000000000000000000, 6.123233995736766036E-17 ) ) ;
#27632=ADVANCED_FACE ( 'NONE', ( #26493 ), #23308, .T. ) ;
#27633=EDGE_CURVE ( 'NONE', #14045, #30081, #18162, .T. ) ;
#27634=VECTOR ( 'NONE', #20183, 1000.000000000000000 ) ;
#27635=ORIENTED_EDGE ( 'NONE', *, *, #34927, .F. ) ;
#27640=CARTESIAN_POINT ( 'NONE',  ( -418.0000000000000000, 105.0000000000000142, -175.0000000000000000 ) ) ;
#27641=ORIENTED_EDGE ( 'NONE', *, *, #28297, .T. ) ;
#27643=DIRECTION ( 'NONE',  ( 0.000000000000000000, -1.000000000000000000, 6.123233995736766036E-17 ) ) ;
#27644=VECTOR ( 'NONE', #25169, 1000.000000000000000 ) ;
#27646=ORIENTED_EDGE ( 'NONE', *, *, #24953, .F. ) ;
#27649=EDGE_LOOP ( 'NONE', ( #16980, #29537, #14367, #13189 ) ) ;
#27651=EDGE_CURVE ( 'NONE', #24189, #4119, #4243, .T. ) ;
#27655=CARTESIAN_POINT ( 'NONE',  ( -349.0000000000000000, 134.9999999999999716, 128.0000000000000000 ) ) ;
#27658=DIRECTION ( 'NONE',  ( 0.000000000000000000, 1.000000000000000000, -6.123233995736766036E-17 ) ) ;
#27659=CARTESIAN_POINT ( 'NONE',  ( -12.00000000000001066, 144.9999999999999716, 194.9999999999999716 ) ) ;
#27667=VERTEX_POINT ( 'NONE', #21155 ) ;
#27672=EDGE_CURVE ( 'NONE', #28835, #19630, #12813, .T. ) ;
#27674=DIRECTION ( 'NONE',  ( -0.000000000000000000, 1.000000000000000000, -0.000000000000000000 ) ) ;
#27675=DIRECTION ( 'NONE',  ( 0.000000000000000000, 1.000000000000000000, 1.224646799147353207E-16 ) ) ;
#27682=CARTESIAN_POINT ( 'NONE',  ( -499.9999999999999432, -145.0000000000000000, -187.0000000000000000 ) ) ;
#27686=CARTESIAN_POINT ( 'NONE',  ( -19.99999999999998934, 112.9999999999999574, -155.0000000000000000 ) ) ;
#27688=DIRECTION ( 'NONE',  ( 2.891205793294675368E-16, 0.000000000000000000, -1.000000000000000000 ) ) ;
#27690=ORIENTED_EDGE ( 'NONE', *, *, #21100, .T. ) ;
#27694=VECTOR ( 'NONE', #17439, 1000.000000000000000 ) ;
#27696=DIRECTION ( 'NONE',  ( 0.000000000000000000, 0.000000000000000000, 1.000000000000000000 ) ) ;
#27699=CIRCLE ( 'NONE', #32242, 3.999999999999976019 ) ;
#27703=EDGE_CURVE ( 'NONE', #4014, #2214, #26984, .T. ) ;
#27704=DIRECTION ( 'NONE',  ( -0.000000000000000000, 2.309213040847544338E-50, 1.000000000000000000 ) ) ;
#27705=FACE_OUTER_BOUND ( 'NONE', #34534, .T. ) ;
#27709=AXIS2_PLACEMENT_3D ( 'NONE', #31340, #3926, #22990 ) ;
#27710=FACE_BOUND ( 'NONE', #18141, .T. ) ;
#27712=LINE ( 'NONE', #16885, #15647 ) ;
#27718=VERTEX_POINT ( 'NONE', #9773 ) ;
#27720=DIRECTION ( 'NONE',  ( 1.000000000000000000, 0.000000000000000000, 0.000000000000000000 ) ) ;
#27722=PLANE ( 'NONE',  #6948 ) ;
#27724=CIRCLE ( 'NONE', #26017, 7.999999999999986677 ) ;
#27726=LINE ( 'NONE', #11542, #16479 ) ;
#27730=AXIS2_PLACEMENT_3D ( 'NONE', #16222, #9248, #33450 ) ;
#27733=VERTEX_POINT ( 'NONE', #24687 ) ;
#27744=EDGE_LOOP ( 'NONE', ( #28511, #34125, #27255, #24082 ) ) ;
#27745=LINE ( 'NONE', #3360, #21457 ) ;
#27748=ORIENTED_EDGE ( 'NONE', *, *, #1447, .T. ) ;
#27752=CARTESIAN_POINT ( 'NONE',  ( -418.0000000000000000, -125.0000000000000000, 162.9999999999999716 ) ) ;
#27753=ORIENTED_EDGE ( 'NONE', *, *, #5963, .F. ) ;
#27755=EDGE_CURVE ( 'NONE', #14836, #14594, #2802, .T. ) ;
#27756=DIRECTION ( 'NONE',  ( 0.000000000000000000, 0.000000000000000000, 1.000000000000000000 ) ) ;
#27759=STYLED_ITEM('',(#35254),#11234);
#27760=DIRECTION ( 'NONE',  ( 1.000000000000000000, 0.000000000000000000, -1.232595164407831220E-32 ) ) ;
#27761=CARTESIAN_POINT ( 'NONE',  ( -355.0000000000000000, 118.9999999999999716, 109.9999999999999858 ) ) ;
#27764=EDGE_LOOP ( 'NONE', ( #12945, #30202, #20889, #12224 ) ) ;
#27773=AXIS2_PLACEMENT_3D ( 'NONE', #15858, #16872, #13172 ) ;
#27776=ORIENTED_EDGE ( 'NONE', *, *, #20000, .T. ) ;
#27779=CIRCLE ( 'NONE', #5586, 7.999999999999979572 ) ;
#27780=LINE ( 'NONE', #17123, #15030 ) ;
#27786=FACE_OUTER_BOUND ( 'NONE', #22759, .T. ) ;
#27791=CARTESIAN_POINT ( 'NONE',  ( 19.99999999999998224, -55.00000000000000711, -158.9999999999999716 ) ) ;
#27797=DIRECTION ( 'NONE',  ( -1.000000000000000000, 0.000000000000000000, 0.000000000000000000 ) ) ;
#27804=EDGE_CURVE ( 'NONE', #31987, #20636, #13849, .T. ) ;
#27806=ORIENTED_EDGE ( 'NONE', *, *, #11310, .T. ) ;
#27808=EDGE_CURVE ( 'NONE', #2690, #29500, #32707, .T. ) ;
#27814=ORIENTED_EDGE ( 'NONE', *, *, #21303, .F. ) ;
#27815=ORIENTED_EDGE ( 'NONE', *, *, #12425, .T. ) ;
#27820=DIRECTION ( 'NONE',  ( -0.000000000000000000, 1.000000000000000000, -0.000000000000000000 ) ) ;
#27827=ADVANCED_FACE ( 'NONE', ( #29349, #16006, #21340 ), #21513, .F. ) ;
#27829=DIRECTION ( 'NONE',  ( 1.000000000000000000, 3.040835319149746090E-31, 1.232595164407830946E-32 ) ) ;
#27833=DIRECTION ( 'NONE',  ( 0.000000000000000000, -1.000000000000000000, 0.000000000000000000 ) ) ;
#27834=EDGE_CURVE ( 'NONE', #17587, #32711, #21904, .T. ) ;
#27836=ORIENTED_EDGE ( 'NONE', *, *, #18517, .T. ) ;
#27837=CARTESIAN_POINT ( 'NONE',  ( -442.0000000000000000, 144.9999999999999716, -155.0000000000000000 ) ) ;
#27843=LINE ( 'NONE', #25883, #22957 ) ;
#27851=DIRECTION ( 'NONE',  ( 0.000000000000000000, 0.000000000000000000, -1.000000000000000000 ) ) ;
#27852=CYLINDRICAL_SURFACE ( 'NONE', #25665, 3.999999999999976019 ) ;
#27853=EDGE_LOOP ( 'NONE', ( #33254, #24009, #3941, #15385 ) ) ;
#27854=EDGE_CURVE ( 'NONE', #11247, #4608, #30044, .T. ) ;
#27858=ORIENTED_EDGE ( 'NONE', *, *, #34334, .T. ) ;
#27866=DIRECTION ( 'NONE',  ( 0.000000000000000000, 0.000000000000000000, -1.000000000000000000 ) ) ;
#27870=FACE_OUTER_BOUND ( 'NONE', #22173, .T. ) ;
#27874=AXIS2_PLACEMENT_3D ( 'NONE', #21136, #34668, #26470 ) ;
#27876=ORIENTED_EDGE ( 'NONE', *, *, #25785, .F. ) ;
#27878=EDGE_CURVE ( 'NONE', #8166, #4507, #22207, .T. ) ;
#27879=CARTESIAN_POINT ( 'NONE',  ( 11.99999999999995559, -134.9999999999999716, -154.9999999999999716 ) ) ;
#27883=ADVANCED_FACE ( 'NONE', ( #19904 ), #11538, .T. ) ;
#27885=ORIENTED_EDGE ( 'NONE', *, *, #30891, .T. ) ;
#27886=LINE ( 'NONE', #17422, #20739 ) ;
#27889=VERTEX_POINT ( 'NONE', #19372 ) ;
#27898=CYLINDRICAL_SURFACE ( 'NONE', #26697, 7.999999999999979572 ) ;
#27899=ADVANCED_FACE ( 'NONE', ( #19551 ), #503, .T. ) ;
#27900=VERTEX_POINT ( 'NONE', #33584 ) ;
#27904=PLANE ( 'NONE',  #27296 ) ;
#27907=ORIENTED_EDGE ( 'NONE', *, *, #17273, .F. ) ;
#27909=VECTOR ( 'NONE', #26600, 1000.000000000000000 ) ;
#27914=ADVANCED_FACE ( 'NONE', ( #25397 ), #30922, .F. ) ;
#27918=ORIENTED_EDGE ( 'NONE', *, *, #18334, .F. ) ;
#27923=CARTESIAN_POINT ( 'NONE',  ( -442.0000000000000000, -124.9999999999999716, 135.9999999999999716 ) ) ;
#27932=ORIENTED_EDGE ( 'NONE', *, *, #17441, .T. ) ;
#27934=DIRECTION ( 'NONE',  ( 0.000000000000000000, -2.309213040847544338E-50, -1.000000000000000000 ) ) ;
#27935=DIRECTION ( 'NONE',  ( -1.292961597001347186E-16, -0.000000000000000000, 1.000000000000000000 ) ) ;
#27938=LINE ( 'NONE', #6571, #33238 ) ;
#27939=DIRECTION ( 'NONE',  ( 0.000000000000000000, 1.310824597558155437E-49, 1.000000000000000000 ) ) ;
#27942=VERTEX_POINT ( 'NONE', #12075 ) ;
#27946=AXIS2_PLACEMENT_3D ( 'NONE', #6249, #760, #941 ) ;
#27948=VECTOR ( 'NONE', #29678, 1000.000000000000000 ) ;
#27949=CARTESIAN_POINT ( 'NONE',  ( -442.0000000000000000, -112.9999999999999858, -174.9999999999999716 ) ) ;
#27950=VECTOR ( 'NONE', #15091, 1000.000000000000000 ) ;
#27951=ORIENTED_EDGE ( 'NONE', *, *, #27804, .F. ) ;
#27952=VECTOR ( 'NONE', #34904, 1000.000000000000000 ) ;
#27955=ADVANCED_FACE ( 'NONE', ( #6529 ), #17066, .F. ) ;
#27960=ORIENTED_EDGE ( 'NONE', *, *, #10429, .T. ) ;
#27962=DIRECTION ( 'NONE',  ( 1.000000000000000000, 0.000000000000000000, -1.848892746611746966E-32 ) ) ;
#27964=CARTESIAN_POINT ( 'NONE',  ( -442.0000000000000000, 137.0000000000000000, -155.0000000000000000 ) ) ;
#27965=CARTESIAN_POINT ( 'NONE',  ( -418.0000000000000568, -104.9999999999999858, -159.0000000000000000 ) ) ;
#27966=CYLINDRICAL_SURFACE ( 'NONE', #2473, 3.999999999999989786 ) ;
#27971=VERTEX_POINT ( 'NONE', #14568 ) ;
#27974=EDGE_CURVE ( 'NONE', #23491, #34313, #14212, .T. ) ;
#27977=FACE_OUTER_BOUND ( 'NONE', #1133, .T. ) ;
#27979=AXIS2_PLACEMENT_3D ( 'NONE', #9713, #21095, #32122 ) ;
#27981=DIRECTION ( 'NONE',  ( 0.000000000000000000, -0.000000000000000000, 1.000000000000000000 ) ) ;
#27988=EDGE_LOOP ( 'NONE', ( #18609, #23395, #12550, #16060 ) ) ;
#27990=EDGE_LOOP ( 'NONE', ( #28617, #19403, #586, #23773 ) ) ;
#27992=DIRECTION ( 'NONE',  ( 0.000000000000000000, 0.000000000000000000, 1.000000000000000000 ) ) ;
#27998=VECTOR ( 'NONE', #14608, 1000.000000000000000 ) ;
#28007=EDGE_CURVE ( 'NONE', #10470, #6402, #14031, .T. ) ;
#28008=PLANE ( 'NONE',  #14765 ) ;
#28009=DIRECTION ( 'NONE',  ( 0.000000000000000000, 0.000000000000000000, 1.000000000000000000 ) ) ;
#28012=DIRECTION ( 'NONE',  ( 3.040835319149746090E-31, 1.000000000000000000, 0.000000000000000000 ) ) ;
#28017=EDGE_LOOP ( 'NONE', ( #1115, #27176, #26242, #9692 ) ) ;
#28020=DIRECTION ( 'NONE',  ( 0.000000000000000000, 0.000000000000000000, 1.000000000000000000 ) ) ;
#28022=DIRECTION ( 'NONE',  ( 0.000000000000000000, 0.000000000000000000, 1.000000000000000000 ) ) ;
#28023=DIRECTION ( 'NONE',  ( 0.000000000000000000, 0.000000000000000000, -1.000000000000000000 ) ) ;
#28024=DIRECTION ( 'NONE',  ( 0.000000000000000000, 1.224646799147353207E-16, -1.000000000000000000 ) ) ;
#28029=EDGE_CURVE ( 'NONE', #16015, #16248, #15613, .T. ) ;
#28034=CARTESIAN_POINT ( 'NONE',  ( -15.99999999999998579, -124.9999999999999432, -162.9999999999999432 ) ) ;
#28035=VERTEX_POINT ( 'NONE', #15266 ) ;
#28040=ORIENTED_EDGE ( 'NONE', *, *, #3989, .T. ) ;
#28041=DIRECTION ( 'NONE',  ( 0.000000000000000000, 0.000000000000000000, 1.000000000000000000 ) ) ;
#28043=VECTOR ( 'NONE', #17889, 1000.000000000000000 ) ;
#28044=CARTESIAN_POINT ( 'NONE',  ( -499.9999999999999432, 112.9999999999999574, 162.9999999999999716 ) ) ;
#28045=DIRECTION ( 'NONE',  ( 0.000000000000000000, 1.000000000000000000, 0.000000000000000000 ) ) ;
#28051=DIRECTION ( 'NONE',  ( 0.000000000000000000, -1.000000000000000000, -2.465190328815662439E-32 ) ) ;
#28052=CARTESIAN_POINT ( 'NONE',  ( 15.99999999999997868, 144.9999999999999716, 187.0000000000000000 ) ) ;
#28054=DIRECTION ( 'NONE',  ( -1.000000000000000000, 0.000000000000000000, -5.546364386991661285E-52 ) ) ;
#28055=VECTOR ( 'NONE', #8619, 1000.000000000000000 ) ;
#28057=EDGE_CURVE ( 'NONE', #2660, #13396, #7222, .T. ) ;
#28058=VECTOR ( 'NONE', #27405, 1000.000000000000000 ) ;
#28059=DIRECTION ( 'NONE',  ( -1.848892746611746419E-32, -6.842277657836020854E-49, 1.000000000000000000 ) ) ;
#28062=LINE ( 'NONE', #31093, #13759 ) ;
#28064=ORIENTED_EDGE ( 'NONE', *, *, #20693, .T. ) ;
#28068=EDGE_CURVE ( 'NONE', #14836, #1154, #24739, .T. ) ;
#28070=ORIENTED_EDGE ( 'NONE', *, *, #22490, .T. ) ;
#28073=CARTESIAN_POINT ( 'NONE',  ( -500.0000000000000000, -113.0000000000000000, -155.0000000000000000 ) ) ;
#28074=EDGE_CURVE ( 'NONE', #15074, #16015, #34108, .T. ) ;
#28076=EDGE_CURVE ( 'NONE', #14266, #18467, #1718, .T. ) ;
#28079=AXIS2_PLACEMENT_3D ( 'NONE', #3769, #3933, #22820 ) ;
#28083=ORIENTED_EDGE ( 'NONE', *, *, #26217, .F. ) ;
#28088=ORIENTED_EDGE ( 'NONE', *, *, #4096, .F. ) ;
#28094=DIRECTION ( 'NONE',  ( -1.000000000000000000, 0.000000000000000000, -1.300283923313630633E-47 ) ) ;
#28098=ADVANCED_FACE ( 'NONE', ( #25934 ), #1551, .F. ) ;
#28102=VECTOR ( 'NONE', #22631, 1000.000000000000000 ) ;
#28103=DIRECTION ( 'NONE',  ( -0.000000000000000000, -1.000000000000000000, -0.000000000000000000 ) ) ;
#28105=ORIENTED_EDGE ( 'NONE', *, *, #3009, .F. ) ;
#28106=VERTEX_POINT ( 'NONE', #7349 ) ;
#28110=DIRECTION ( 'NONE',  ( 0.000000000000000000, -1.000000000000000000, -5.053935297177146739E-49 ) ) ;
#28113=( NAMED_UNIT ( * ) PLANE_ANGLE_UNIT ( ) SI_UNIT ( $, .RADIAN. ) );
#28114=AXIS2_PLACEMENT_3D ( 'NONE', #14667, #30671, #8769 ) ;
#28118=DIRECTION ( 'NONE',  ( -1.000000000000000000, -3.040835319149746090E-31, 1.232595164407830946E-32 ) ) ;
#28119=VERTEX_POINT ( 'NONE', #18125 ) ;
#28123=EDGE_LOOP ( 'NONE', ( #9236, #17043, #7065, #29690 ) ) ;
#28126=AXIS2_PLACEMENT_3D ( 'NONE', #17972, #31464, #34129 ) ;
#28127=ORIENTED_EDGE ( 'NONE', *, *, #17635, .F. ) ;
#28128=CARTESIAN_POINT ( 'NONE',  ( 11.99999999999999645, 134.9999999999998863, 155.0000000000000000 ) ) ;
#28130=CIRCLE ( 'NONE', #33821, 7.999999999999979572 ) ;
#28131=LINE ( 'NONE', #14628, #18203 ) ;
#28136=CARTESIAN_POINT ( 'NONE',  ( -499.9999999999999432, 104.9999999999999858, -162.9999999999999716 ) ) ;
#28138=DIRECTION ( 'NONE',  ( 1.000000000000000000, 3.040835319149746528E-31, 1.232595164407830946E-32 ) ) ;
#28143=CYLINDRICAL_SURFACE ( 'NONE', #25562, 3.999999999999976019 ) ;
#28146=ORIENTED_EDGE ( 'NONE', *, *, #33067, .T. ) ;
#28148=VECTOR ( 'NONE', #5172, 1000.000000000000000 ) ;
#28150=VECTOR ( 'NONE', #18109, 1000.000000000000000 ) ;
#28152=AXIS2_PLACEMENT_3D ( 'NONE', #19710, #30728, #30558 ) ;
#28153=CARTESIAN_POINT ( 'NONE',  ( 11.99999999999999645, 124.9999999999999716, 194.9999999999999716 ) ) ;
#28154=DIRECTION ( 'NONE',  ( 0.000000000000000000, 0.000000000000000000, -1.000000000000000000 ) ) ;
#28166=EDGE_CURVE ( 'NONE', #21633, #6559, #25753, .T. ) ;
#28171=ORIENTED_EDGE ( 'NONE', *, *, #23202, .T. ) ;
#28174=DIRECTION ( 'NONE',  ( 0.000000000000000000, 0.000000000000000000, 1.000000000000000000 ) ) ;
#28176=VERTEX_POINT ( 'NONE', #21634 ) ;
#28177=CARTESIAN_POINT ( 'NONE',  ( -430.0000000000000000, -119.0000000000000000, 130.0000000000000000 ) ) ;
#28178=AXIS2_PLACEMENT_3D ( 'NONE', #16650, #27833, #22150 ) ;
#28181=PLANE ( 'NONE',  #14095 ) ;
#28184=ORIENTED_EDGE ( 'NONE', *, *, #9241, .F. ) ;
#28192=ORIENTED_EDGE ( 'NONE', *, *, #21608, .T. ) ;
#28196=LINE ( 'NONE', #14692, #33280 ) ;
#28199=DIRECTION ( 'NONE',  ( 0.000000000000000000, 0.000000000000000000, -1.000000000000000000 ) ) ;
#28206=CARTESIAN_POINT ( 'NONE',  ( -349.0000000000000000, -125.0000000000000284, 126.0000000000000000 ) ) ;
#28209=EDGE_CURVE ( 'NONE', #30170, #18484, #23946, .T. ) ;
#28213=AXIS2_PLACEMENT_3D ( 'NONE', #29300, #15260, #17941 ) ;
#28216=EDGE_CURVE ( 'NONE', #10965, #27900, #33621, .T. ) ;
#28219=ORIENTED_EDGE ( 'NONE', *, *, #20341, .T. ) ;
#28227=CARTESIAN_POINT ( 'NONE',  ( -442.0000000000000000, -104.9999999999999858, -162.9999999999999716 ) ) ;
#28228=PLANE ( 'NONE',  #24490 ) ;
#28235=AXIS2_PLACEMENT_3D ( 'NONE', #15249, #26257, #9378 ) ;
#28236=DIRECTION ( 'NONE',  ( -0.000000000000000000, 0.000000000000000000, 1.000000000000000000 ) ) ;
#28242=FACE_OUTER_BOUND ( 'NONE', #4580, .T. ) ;
#28245=ORIENTED_EDGE ( 'NONE', *, *, #3463, .F. ) ;
#28246=LINE ( 'NONE', #22561, #16100 ) ;
#28253=DIRECTION ( 'NONE',  ( -0.000000000000000000, -0.000000000000000000, -1.000000000000000000 ) ) ;
#28255=PLANE ( 'NONE',  #29118 ) ;
#28257=ORIENTED_EDGE ( 'NONE', *, *, #22152, .T. ) ;
#28269=EDGE_LOOP ( 'NONE', ( #299, #9198, #14988, #6705 ) ) ;
#28271=VERTEX_POINT ( 'NONE', #26624 ) ;
#28273=CARTESIAN_POINT ( 'NONE',  ( -442.0000000000000000, 105.0000000000000142, -175.0000000000000000 ) ) ;
#28278=AXIS2_PLACEMENT_3D ( 'NONE', #34945, #7693, #29243 ) ;
#28279=CARTESIAN_POINT ( 'NONE',  ( -12.00000000000001066, -145.0000000000000000, 159.0000000000000000 ) ) ;
#28281=ORIENTED_EDGE ( 'NONE', *, *, #13293, .T. ) ;
#28283=DIRECTION ( 'NONE',  ( 0.000000000000000000, -1.131431318426415506E-52, -1.000000000000000000 ) ) ;
#28284=ORIENTED_EDGE ( 'NONE', *, *, #8908, .F. ) ;
#28285=ADVANCED_FACE ( 'NONE', ( #24119 ), #18804, .F. ) ;
#28286=CARTESIAN_POINT ( 'NONE',  ( -499.9999999999999432, 136.9999999999999432, -190.9999999999999716 ) ) ;
#28290=EDGE_CURVE ( 'NONE', #32869, #19981, #25354, .T. ) ;
#28293=CIRCLE ( 'NONE', #32726, 3.999999999999976019 ) ;
#28294=DIRECTION ( 'NONE',  ( 0.000000000000000000, 1.310824597558155437E-49, 1.000000000000000000 ) ) ;
#28297=EDGE_CURVE ( 'NONE', #20392, #23064, #6129, .T. ) ;
#28299=AXIS2_PLACEMENT_3D ( 'NONE', #20232, #30724, #33740 ) ;
#28304=VECTOR ( 'NONE', #18190, 1000.000000000000000 ) ;
#28305=ORIENTED_EDGE ( 'NONE', *, *, #16602, .F. ) ;
#28307=ADVANCED_FACE ( 'NONE', ( #986 ), #19331, .F. ) ;
#28310=VERTEX_POINT ( 'NONE', #629 ) ;
#28312=CARTESIAN_POINT ( 'NONE',  ( -12.00000000000001066, -124.9999999999999432, -154.9999999999999716 ) ) ;
#28326=ORIENTED_EDGE ( 'NONE', *, *, #22349, .T. ) ;
#28329=DIRECTION ( 'NONE',  ( -1.000000000000000000, 0.000000000000000000, -5.546364386991661285E-52 ) ) ;
#28332=ORIENTED_EDGE ( 'NONE', *, *, #26475, .T. ) ;
#28335=ADVANCED_FACE ( 'NONE', ( #22706 ), #27852, .F. ) ;
#28338=LINE ( 'NONE', #33850, #23034 ) ;
#28347=AXIS2_PLACEMENT_3D ( 'NONE', #15495, #15147, #7636 ) ;
#28348=EDGE_LOOP ( 'NONE', ( #28436, #21363, #16952, #8911 ) ) ;
#28352=CARTESIAN_POINT ( 'NONE',  ( 19.99999999999998934, 4.559999999999908127, -172.9900000000000091 ) ) ;
#28353=ORIENTED_EDGE ( 'NONE', *, *, #16373, .T. ) ;
#28356=ADVANCED_FACE ( 'NONE', ( #22168 ), #20038, .F. ) ;
#28367=LINE ( 'NONE', #28707, #19868 ) ;
#28369=DIRECTION ( 'NONE',  ( -3.469446951953832974E-18, -1.000000000000000000, -7.888609052210116302E-31 ) ) ;
#28372=PLANE ( 'NONE',  #13491 ) ;
#28376=ORIENTED_EDGE ( 'NONE', *, *, #1542, .T. ) ;
#28380=DIRECTION ( 'NONE',  ( 0.000000000000000000, 1.000000000000000000, -3.374343856708137958E-53 ) ) ;
#28381=LINE ( 'NONE', #12015, #33802 ) ;
#28382=DIRECTION ( 'NONE',  ( 0.000000000000000000, 0.000000000000000000, 1.000000000000000000 ) ) ;
#28385=EDGE_LOOP ( 'NONE', ( #34653, #26280, #30661, #7102 ) ) ;
#28386=DIRECTION ( 'NONE',  ( 1.000000000000000000, 3.040835319149746528E-31, 1.232595164407830946E-32 ) ) ;
#28388=CARTESIAN_POINT ( 'NONE',  ( -12.00000000000001066, -124.9999999999999432, -154.9999999999999716 ) ) ;
#28391=ORIENTED_EDGE ( 'NONE', *, *, #28841, .T. ) ;
#28398=VERTEX_POINT ( 'NONE', #30533 ) ;
#28402=DIRECTION ( 'NONE',  ( -1.000000000000000000, 0.000000000000000000, 1.232595164407831220E-32 ) ) ;
#28405=ORIENTED_EDGE ( 'NONE', *, *, #12465, .T. ) ;
#28407=LINE ( 'NONE', #1354, #14572 ) ;
#28409=CARTESIAN_POINT ( 'NONE',  ( -20.00000000000007461, -109.0000000000000142, -162.9999999999999716 ) ) ;
#28411=CARTESIAN_POINT ( 'NONE',  ( -499.9999999999999432, -113.0000000000000000, -187.0000000000000000 ) ) ;
#28416=CARTESIAN_POINT ( 'NONE',  ( -449.9999999999999432, 124.9999999999999432, -162.9999999999999716 ) ) ;
#28417=VERTEX_POINT ( 'NONE', #26710 ) ;
#28419=DIRECTION ( 'NONE',  ( -0.000000000000000000, -0.000000000000000000, -1.000000000000000000 ) ) ;
#28420=CARTESIAN_POINT ( 'NONE',  ( -442.0000000000000000, 105.0000000000000142, 107.9999999999999858 ) ) ;
#28421=DIRECTION ( 'NONE',  ( 0.000000000000000000, 2.465190328815661892E-32, 1.000000000000000000 ) ) ;
#28422=VERTEX_POINT ( 'NONE', #28906 ) ;
#28424=ORIENTED_EDGE ( 'NONE', *, *, #6531, .T. ) ;
#28428=ORIENTED_EDGE ( 'NONE', *, *, #5810, .T. ) ;
#28432=ORIENTED_EDGE ( 'NONE', *, *, #440, .T. ) ;
#28436=ORIENTED_EDGE ( 'NONE', *, *, #24584, .F. ) ;
#28443=ORIENTED_EDGE ( 'NONE', *, *, #809, .T. ) ;
#28445=EDGE_CURVE ( 'NONE', #22809, #11184, #34771, .T. ) ;
#28446=DIRECTION ( 'NONE',  ( -1.000000000000000000, -3.469446951953834515E-18, 2.736911063134582149E-48 ) ) ;
#28447=DIRECTION ( 'NONE',  ( -0.000000000000000000, -1.000000000000000000, -0.000000000000000000 ) ) ;
#28448=CYLINDRICAL_SURFACE ( 'NONE', #4629, 3.999999999999982681 ) ;
#28449=CARTESIAN_POINT ( 'NONE',  ( -15.99999999999998579, -145.0000000000000000, -162.9999999999999432 ) ) ;
#28452=EDGE_CURVE ( 'NONE', #392, #32678, #9524, .T. ) ;
#28455=CIRCLE ( 'NONE', #2292, 7.999999999999979572 ) ;
#28457=DIRECTION ( 'NONE',  ( -1.000000000000000000, 0.000000000000000000, 0.000000000000000000 ) ) ;
#28462=CARTESIAN_POINT ( 'NONE',  ( -20.00000000000001776, -109.0000000000000142, 162.9999999999999716 ) ) ;
#28464=LINE ( 'NONE', #12630, #27518 ) ;
#28470=LINE ( 'NONE', #1419, #33638 ) ;
#28475=AXIS2_PLACEMENT_3D ( 'NONE', #1698, #9705, #23250 ) ;
#28476=VERTEX_POINT ( 'NONE', #1507 ) ;
#28477=AXIS2_PLACEMENT_3D ( 'NONE', #250, #24611, #3084 ) ;
#28478=DIRECTION ( 'NONE',  ( -1.000000000000000000, 0.000000000000000000, 1.848892746611746966E-32 ) ) ;
#28480=EDGE_CURVE ( 'NONE', #10477, #15683, #9688, .T. ) ;
#28489=VERTEX_POINT ( 'NONE', #7007 ) ;
#28490=EDGE_LOOP ( 'NONE', ( #6253, #6153, #21638, #4445 ) ) ;
#28492=VECTOR ( 'NONE', #26883, 1000.000000000000000 ) ;
#28493=AXIS2_PLACEMENT_3D ( 'NONE', #93, #2581, #18976 ) ;
#28494=DIRECTION ( 'NONE',  ( 0.000000000000000000, -1.131431318426415506E-52, -1.000000000000000000 ) ) ;
#28496=ORIENTED_EDGE ( 'NONE', *, *, #7283, .F. ) ;
#28501=ORIENTED_EDGE ( 'NONE', *, *, #5568, .F. ) ;
#28502=AXIS2_PLACEMENT_3D ( 'NONE', #15023, #2180, #23365 ) ;
#28504=CARTESIAN_POINT ( 'NONE',  ( -11.99999999999998224, -134.9999999999999716, 187.0000000000000000 ) ) ;
#28511=ORIENTED_EDGE ( 'NONE', *, *, #887, .F. ) ;
#28513=PLANE ( 'NONE',  #29652 ) ;
#28518=AXIS2_PLACEMENT_3D ( 'NONE', #28504, #14467, #28154 ) ;
#28524=CARTESIAN_POINT ( 'NONE',  ( -499.9999999999999432, 104.9999999999999858, 187.0000000000000000 ) ) ;
#28525=ORIENTED_EDGE ( 'NONE', *, *, #6753, .F. ) ;
#28526=EDGE_LOOP ( 'NONE', ( #35050, #24706, #877, #24069, #11347, #31254, #26537, #16915 ) ) ;
#28528=CARTESIAN_POINT ( 'NONE',  ( -19.99999999999998934, 144.9999999999999716, -186.9999999999999716 ) ) ;
#28532=VERTEX_POINT ( 'NONE', #16057 ) ;
#28535=ORIENTED_EDGE ( 'NONE', *, *, #24939, .T. ) ;
#28537=CARTESIAN_POINT ( 'NONE',  ( -12.00000000000003908, -134.9999999999999716, -194.9999999999999432 ) ) ;
#28545=DIRECTION ( 'NONE',  ( -1.000000000000000000, 0.000000000000000000, -1.300283923313630633E-47 ) ) ;
#28546=ORIENTED_EDGE ( 'NONE', *, *, #24293, .F. ) ;
#28548=AXIS2_PLACEMENT_3D ( 'NONE', #28810, #9945, #18159 ) ;
#28552=CARTESIAN_POINT ( 'NONE',  ( -20.00000000000004619, -137.0000000000000000, -162.9999999999999716 ) ) ;
#28553=DIRECTION ( 'NONE',  ( -3.469446951953832974E-18, -1.000000000000000000, -7.888609052210116302E-31 ) ) ;
#28554=DIRECTION ( 'NONE',  ( 0.000000000000000000, -0.000000000000000000, -1.000000000000000000 ) ) ;
#28557=DIRECTION ( 'NONE',  ( 0.000000000000000000, 1.310824597558155437E-49, 1.000000000000000000 ) ) ;
#28558=CARTESIAN_POINT ( 'NONE',  ( -349.0000000000000000, -135.0000000000000000, 128.0000000000000000 ) ) ;
#28565=EDGE_CURVE ( 'NONE', #7091, #25547, #21675, .T. ) ;
#28566=AXIS2_PLACEMENT_3D ( 'NONE', #26579, #2200, #13073 ) ;
#28570=CIRCLE ( 'NONE', #8666, 7.999999999999979572 ) ;
#28571=VERTEX_POINT ( 'NONE', #8192 ) ;
#28572=CARTESIAN_POINT ( 'NONE',  ( 11.99999999999999645, -141.0000000000000000, -155.0000000000000284 ) ) ;
#28573=ORIENTED_EDGE ( 'NONE', *, *, #20266, .T. ) ;
#28576=LINE ( 'NONE', #19263, #26664 ) ;
#28577=CARTESIAN_POINT ( 'NONE',  ( 11.99999999999995559, -145.0000000000000000, 194.9999999999999716 ) ) ;
#28579=ORIENTED_EDGE ( 'NONE', *, *, #20000, .F. ) ;
#28580=ORIENTED_EDGE ( 'NONE', *, *, #32146, .T. ) ;
#28583=DIRECTION ( 'NONE',  ( -1.000000000000000000, 0.000000000000000000, -1.300283923313630633E-47 ) ) ;
#28584=LINE ( 'NONE', #17577, #20975 ) ;
#28586=CARTESIAN_POINT ( 'NONE',  ( -12.00000000000001066, -112.9999999999999858, -155.0000000000000284 ) ) ;
#28592=CARTESIAN_POINT ( 'NONE',  ( -70.00000000000000000, 4.559999999999908127, 172.9900000000000091 ) ) ;
#28593=ORIENTED_EDGE ( 'NONE', *, *, #8387, .F. ) ;
#28597=DIRECTION ( 'NONE',  ( -0.000000000000000000, 1.000000000000000000, -0.000000000000000000 ) ) ;
#28599=CARTESIAN_POINT ( 'NONE',  ( -12.00000000000001066, 144.9999999999999716, -175.0000000000000284 ) ) ;
#28611=LINE ( 'NONE', #20265, #34912 ) ;
#28613=LINE ( 'NONE', #4550, #7888 ) ;
#28614=VECTOR ( 'NONE', #14021, 1000.000000000000000 ) ;
#28617=ORIENTED_EDGE ( 'NONE', *, *, #13495, .F. ) ;
#28618=ORIENTED_EDGE ( 'NONE', *, *, #27569, .T. ) ;
#28619=VECTOR ( 'NONE', #11759, 1000.000000000000000 ) ;
#28620=ORIENTED_EDGE ( 'NONE', *, *, #31740, .F. ) ;
#28624=CARTESIAN_POINT ( 'NONE',  ( -410.0000000000000568, 137.0000000000000000, -155.0000000000000000 ) ) ;
#28625=DIRECTION ( 'NONE',  ( 0.000000000000000000, 1.000000000000000000, -3.374343856708137958E-53 ) ) ;
#28627=VERTEX_POINT ( 'NONE', #10874 ) ;
#28629=VERTEX_POINT ( 'NONE', #24387 ) ;
#28630=AXIS2_PLACEMENT_3D ( 'NONE', #3226, #568, #22280 ) ;
#28631=DIRECTION ( 'NONE',  ( 0.000000000000000000, -1.310824597558155437E-49, -1.000000000000000000 ) ) ;
#28633=DIRECTION ( 'NONE',  ( 1.000000000000000000, 3.040835319149746090E-31, 1.232595164407830946E-32 ) ) ;
#28639=FACE_OUTER_BOUND ( 'NONE', #7132, .T. ) ;
#28640=CARTESIAN_POINT ( 'NONE',  ( -361.0000000000000000, -125.0000000000000284, 112.0000000000000000 ) ) ;
#28648=EDGE_CURVE ( 'NONE', #33070, #7332, #13898, .T. ) ;
#28650=AXIS2_PLACEMENT_3D ( 'NONE', #7229, #31280, #15445 ) ;
#28653=EDGE_CURVE ( 'NONE', #27112, #19297, #377, .T. ) ;
#28655=ORIENTED_EDGE ( 'NONE', *, *, #4130, .F. ) ;
#28657=DIRECTION ( 'NONE',  ( -1.000000000000000000, 0.000000000000000000, 0.000000000000000000 ) ) ;
#28661=DIRECTION ( 'NONE',  ( 0.000000000000000000, 0.000000000000000000, -1.000000000000000000 ) ) ;
#28665=VERTEX_POINT ( 'NONE', #21903 ) ;
#28667=CARTESIAN_POINT ( 'NONE',  ( 11.99999999999999645, 144.9999999999999147, 162.9999999999999716 ) ) ;
#28671=ORIENTED_EDGE ( 'NONE', *, *, #22428, .F. ) ;
#28679=FACE_OUTER_BOUND ( 'NONE', #5516, .T. ) ;
#28682=CARTESIAN_POINT ( 'NONE',  ( -12.00000000000001066, 124.9999999999999716, 155.0000000000000000 ) ) ;
#28683=CIRCLE ( 'NONE', #1977, 3.999999999999976019 ) ;
#28684=DIRECTION ( 'NONE',  ( 0.000000000000000000, 0.000000000000000000, -1.000000000000000000 ) ) ;
#28686=AXIS2_PLACEMENT_3D ( 'NONE', #19941, #17288, #11938 ) ;
#28688=ORIENTED_EDGE ( 'NONE', *, *, #16889, .T. ) ;
#28692=EDGE_CURVE ( 'NONE', #31670, #21641, #3527, .T. ) ;
#28696=DIRECTION ( 'NONE',  ( -0.000000000000000000, 1.000000000000000000, -0.000000000000000000 ) ) ;
#28698=CIRCLE ( 'NONE', #32096, 4.000000000000003553 ) ;
#28701=FACE_BOUND ( 'NONE', #16695, .T. ) ;
#28702=ORIENTED_EDGE ( 'NONE', *, *, #22058, .F. ) ;
#28705=FACE_OUTER_BOUND ( 'NONE', #26808, .T. ) ;
#28706=VECTOR ( 'NONE', #2053, 1000.000000000000000 ) ;
#28707=CARTESIAN_POINT ( 'NONE',  ( -70.00000000000000000, 4.559999999999908127, -177.7400000000000091 ) ) ;
#28709=ADVANCED_FACE ( 'NONE', ( #1398 ), #20447, .F. ) ;
#28710=CARTESIAN_POINT ( 'NONE',  ( -414.0000000000000568, -112.9999999999999858, -174.9999999999999716 ) ) ;
#28711=VERTEX_POINT ( 'NONE', #28624 ) ;
#28714=CARTESIAN_POINT ( 'NONE',  ( -442.0000000000000000, -105.0000000000000142, -109.9999999999999574 ) ) ;
#28716=AXIS2_PLACEMENT_3D ( 'NONE', #9678, #13062, #23217 ) ;
#28718=LINE ( 'NONE', #1, #24582 ) ;
#28721=CARTESIAN_POINT ( 'NONE',  ( -499.9999999999999432, 108.9999999999999858, -187.0000000000000000 ) ) ;
#28722=LINE ( 'NONE', #20884, #13904 ) ;
#28725=DIRECTION ( 'NONE',  ( 0.000000000000000000, -1.000000000000000000, -2.309213040847544338E-50 ) ) ;
#28728=DIRECTION ( 'NONE',  ( 1.000000000000000000, -0.000000000000000000, -0.000000000000000000 ) ) ;
#28735=AXIS2_PLACEMENT_3D ( 'NONE', #34942, #24057, #12886 ) ;
#28738=ORIENTED_EDGE ( 'NONE', *, *, #31263, .T. ) ;
#28739=DIRECTION ( 'NONE',  ( 1.000000000000000000, 0.000000000000000000, -1.848892746611746966E-32 ) ) ;
#28741=ORIENTED_EDGE ( 'NONE', *, *, #9161, .F. ) ;
#28742=DIRECTION ( 'NONE',  ( 0.000000000000000000, 1.000000000000000000, 0.000000000000000000 ) ) ;
#28743=CIRCLE ( 'NONE', #25330, 4.000000000000003553 ) ;
#28744=DIRECTION ( 'NONE',  ( -3.040835319149746090E-31, -1.000000000000000000, 0.000000000000000000 ) ) ;
#28745=CYLINDRICAL_SURFACE ( 'NONE', #22816, 3.999999999999976019 ) ;
#28748=DIRECTION ( 'NONE',  ( 0.000000000000000000, -1.000000000000000000, 3.421138828918010427E-49 ) ) ;
#28749=LINE ( 'NONE', #1175, #20321 ) ;
#28750=CARTESIAN_POINT ( 'NONE',  ( 11.99999999999999645, 124.9999999999999716, 155.0000000000000000 ) ) ;
#28751=DIRECTION ( 'NONE',  ( 0.000000000000000000, 0.000000000000000000, 1.000000000000000000 ) ) ;
#28752=DIRECTION ( 'NONE',  ( 0.000000000000000000, 0.000000000000000000, -1.000000000000000000 ) ) ;
#28758=CIRCLE ( 'NONE', #23653, 2.000000000000001776 ) ;
#28766=CYLINDRICAL_SURFACE ( 'NONE', #8127, 4.000000000000003553 ) ;
#28768=DIRECTION ( 'NONE',  ( 0.000000000000000000, 1.131431318426415506E-52, 1.000000000000000000 ) ) ;
#28772=AXIS2_PLACEMENT_3D ( 'NONE', #31076, #22720, #14542 ) ;
#28781=LINE ( 'NONE', #26456, #10211 ) ;
#28783=AXIS2_PLACEMENT_3D ( 'NONE', #30113, #6064, #24238 ) ;
#28784=DIRECTION ( 'NONE',  ( 0.000000000000000000, 0.000000000000000000, 1.000000000000000000 ) ) ;
#28792=CARTESIAN_POINT ( 'NONE',  ( -19.99999999999998934, 4.559999999999908127, -172.9900000000000091 ) ) ;
#28793=VECTOR ( 'NONE', #8233, 1000.000000000000000 ) ;
#28795=CARTESIAN_POINT ( 'NONE',  ( -15.99999999999998579, 124.9999999999999716, 187.0000000000000000 ) ) ;
#28796=DIRECTION ( 'NONE',  ( -1.000000000000000000, 0.000000000000000000, 0.000000000000000000 ) ) ;
#28797=PLANE ( 'NONE',  #12357 ) ;
#28801=AXIS2_PLACEMENT_3D ( 'NONE', #9978, #29012, #4607 ) ;
#28804=EDGE_CURVE ( 'NONE', #12748, #14760, #31847, .T. ) ;
#28805=ORIENTED_EDGE ( 'NONE', *, *, #30594, .F. ) ;
#28807=EDGE_CURVE ( 'NONE', #31407, #763, #7482, .T. ) ;
#28810=CARTESIAN_POINT ( 'NONE',  ( -12.00000000000003908, -134.9999999999999716, -162.9999999999999432 ) ) ;
#28812=DIRECTION ( 'NONE',  ( 1.000000000000000000, 0.000000000000000000, -1.848892746611746966E-32 ) ) ;
#28815=ORIENTED_EDGE ( 'NONE', *, *, #6455, .T. ) ;
#28819=AXIS2_PLACEMENT_3D ( 'NONE', #7738, #25778, #1407 ) ;
#28821=AXIS2_PLACEMENT_3D ( 'NONE', #16692, #24147, #24320 ) ;
#28826=LINE ( 'NONE', #27336, #6569 ) ;
#28829=CARTESIAN_POINT ( 'NONE',  ( -20.00000000000004619, -113.0000000000000000, -194.9999999999999432 ) ) ;
#28831=ORIENTED_EDGE ( 'NONE', *, *, #19077, .F. ) ;
#28834=ADVANCED_FACE ( 'NONE', ( #875 ), #28448, .F. ) ;
#28835=VERTEX_POINT ( 'NONE', #9418 ) ;
#28836=ADVANCED_FACE ( 'NONE', ( #17620 ), #2094, .T. ) ;
#28838=DIRECTION ( 'NONE',  ( -0.000000000000000000, 1.000000000000000000, -0.000000000000000000 ) ) ;
#28840=DIRECTION ( 'NONE',  ( 0.000000000000000000, 0.000000000000000000, 1.000000000000000000 ) ) ;
#28841=EDGE_CURVE ( 'NONE', #19925, #4470, #1180, .T. ) ;
#28843=ORIENTED_EDGE ( 'NONE', *, *, #23003, .T. ) ;
#28845=CARTESIAN_POINT ( 'NONE',  ( -499.9999999999999432, -113.0000000000000000, -190.9999999999999716 ) ) ;
#28848=CARTESIAN_POINT ( 'NONE',  ( -347.0000000000000000, -125.0000000000000284, 181.0000000000000000 ) ) ;
#28851=DIRECTION ( 'NONE',  ( -0.000000000000000000, -0.000000000000000000, -1.000000000000000000 ) ) ;
#28852=CARTESIAN_POINT ( 'NONE',  ( -418.0000000000000000, 104.9999999999999858, -190.9999999999999716 ) ) ;
#28853=DIRECTION ( 'NONE',  ( -1.000000000000000000, 0.000000000000000000, -5.546364386991661285E-52 ) ) ;
#28856=ADVANCED_FACE ( 'NONE', ( #26651 ), #26824, .F. ) ;
#28861=VERTEX_POINT ( 'NONE', #34488 ) ;
#28865=VERTEX_POINT ( 'NONE', #5098 ) ;
#28869=AXIS2_PLACEMENT_3D ( 'NONE', #34711, #8000, #27051 ) ;
#28871=EDGE_LOOP ( 'NONE', ( #13008, #21032, #12480, #28353 ) ) ;
#28873=CARTESIAN_POINT ( 'NONE',  ( 19.99999999999998934, -124.9999999999999432, -186.9999999999999716 ) ) ;
#28875=VERTEX_POINT ( 'NONE', #4922 ) ;
#28879=LINE ( 'NONE', #4479, #30183 ) ;
#28881=VERTEX_POINT ( 'NONE', #18661 ) ;
#28882=VECTOR ( 'NONE', #16251, 1000.000000000000000 ) ;
#28885=CARTESIAN_POINT ( 'NONE',  ( 19.99999999999998934, 4.559999999999909015, -168.2400000000000091 ) ) ;
#28887=EDGE_CURVE ( 'NONE', #33691, #15781, #29095, .T. ) ;
#28888=FACE_OUTER_BOUND ( 'NONE', #5800, .T. ) ;
#28890=ADVANCED_FACE ( 'NONE', ( #10460, #23636, #7070 ), #2261, .F. ) ;
#28891=AXIS2_PLACEMENT_3D ( 'NONE', #34004, #6594, #920 ) ;
#28896=ADVANCED_FACE ( 'NONE', ( #13135 ), #12446, .F. ) ;
#28898=CARTESIAN_POINT ( 'NONE',  ( 11.99999999999999645, 140.9999999999999716, 155.0000000000000000 ) ) ;
#28902=LINE ( 'NONE', #7707, #22556 ) ;
#28904=ORIENTED_EDGE ( 'NONE', *, *, #19305, .T. ) ;
#28906=CARTESIAN_POINT ( 'NONE',  ( 11.99999999999995559, -145.0000000000000000, -154.9999999999999716 ) ) ;
#28908=EDGE_CURVE ( 'NONE', #22409, #29056, #12543, .T. ) ;
#28909=AXIS2_PLACEMENT_3D ( 'NONE', #18663, #13137, #21831 ) ;
#28910=ORIENTED_EDGE ( 'NONE', *, *, #19154, .F. ) ;
#28912=ORIENTED_EDGE ( 'NONE', *, *, #367, .F. ) ;
#28913=ORIENTED_EDGE ( 'NONE', *, *, #22745, .F. ) ;
#28914=DIRECTION ( 'NONE',  ( 0.000000000000000000, 0.000000000000000000, 1.000000000000000000 ) ) ;
#28915=EDGE_CURVE ( 'NONE', #24841, #9803, #20789, .T. ) ;
#28918=ADVANCED_FACE ( 'NONE', ( #31634 ), #18492, .F. ) ;
#28920=ORIENTED_EDGE ( 'NONE', *, *, #6575, .F. ) ;
#28922=CARTESIAN_POINT ( 'NONE',  ( -500.0000000000000000, -115.0000000000000000, -155.0000000000000000 ) ) ;
#28926=DIRECTION ( 'NONE',  ( -0.000000000000000000, 0.000000000000000000, 1.000000000000000000 ) ) ;
#28930=CARTESIAN_POINT ( 'NONE',  ( 19.99999999999998934, -32.99999999999997158, -175.0000000000000000 ) ) ;
#28932=ORIENTED_EDGE ( 'NONE', *, *, #31648, .F. ) ;
#28934=LINE ( 'NONE', #26608, #21166 ) ;
#28936=DIRECTION ( 'NONE',  ( 0.000000000000000000, 1.131431318426415506E-52, 1.000000000000000000 ) ) ;
#28937=ORIENTED_EDGE ( 'NONE', *, *, #5759, .F. ) ;
#28944=DIRECTION ( 'NONE',  ( 0.000000000000000000, 0.000000000000000000, 1.000000000000000000 ) ) ;
#28948=CARTESIAN_POINT ( 'NONE',  ( -418.0000000000000000, -125.0000000000000000, 107.9999999999999858 ) ) ;
#28953=ORIENTED_EDGE ( 'NONE', *, *, #31646, .T. ) ;
#28955=ORIENTED_EDGE ( 'NONE', *, *, #32697, .F. ) ;
#28957=VECTOR ( 'NONE', #34831, 1000.000000000000000 ) ;
#28958=EDGE_CURVE ( 'NONE', #18391, #28976, #17359, .T. ) ;
#28967=ADVANCED_FACE ( 'NONE', ( #24144 ), #17005, .T. ) ;
#28971=AXIS2_PLACEMENT_3D ( 'NONE', #35072, #10852, #16034 ) ;
#28972=DIRECTION ( 'NONE',  ( 0.000000000000000000, 0.000000000000000000, -1.000000000000000000 ) ) ;
#28975=DIRECTION ( 'NONE',  ( 0.000000000000000000, 0.000000000000000000, -1.000000000000000000 ) ) ;
#28976=VERTEX_POINT ( 'NONE', #13481 ) ;
#28977=EDGE_CURVE ( 'NONE', #17491, #5593, #29853, .T. ) ;
#28978=CYLINDRICAL_SURFACE ( 'NONE', #12868, 3.999999999999976019 ) ;
#28979=PLANE ( 'NONE',  #1252 ) ;
#28989=CARTESIAN_POINT ( 'NONE',  ( -355.0000000000000000, 130.9999999999999716, 109.9999999999999858 ) ) ;
#28997=EDGE_CURVE ( 'NONE', #33799, #12627, #23347, .T. ) ;
#28999=CARTESIAN_POINT ( 'NONE',  ( 19.99999999999998934, -137.0000000000000000, 174.9999999999999432 ) ) ;
#29001=DIRECTION ( 'NONE',  ( 0.000000000000000000, 2.309213040847544338E-50, 1.000000000000000000 ) ) ;
#29002=VECTOR ( 'NONE', #9262, 1000.000000000000000 ) ;
#29005=ORIENTED_EDGE ( 'NONE', *, *, #15508, .T. ) ;
#29006=ORIENTED_EDGE ( 'NONE', *, *, #5873, .F. ) ;
#29010=CARTESIAN_POINT ( 'NONE',  ( -12.00000000000001066, -60.99999999999996447, -154.9999999999999716 ) ) ;
#29012=DIRECTION ( 'NONE',  ( 0.000000000000000000, -1.000000000000000000, -5.053935297177146739E-49 ) ) ;
#29014=ORIENTED_EDGE ( 'NONE', *, *, #19110, .T. ) ;
#29020=CARTESIAN_POINT ( 'NONE',  ( -20.00000000000001776, -137.0000000000000000, -194.9999999999999432 ) ) ;
#29023=CIRCLE ( 'NONE', #3461, 7.999999999999979572 ) ;
#29024=CARTESIAN_POINT ( 'NONE',  ( -15.99999999999998579, -112.9999999999999858, -155.0000000000000284 ) ) ;
#29026=EDGE_LOOP ( 'NONE', ( #30757, #17200, #2793, #9254 ) ) ;
#29037=ORIENTED_EDGE ( 'NONE', *, *, #7655, .F. ) ;
#29042=FACE_BOUND ( 'NONE', #6826, .T. ) ;
#29043=EDGE_LOOP ( 'NONE', ( #12118, #7781, #1866, #27154 ) ) ;
#29045=DIRECTION ( 'NONE',  ( 0.000000000000000000, 0.000000000000000000, -1.000000000000000000 ) ) ;
#29051=DIRECTION ( 'NONE',  ( -0.000000000000000000, 5.053935297177146739E-49, 1.000000000000000000 ) ) ;
#29052=ORIENTED_EDGE ( 'NONE', *, *, #6022, .F. ) ;
#29053=VECTOR ( 'NONE', #33916, 1000.000000000000000 ) ;
#29056=VERTEX_POINT ( 'NONE', #33167 ) ;
#29057=DIRECTION ( 'NONE',  ( 0.000000000000000000, 2.465190328815661892E-32, 1.000000000000000000 ) ) ;
#29058=DIRECTION ( 'NONE',  ( -0.000000000000000000, 1.000000000000000000, -0.000000000000000000 ) ) ;
#29066=ORIENTED_EDGE ( 'NONE', *, *, #12755, .T. ) ;
#29068=( GEOMETRIC_REPRESENTATION_CONTEXT ( 3 ) GLOBAL_UNCERTAINTY_ASSIGNED_CONTEXT ( ( #3584 ) ) GLOBAL_UNIT_ASSIGNED_CONTEXT ( ( #34719, #10332, #31681 ) ) REPRESENTATION_CONTEXT ( 'NONE', 'WORKASPACE' ) );
#29070=CARTESIAN_POINT ( 'NONE',  ( -418.0000000000000000, -105.0000000000000142, -69.99999999999998579 ) ) ;
#29073=ORIENTED_EDGE ( 'NONE', *, *, #24986, .F. ) ;
#29074=ADVANCED_FACE ( 'NONE', ( #19667 ), #30512, .T. ) ;
#29076=ORIENTED_EDGE ( 'NONE', *, *, #16893, .T. ) ;
#29078=ORIENTED_EDGE ( 'NONE', *, *, #26819, .T. ) ;
#29083=EDGE_CURVE ( 'NONE', #27224, #24780, #18263, .T. ) ;
#29084=AXIS2_PLACEMENT_3D ( 'NONE', #8897, #17106, #27939 ) ;
#29088=EDGE_CURVE ( 'NONE', #8531, #15586, #1653, .T. ) ;
#29089=ORIENTED_EDGE ( 'NONE', *, *, #3327, .T. ) ;
#29095=CIRCLE ( 'NONE', #33643, 3.999999999999976019 ) ;
#29100=UNCERTAINTY_MEASURE_WITH_UNIT (LENGTH_MEASURE( 1.000000000000000082E-05 ), #16721, 'distance_accuracy_value', 'NONE');
#29102=ORIENTED_EDGE ( 'NONE', *, *, #22595, .T. ) ;
#29104=DIRECTION ( 'NONE',  ( 1.000000000000000000, 0.000000000000000000, 0.000000000000000000 ) ) ;
#29106=DIRECTION ( 'NONE',  ( 0.000000000000000000, -1.000000000000000000, -1.131431318426415506E-52 ) ) ;
#29108=FACE_OUTER_BOUND ( 'NONE', #20474, .T. ) ;
#29112=DIRECTION ( 'NONE',  ( 0.000000000000000000, 0.000000000000000000, 1.000000000000000000 ) ) ;
#29118=AXIS2_PLACEMENT_3D ( 'NONE', #28073, #12726, #15566 ) ;
#29119=AXIS2_PLACEMENT_3D ( 'NONE', #23041, #6468, #14513 ) ;
#29122=DIRECTION ( 'NONE',  ( 0.000000000000000000, 1.310824597558155437E-49, 1.000000000000000000 ) ) ;
#29123=DIRECTION ( 'NONE',  ( 0.000000000000000000, 2.309213040847544338E-50, 1.000000000000000000 ) ) ;
#29130=CARTESIAN_POINT ( 'NONE',  ( 12.00000000000001066, 144.9999999999999716, 155.0000000000000000 ) ) ;
#29131=DIRECTION ( 'NONE',  ( 1.000000000000000000, 0.000000000000000000, 0.000000000000000000 ) ) ;
#29132=CARTESIAN_POINT ( 'NONE',  ( -19.99999999999998934, 144.9999999999999716, 162.9999999999999716 ) ) ;
#29135=ORIENTED_EDGE ( 'NONE', *, *, #19549, .T. ) ;
#29136=EDGE_CURVE ( 'NONE', #173, #34313, #34146, .T. ) ;
#29137=VERTEX_POINT ( 'NONE', #20361 ) ;
#29140=CARTESIAN_POINT ( 'NONE',  ( 12.00000000000003908, -115.0000000000000000, -158.9999999999999716 ) ) ;
#29144=CARTESIAN_POINT ( 'NONE',  ( -19.99999999999998934, 4.559999999999908127, 172.9900000000000091 ) ) ;
#29147=LINE ( 'NONE', #10278, #13461 ) ;
#29154=PLANE ( 'NONE',  #14915 ) ;
#29155=ORIENTED_EDGE ( 'NONE', *, *, #16645, .F. ) ;
#29158=ORIENTED_EDGE ( 'NONE', *, *, #3903, .T. ) ;
#29160=EDGE_CURVE ( 'NONE', #13520, #7154, #25684, .T. ) ;
#29162=EDGE_CURVE ( 'NONE', #22441, #19038, #20871, .T. ) ;
#29164=AXIS2_PLACEMENT_3D ( 'NONE', #31727, #18402, #26567 ) ;
#29165=ORIENTED_EDGE ( 'NONE', *, *, #15825, .T. ) ;
#29167=DIRECTION ( 'NONE',  ( 1.000000000000000000, 0.000000000000000000, 0.000000000000000000 ) ) ;
#29173=VECTOR ( 'NONE', #21503, 1000.000000000000000 ) ;
#29177=CARTESIAN_POINT ( 'NONE',  ( -499.9999999999999432, 112.9999999999999574, -187.0000000000000000 ) ) ;
#29183=ORIENTED_EDGE ( 'NONE', *, *, #28007, .F. ) ;
#29188=ORIENTED_EDGE ( 'NONE', *, *, #11333, .T. ) ;
#29189=ORIENTED_EDGE ( 'NONE', *, *, #7251, .T. ) ;
#29191=VERTEX_POINT ( 'NONE', #12521 ) ;
#29193=CARTESIAN_POINT ( 'NONE',  ( -418.0000000000000000, 105.0000000000000142, 194.9999999999999716 ) ) ;
#29196=CYLINDRICAL_SURFACE ( 'NONE', #24241, 4.000000000000003553 ) ;
#29197=CIRCLE ( 'NONE', #23500, 3.999999999999976019 ) ;
#29202=EDGE_CURVE ( 'NONE', #5838, #18998, #9664, .T. ) ;
#29204=DIRECTION ( 'NONE',  ( 0.000000000000000000, -1.310824597558155437E-49, -1.000000000000000000 ) ) ;
#29206=EDGE_CURVE ( 'NONE', #27900, #18998, #28879, .T. ) ;
#29209=EDGE_CURVE ( 'NONE', #32109, #24914, #26037, .T. ) ;
#29210=CARTESIAN_POINT ( 'NONE',  ( 12.00000000000001066, -134.9999999999999716, 162.9999999999999716 ) ) ;
#29214=AXIS2_PLACEMENT_3D ( 'NONE', #2773, #23955, #12954 ) ;
#29215=ORIENTED_EDGE ( 'NONE', *, *, #16942, .F. ) ;
#29223=ORIENTED_EDGE ( 'NONE', *, *, #18375, .T. ) ;
#29236=DIRECTION ( 'NONE',  ( 0.000000000000000000, 1.000000000000000000, 1.310824597558155437E-49 ) ) ;
#29241=AXIS2_PLACEMENT_3D ( 'NONE', #33011, #27328, #28041 ) ;
#29243=DIRECTION ( 'NONE',  ( 0.000000000000000000, 0.000000000000000000, -1.000000000000000000 ) ) ;
#29253=CYLINDRICAL_SURFACE ( 'NONE', #794, 4.750000000000004441 ) ;
#29260=CARTESIAN_POINT ( 'NONE',  ( -12.00000000000001243, 134.9999999999999432, -154.9999999999999716 ) ) ;
#29261=ORIENTED_EDGE ( 'NONE', *, *, #23739, .T. ) ;
#29265=ORIENTED_EDGE ( 'NONE', *, *, #5677, .F. ) ;
#29270=CARTESIAN_POINT ( 'NONE',  ( -12.00000000000001066, 144.9999999999999716, 155.0000000000000000 ) ) ;
#29271=VECTOR ( 'NONE', #20249, 1000.000000000000000 ) ;
#29273=DIRECTION ( 'NONE',  ( -0.000000000000000000, 1.000000000000000000, 0.000000000000000000 ) ) ;
#29275=ORIENTED_EDGE ( 'NONE', *, *, #26350, .F. ) ;
#29278=DIRECTION ( 'NONE',  ( -3.040835319149746090E-31, -1.000000000000000000, 0.000000000000000000 ) ) ;
#29283=ORIENTED_EDGE ( 'NONE', *, *, #31959, .F. ) ;
#29284=DIRECTION ( 'NONE',  ( -0.000000000000000000, -0.000000000000000000, 1.000000000000000000 ) ) ;
#29287=EDGE_CURVE ( 'NONE', #6968, #20076, #15541, .T. ) ;
#29290=EDGE_CURVE ( 'NONE', #30714, #12639, #23720, .T. ) ;
#29293=FACE_BOUND ( 'NONE', #27227, .T. ) ;
#29294=EDGE_LOOP ( 'NONE', ( #15958, #10207, #7273, #1014 ) ) ;
#29295=VECTOR ( 'NONE', #13041, 1000.000000000000000 ) ;
#29296=VECTOR ( 'NONE', #5795, 1000.000000000000000 ) ;
#29300=CARTESIAN_POINT ( 'NONE',  ( -12.00000000000001066, 144.9999999999999716, 162.9999999999999716 ) ) ;
#29304=EDGE_CURVE ( 'NONE', #34809, #18790, #24053, .T. ) ;
#29307=VECTOR ( 'NONE', #25897, 1000.000000000000000 ) ;
#29312=EDGE_CURVE ( 'NONE', #32956, #10280, #32050, .T. ) ;
#29316=EDGE_LOOP ( 'NONE', ( #32573, #4246, #17928, #32664 ) ) ;
#29318=( NAMED_UNIT ( * ) SI_UNIT ( $, .STERADIAN. ) SOLID_ANGLE_UNIT ( ) );
#29319=AXIS2_PLACEMENT_3D ( 'NONE', #9090, #6403, #24312 ) ;
#29320=CARTESIAN_POINT ( 'NONE',  ( -345.0000000000000000, -125.0000000000000284, 168.9999999999999716 ) ) ;
#29321=DIRECTION ( 'NONE',  ( -1.000000000000000000, 0.000000000000000000, -1.300283923313630633E-47 ) ) ;
#29324=VERTEX_POINT ( 'NONE', #21579 ) ;
#29325=ORIENTED_EDGE ( 'NONE', *, *, #11924, .T. ) ;
#29326=CARTESIAN_POINT ( 'NONE',  ( -445.9999999999999432, -104.9999999999999858, -162.9999999999999716 ) ) ;
#29329=FACE_OUTER_BOUND ( 'NONE', #19375, .T. ) ;
#29331=CARTESIAN_POINT ( 'NONE',  ( -20.00000000000004619, -134.9999999999999716, -162.9999999999999432 ) ) ;
#29332=( LENGTH_UNIT ( ) NAMED_UNIT ( * ) SI_UNIT ( .MILLI., .METRE. ) );
#29333=ORIENTED_EDGE ( 'NONE', *, *, #20887, .T. ) ;
#29335=CARTESIAN_POINT ( 'NONE',  ( 19.99999999999998934, -145.0000000000000000, -162.9999999999999432 ) ) ;
#29337=DIRECTION ( 'NONE',  ( 0.000000000000000000, 1.000000000000000000, -6.123233995736766036E-17 ) ) ;
#29338=ORIENTED_EDGE ( 'NONE', *, *, #23185, .F. ) ;
#29344=AXIS2_PLACEMENT_3D ( 'NONE', #23025, #18051, #6982 ) ;
#29348=DIRECTION ( 'NONE',  ( 0.000000000000000000, 0.000000000000000000, -1.000000000000000000 ) ) ;
#29349=FACE_BOUND ( 'NONE', #3775, .T. ) ;
#29350=CARTESIAN_POINT ( 'NONE',  ( 15.99999999999998579, -145.0000000000000000, -162.9999999999999432 ) ) ;
#29352=ORIENTED_EDGE ( 'NONE', *, *, #19455, .T. ) ;
#29357=DIRECTION ( 'NONE',  ( 1.000000000000000000, 0.000000000000000000, 0.000000000000000000 ) ) ;
#29358=ADVANCED_FACE ( 'NONE', ( #10896 ), #34938, .T. ) ;
#29360=DIRECTION ( 'NONE',  ( 1.000000000000000000, 0.000000000000000000, -1.848892746611746966E-32 ) ) ;
#29362=ORIENTED_EDGE ( 'NONE', *, *, #22508, .F. ) ;
#29369=EDGE_CURVE ( 'NONE', #26816, #34740, #8558, .T. ) ;
#29374=EDGE_CURVE ( 'NONE', #6935, #17160, #13572, .T. ) ;
#29377=ORIENTED_EDGE ( 'NONE', *, *, #29780, .T. ) ;
#29378=LINE ( 'NONE', #32216, #24316 ) ;
#29379=DIRECTION ( 'NONE',  ( 0.000000000000000000, -1.000000000000000000, 0.000000000000000000 ) ) ;
#29380=ORIENTED_EDGE ( 'NONE', *, *, #8435, .F. ) ;
#29382=CARTESIAN_POINT ( 'NONE',  ( 11.99999999999999645, 134.9999999999998863, 162.9999999999999716 ) ) ;
#29387=EDGE_CURVE ( 'NONE', #17403, #19022, #18915, .T. ) ;
#29390=DIRECTION ( 'NONE',  ( 0.000000000000000000, 0.000000000000000000, -1.000000000000000000 ) ) ;
#29391=CIRCLE ( 'NONE', #14048, 3.999999999999976019 ) ;
#29392=CIRCLE ( 'NONE', #969, 7.999999999999979572 ) ;
#29395=EDGE_LOOP ( 'NONE', ( #29555, #5202, #28953, #1983 ) ) ;
#29409=EDGE_LOOP ( 'NONE', ( #23351, #178, #16138, #3387, #18179 ) ) ;
#29411=DIRECTION ( 'NONE',  ( 1.000000000000000000, 0.000000000000000000, 0.000000000000000000 ) ) ;
#29413=CARTESIAN_POINT ( 'NONE',  ( -355.0000000000000000, 134.9999999999999716, 126.0000000000000000 ) ) ;
#29418=CIRCLE ( 'NONE', #32803, 3.999999999999976019 ) ;
#29419=CIRCLE ( 'NONE', #19748, 3.999999999999976019 ) ;
#29422=EDGE_CURVE ( 'NONE', #31845, #4999, #30467, .T. ) ;
#29425=CARTESIAN_POINT ( 'NONE',  ( -19.99999999999998934, -134.9999999999999716, 187.0000000000000000 ) ) ;
#29426=CIRCLE ( 'NONE', #30546, 4.750000000000004441 ) ;
#29429=DIRECTION ( 'NONE',  ( 0.000000000000000000, 0.000000000000000000, -1.000000000000000000 ) ) ;
#29432=CARTESIAN_POINT ( 'NONE',  ( -15.99999999999998579, 144.9999999999999716, 162.9999999999999716 ) ) ;
#29433=LINE ( 'NONE', #20548, #33905 ) ;
#29434=VECTOR ( 'NONE', #32449, 1000.000000000000000 ) ;
#29442=ORIENTED_EDGE ( 'NONE', *, *, #6730, .F. ) ;
#29445=ORIENTED_EDGE ( 'NONE', *, *, #22548, .T. ) ;
#29446=DIRECTION ( 'NONE',  ( 0.000000000000000000, 1.131431318426415506E-52, 1.000000000000000000 ) ) ;
#29447=EDGE_CURVE ( 'NONE', #35, #32367, #21090, .T. ) ;
#29452=CYLINDRICAL_SURFACE ( 'NONE', #29618, 4.000000000000003553 ) ;
#29454=ORIENTED_EDGE ( 'NONE', *, *, #29290, .T. ) ;
#29455=CARTESIAN_POINT ( 'NONE',  ( -442.0000000000000000, -105.0000000000000142, 155.0000000000000000 ) ) ;
#29460=EDGE_LOOP ( 'NONE', ( #20469, #9122, #19093, #2981, #4464, #3749, #16031, #15468 ) ) ;
#29463=DIRECTION ( 'NONE',  ( -1.000000000000000000, -3.040835319149746090E-31, -1.232595164407830946E-32 ) ) ;
#29465=PLANE ( 'NONE',  #387 ) ;
#29466=CARTESIAN_POINT ( 'NONE',  ( -410.0000000000000568, 105.0000000000000142, -101.9999999999999858 ) ) ;
#29470=VERTEX_POINT ( 'NONE', #27965 ) ;
#29472=VECTOR ( 'NONE', #33256, 1000.000000000000000 ) ;
#29473=CARTESIAN_POINT ( 'NONE',  ( -12.00000000000001066, 144.9999999999999147, 162.9999999999999716 ) ) ;
#29474=ORIENTED_EDGE ( 'NONE', *, *, #11577, .F. ) ;
#29478=AXIS2_PLACEMENT_3D ( 'NONE', #33438, #17453, #30769 ) ;
#29479=ORIENTED_EDGE ( 'NONE', *, *, #8435, .T. ) ;
#29480=CARTESIAN_POINT ( 'NONE',  ( 11.99999999999999645, 124.9999999999999716, 162.9999999999999716 ) ) ;
#29483=VECTOR ( 'NONE', #29901, 1000.000000000000000 ) ;
#29487=ORIENTED_EDGE ( 'NONE', *, *, #10768, .F. ) ;
#29488=DIRECTION ( 'NONE',  ( 5.546364386991661285E-52, 0.000000000000000000, 1.000000000000000000 ) ) ;
#29489=VERTEX_POINT ( 'NONE', #19443 ) ;
#29490=CARTESIAN_POINT ( 'NONE',  ( 19.99999999999996092, -134.9999999999999716, -162.9999999999999432 ) ) ;
#29491=ADVANCED_FACE ( 'NONE', ( #3571 ), #27611, .F. ) ;
#29493=AXIS2_PLACEMENT_3D ( 'NONE', #23442, #1726, #4213 ) ;
#29494=ADVANCED_FACE ( 'NONE', ( #27786 ), #3049, .T. ) ;
#29497=ORIENTED_EDGE ( 'NONE', *, *, #18980, .T. ) ;
#29498=ORIENTED_EDGE ( 'NONE', *, *, #34474, .F. ) ;
#29500=VERTEX_POINT ( 'NONE', #19797 ) ;
#29503=CARTESIAN_POINT ( 'NONE',  ( -499.9999999999999432, 104.9999999999999858, 162.9999999999999716 ) ) ;
#29505=CIRCLE ( 'NONE', #28909, 7.999999999999952038 ) ;
#29506=DIRECTION ( 'NONE',  ( -1.000000000000000000, 0.000000000000000000, -1.292961597001347186E-16 ) ) ;
#29507=DIRECTION ( 'NONE',  ( 1.232595164407830946E-32, 7.496237820289040735E-63, -1.000000000000000000 ) ) ;
#29510=ORIENTED_EDGE ( 'NONE', *, *, #33501, .F. ) ;
#29512=EDGE_CURVE ( 'NONE', #12400, #19207, #30644, .T. ) ;
#29513=FACE_OUTER_BOUND ( 'NONE', #26594, .T. ) ;
#29515=VERTEX_POINT ( 'NONE', #25105 ) ;
#29520=CARTESIAN_POINT ( 'NONE',  ( 11.99999999999999645, 124.9999999999999716, 162.9999999999999716 ) ) ;
#29525=ORIENTED_EDGE ( 'NONE', *, *, #23432, .F. ) ;
#29527=ORIENTED_EDGE ( 'NONE', *, *, #32103, .F. ) ;
#29530=ORIENTED_EDGE ( 'NONE', *, *, #33939, .T. ) ;
#29532=EDGE_CURVE ( 'NONE', #9246, #10430, #6232, .T. ) ;
#29533=DIRECTION ( 'NONE',  ( 0.000000000000000000, 0.000000000000000000, 1.000000000000000000 ) ) ;
#29534=VECTOR ( 'NONE', #17534, 1000.000000000000000 ) ;
#29537=ORIENTED_EDGE ( 'NONE', *, *, #27031, .F. ) ;
#29541=DIRECTION ( 'NONE',  ( -3.469446951953832974E-18, -1.000000000000000000, -7.888609052210116302E-31 ) ) ;
#29542=CARTESIAN_POINT ( 'NONE',  ( -499.9999999999999432, 136.9999999999999432, 162.9999999999999716 ) ) ;
#29552=VECTOR ( 'NONE', #23210, 1000.000000000000000 ) ;
#29553=LINE ( 'NONE', #15870, #18114 ) ;
#29554=DIRECTION ( 'NONE',  ( -1.000000000000000000, 0.000000000000000000, -1.300283923313630633E-47 ) ) ;
#29555=ORIENTED_EDGE ( 'NONE', *, *, #31273, .F. ) ;
#29557=LINE ( 'NONE', #22249, #9766 ) ;
#29559=CARTESIAN_POINT ( 'NONE',  ( -349.0000000000000000, -125.0000000000000284, 130.0000000000000000 ) ) ;
#29560=CARTESIAN_POINT ( 'NONE',  ( -442.0000000000000000, -125.0000000000000000, 100.0000000000000000 ) ) ;
#29563=CARTESIAN_POINT ( 'NONE',  ( -430.0000000000000000, 130.9999999999999716, 126.0000000000000000 ) ) ;
#29572=VECTOR ( 'NONE', #26544, 1000.000000000000000 ) ;
#29581=EDGE_CURVE ( 'NONE', #8689, #26511, #22984, .T. ) ;
#29583=DIRECTION ( 'NONE',  ( 1.000000000000000000, 3.040835319149746528E-31, 1.232595164407830946E-32 ) ) ;
#29587=LINE ( 'NONE', #5182, #30197 ) ;
#29589=CARTESIAN_POINT ( 'NONE',  ( -500.0000000000000000, -105.0000000000000142, 187.0000000000000000 ) ) ;
#29591=DIRECTION ( 'NONE',  ( 0.000000000000000000, -1.000000000000000000, 0.000000000000000000 ) ) ;
#29594=ADVANCED_FACE ( 'NONE', ( #9277, #1612 ), #31170, .T. ) ;
#29601=CARTESIAN_POINT ( 'NONE',  ( -361.0000000000000000, 134.9999999999999716, 112.0000000000000000 ) ) ;
#29602=DIRECTION ( 'NONE',  ( -1.232595164407830946E-32, 0.000000000000000000, -1.000000000000000000 ) ) ;
#29606=ORIENTED_EDGE ( 'NONE', *, *, #32256, .T. ) ;
#29608=CARTESIAN_POINT ( 'NONE',  ( -12.00000000000001066, -112.9999999999999858, 155.0000000000000000 ) ) ;
#29609=VECTOR ( 'NONE', #9029, 1000.000000000000000 ) ;
#29612=ORIENTED_EDGE ( 'NONE', *, *, #33754, .T. ) ;
#29614=ORIENTED_EDGE ( 'NONE', *, *, #18930, .F. ) ;
#29617=CARTESIAN_POINT ( 'NONE',  ( -361.0000000000000000, -125.0000000000000284, 168.9999999999999716 ) ) ;
#29618=AXIS2_PLACEMENT_3D ( 'NONE', #32628, #10932, #29620 ) ;
#29619=CARTESIAN_POINT ( 'NONE',  ( -12.00000000000001066, -28.99999999999999645, -175.0000000000000000 ) ) ;
#29620=DIRECTION ( 'NONE',  ( 0.000000000000000000, 0.000000000000000000, 1.000000000000000000 ) ) ;
#29621=VERTEX_POINT ( 'NONE', #30816 ) ;
#29623=DIRECTION ( 'NONE',  ( 0.000000000000000000, 1.000000000000000000, 5.145227585319922065E-49 ) ) ;
#29632=AXIS2_PLACEMENT_3D ( 'NONE', #5673, #10518, #30083 ) ;
#29638=EDGE_LOOP ( 'NONE', ( #14641, #13210, #10996, #11493 ) ) ;
#29640=ORIENTED_EDGE ( 'NONE', *, *, #18289, .T. ) ;
#29641=LINE ( 'NONE', #15787, #14869 ) ;
#29646=VERTEX_POINT ( 'NONE', #7462 ) ;
#29648=( NAMED_UNIT ( * ) PLANE_ANGLE_UNIT ( ) SI_UNIT ( $, .RADIAN. ) );
#29650=CARTESIAN_POINT ( 'NONE',  ( -418.0000000000000000, -125.0000000000000000, 194.9999999999999716 ) ) ;
#29652=AXIS2_PLACEMENT_3D ( 'NONE', #28682, #20163, #17678 ) ;
#29653=AXIS2_PLACEMENT_3D ( 'NONE', #8170, #11382, #22238 ) ;
#29655=AXIS2_PLACEMENT_3D ( 'NONE', #4400, #26296, #21317 ) ;
#29657=DIRECTION ( 'NONE',  ( 0.000000000000000000, 1.000000000000000000, 2.309213040847544338E-50 ) ) ;
#29658=CARTESIAN_POINT ( 'NONE',  ( -499.9999999999999432, 108.9999999999999858, 187.0000000000000000 ) ) ;
#29667=EDGE_LOOP ( 'NONE', ( #30337, #28405, #21421, #20082 ) ) ;
#29669=DIRECTION ( 'NONE',  ( -0.000000000000000000, -1.000000000000000000, -0.000000000000000000 ) ) ;
#29674=LINE ( 'NONE', #16165, #34516 ) ;
#29676=VERTEX_POINT ( 'NONE', #2138 ) ;
#29678=DIRECTION ( 'NONE',  ( -3.469446951953832974E-18, -1.000000000000000000, -7.888609052210116302E-31 ) ) ;
#29680=CARTESIAN_POINT ( 'NONE',  ( -20.00000000000007461, -113.0000000000000000, -159.0000000000000000 ) ) ;
#29681=ORIENTED_EDGE ( 'NONE', *, *, #17797, .T. ) ;
#29686=DIRECTION ( 'NONE',  ( -0.000000000000000000, 1.000000000000000000, -0.000000000000000000 ) ) ;
#29689=EDGE_CURVE ( 'NONE', #32490, #1130, #34356, .T. ) ;
#29690=ORIENTED_EDGE ( 'NONE', *, *, #3155, .F. ) ;
#29692=DIRECTION ( 'NONE',  ( 0.000000000000000000, 1.000000000000000000, 5.145227585319922065E-49 ) ) ;
#29694=DIRECTION ( 'NONE',  ( 1.000000000000000000, 0.000000000000000000, 0.000000000000000000 ) ) ;
#29698=DIRECTION ( 'NONE',  ( -1.000000000000000000, 0.000000000000000000, -0.000000000000000000 ) ) ;
#29703=VECTOR ( 'NONE', #24724, 1000.000000000000000 ) ;
#29707=VECTOR ( 'NONE', #18411, 1000.000000000000000 ) ;
#29708=VERTEX_POINT ( 'NONE', #34533 ) ;
#29709=VECTOR ( 'NONE', #24109, 1000.000000000000000 ) ;
#29710=ORIENTED_EDGE ( 'NONE', *, *, #27569, .F. ) ;
#29711=CARTESIAN_POINT ( 'NONE',  ( 19.99999999999998934, 144.9999999999999716, -186.9999999999999716 ) ) ;
#29712=FACE_OUTER_BOUND ( 'NONE', #21727, .T. ) ;
#29714=ORIENTED_EDGE ( 'NONE', *, *, #15853, .F. ) ;
#29716=CARTESIAN_POINT ( 'NONE',  ( -418.0000000000000000, -125.0000000000000000, 190.9999999999999716 ) ) ;
#29718=CARTESIAN_POINT ( 'NONE',  ( -361.0000000000000000, -135.0000000000000000, 128.0000000000000000 ) ) ;
#29723=LINE ( 'NONE', #16220, #8633 ) ;
#29725=DIRECTION ( 'NONE',  ( 0.000000000000000000, 1.000000000000000000, 0.000000000000000000 ) ) ;
#29728=LINE ( 'NONE', #16224, #17837 ) ;
#29731=AXIS2_PLACEMENT_3D ( 'NONE', #32514, #27352, #8137 ) ;
#29733=AXIS2_PLACEMENT_3D ( 'NONE', #17711, #20026, #28022 ) ;
#29735=CYLINDRICAL_SURFACE ( 'NONE', #20744, 4.750000000000004441 ) ;
#29737=EDGE_CURVE ( 'NONE', #18467, #30469, #13184, .T. ) ;
#29739=EDGE_CURVE ( 'NONE', #11787, #13964, #9177, .T. ) ;
#29740=DIRECTION ( 'NONE',  ( 0.000000000000000000, 0.000000000000000000, -1.000000000000000000 ) ) ;
#29744=EDGE_CURVE ( 'NONE', #11473, #6935, #80, .T. ) ;
#29745=VECTOR ( 'NONE', #23888, 1000.000000000000000 ) ;
#29746=LINE ( 'NONE', #14087, #22179 ) ;
#29749=CARTESIAN_POINT ( 'NONE',  ( -449.9999999999999432, 105.0000000000000142, 132.0000000000000000 ) ) ;
#29753=AXIS2_PLACEMENT_3D ( 'NONE', #11138, #26970, #13981 ) ;
#29756=FACE_OUTER_BOUND ( 'NONE', #3879, .T. ) ;
#29758=FACE_OUTER_BOUND ( 'NONE', #23144, .T. ) ;
#29759=DIRECTION ( 'NONE',  ( 1.000000000000000000, 0.000000000000000000, 0.000000000000000000 ) ) ;
#29760=DIRECTION ( 'NONE',  ( -0.000000000000000000, 1.000000000000000000, -0.000000000000000000 ) ) ;
#29762=PLANE ( 'NONE',  #12939 ) ;
#29763=LINE ( 'NONE', #402, #14578 ) ;
#29765=CARTESIAN_POINT ( 'NONE',  ( -410.0000000000000568, -104.9999999999999716, -187.0000000000000000 ) ) ;
#29771=CARTESIAN_POINT ( 'NONE',  ( 11.99999999999999645, 124.9999999999999716, 159.0000000000000000 ) ) ;
#29774=LINE ( 'NONE', #5384, #15514 ) ;
#29776=EDGE_CURVE ( 'NONE', #591, #16412, #18355, .T. ) ;
#29779=VERTEX_POINT ( 'NONE', #24013 ) ;
#29780=EDGE_CURVE ( 'NONE', #8977, #34561, #32026, .T. ) ;
#29783=FACE_OUTER_BOUND ( 'NONE', #33903, .T. ) ;
#29785=EDGE_LOOP ( 'NONE', ( #15686, #19269, #34919, #13453, #17342 ) ) ;
#29786=ORIENTED_EDGE ( 'NONE', *, *, #32576, .F. ) ;
#29789=VERTEX_POINT ( 'NONE', #29010 ) ;
#29790=CARTESIAN_POINT ( 'NONE',  ( -500.0000000000000000, -105.0000000000000142, 162.9999999999999716 ) ) ;
#29792=CIRCLE ( 'NONE', #13871, 2.000000000000001776 ) ;
#29794=FACE_OUTER_BOUND ( 'NONE', #25718, .T. ) ;
#29798=( NAMED_UNIT ( * ) SI_UNIT ( $, .STERADIAN. ) SOLID_ANGLE_UNIT ( ) );
#29799=AXIS2_PLACEMENT_3D ( 'NONE', #23158, #3913, #28661 ) ;
#29800=EDGE_CURVE ( 'NONE', #25155, #33086, #4968, .T. ) ;
#29810=AXIS2_PLACEMENT_3D ( 'NONE', #8157, #26853, #18693 ) ;
#29811=FACE_OUTER_BOUND ( 'NONE', #958, .T. ) ;
#29812=EDGE_CURVE ( 'NONE', #5593, #1001, #30207, .T. ) ;
#29814=DIRECTION ( 'NONE',  ( 1.000000000000000000, 0.000000000000000000, 0.000000000000000000 ) ) ;
#29820=CARTESIAN_POINT ( 'NONE',  ( -12.00000000000003908, -145.0000000000000000, -162.9999999999999432 ) ) ;
#29822=AXIS2_PLACEMENT_3D ( 'NONE', #31583, #7186, #28914 ) ;
#29826=CARTESIAN_POINT ( 'NONE',  ( 11.99999999999999645, -55.00000000000000711, -162.9999999999999432 ) ) ;
#29827=DIRECTION ( 'NONE',  ( 0.000000000000000000, 1.131431318426415506E-52, 1.000000000000000000 ) ) ;
#29838=DIRECTION ( 'NONE',  ( 0.000000000000000000, -1.131431318426415506E-52, -1.000000000000000000 ) ) ;
#29840=FACE_OUTER_BOUND ( 'NONE', #10286, .T. ) ;
#29842=EDGE_LOOP ( 'NONE', ( #34342, #11556 ) ) ;
#29844=LINE ( 'NONE', #21824, #5973 ) ;
#29850=EDGE_CURVE ( 'NONE', #35062, #17587, #13530, .T. ) ;
#29851=VECTOR ( 'NONE', #1086, 1000.000000000000000 ) ;
#29853=LINE ( 'NONE', #21657, #6258 ) ;
#29859=DIRECTION ( 'NONE',  ( 1.000000000000000000, 0.000000000000000000, 0.000000000000000000 ) ) ;
#29860=FACE_OUTER_BOUND ( 'NONE', #19752, .T. ) ;
#29866=CARTESIAN_POINT ( 'NONE',  ( -499.9999999999999432, 136.9999999999999432, 187.0000000000000000 ) ) ;
#29868=CARTESIAN_POINT ( 'NONE',  ( 15.99999999999998579, 124.9999999999999716, 187.0000000000000000 ) ) ;
#29872=CARTESIAN_POINT ( 'NONE',  ( -12.00000000000001066, 134.9999999999999432, -186.9999999999999716 ) ) ;
#29876=CIRCLE ( 'NONE', #11137, 7.999999999999979572 ) ;
#29880=ADVANCED_FACE ( 'NONE', ( #27397 ), #22415, .T. ) ;
#29882=VECTOR ( 'NONE', #28012, 1000.000000000000000 ) ;
#29883=CARTESIAN_POINT ( 'NONE',  ( -430.0000000000000000, -119.0000000000000000, 113.9999999999999858 ) ) ;
#29884=CARTESIAN_POINT ( 'NONE',  ( 11.99999999999999645, -141.0000000000000000, -155.0000000000000284 ) ) ;
#29887=ORIENTED_EDGE ( 'NONE', *, *, #33632, .F. ) ;
#29893=EDGE_CURVE ( 'NONE', #6460, #12542, #32907, .T. ) ;
#29896=DIRECTION ( 'NONE',  ( 0.000000000000000000, 0.000000000000000000, 1.000000000000000000 ) ) ;
#29897=ORIENTED_EDGE ( 'NONE', *, *, #31697, .F. ) ;
#29898=VERTEX_POINT ( 'NONE', #33267 ) ;
#29899=DIRECTION ( 'NONE',  ( 0.000000000000000000, -1.000000000000000000, 3.374343856708137958E-53 ) ) ;
#29901=DIRECTION ( 'NONE',  ( 0.000000000000000000, -7.888609052210118054E-31, -1.000000000000000000 ) ) ;
#29915=LINE ( 'NONE', #2845, #11441 ) ;
#29916=CARTESIAN_POINT ( 'NONE',  ( -20.00000000000007461, -145.0000000000000000, -187.0000000000000000 ) ) ;
#29918=VECTOR ( 'NONE', #7040, 1000.000000000000000 ) ;
#29919=ORIENTED_EDGE ( 'NONE', *, *, #15022, .T. ) ;
#29922=VERTEX_POINT ( 'NONE', #33085 ) ;
#29928=ORIENTED_EDGE ( 'NONE', *, *, #10411, .T. ) ;
#29930=LINE ( 'NONE', #8385, #3938 ) ;
#29932=EDGE_CURVE ( 'NONE', #2181, #17362, #8702, .T. ) ;
#29937=CARTESIAN_POINT ( 'NONE',  ( -365.0000000000000000, 118.9999999999999716, 113.9999999999999858 ) ) ;
#29943=VERTEX_POINT ( 'NONE', #24534 ) ;
#29945=DIRECTION ( 'NONE',  ( 0.000000000000000000, -6.123233995736766036E-17, -1.000000000000000000 ) ) ;
#29948=DIRECTION ( 'NONE',  ( 1.000000000000000000, 0.000000000000000000, 0.000000000000000000 ) ) ;
#29949=EDGE_CURVE ( 'NONE', #7621, #11365, #25663, .T. ) ;
#29951=LINE ( 'NONE', #5543, #11061 ) ;
#29956=CARTESIAN_POINT ( 'NONE',  ( -449.9999999999999432, 105.0000000000000142, -175.0000000000000000 ) ) ;
#29958=FACE_BOUND ( 'NONE', #1709, .T. ) ;
#29959=ORIENTED_EDGE ( 'NONE', *, *, #7333, .F. ) ;
#29960=( NAMED_UNIT ( * ) PLANE_ANGLE_UNIT ( ) SI_UNIT ( $, .RADIAN. ) );
#29961=ORIENTED_EDGE ( 'NONE', *, *, #18428, .F. ) ;
#29969=AXIS2_PLACEMENT_3D ( 'NONE', #23549, #26391, #5019 ) ;
#29970=DIRECTION ( 'NONE',  ( 0.000000000000000000, -1.000000000000000000, -2.465190328815662439E-32 ) ) ;
#29971=CYLINDRICAL_SURFACE ( 'NONE', #18282, 7.999999999999979572 ) ;
#29975=( NAMED_UNIT ( * ) PLANE_ANGLE_UNIT ( ) SI_UNIT ( $, .RADIAN. ) );
#29977=ADVANCED_FACE ( 'NONE', ( #3187 ), #531, .T. ) ;
#29980=EDGE_LOOP ( 'NONE', ( #60, #711, #6101, #6621 ) ) ;
#29983=ADVANCED_FACE ( 'NONE', ( #19579 ), #16393, .T. ) ;
#29984=EDGE_CURVE ( 'NONE', #4470, #19925, #2937, .T. ) ;
#29990=CARTESIAN_POINT ( 'NONE',  ( -20.00000000000007461, 112.9999999999999574, -162.9999999999999716 ) ) ;
#29991=VERTEX_POINT ( 'NONE', #23296 ) ;
#29992=VECTOR ( 'NONE', #6194, 1000.000000000000000 ) ;
#29995=FACE_OUTER_BOUND ( 'NONE', #17451, .T. ) ;
#29998=EDGE_CURVE ( 'NONE', #22841, #21039, #17275, .T. ) ;
#29999=AXIS2_PLACEMENT_3D ( 'NONE', #33127, #32946, #30470 ) ;
#30004=VERTEX_POINT ( 'NONE', #31470 ) ;
#30007=ORIENTED_EDGE ( 'NONE', *, *, #21571, .T. ) ;
#30012=LINE ( 'NONE', #33379, #27502 ) ;
#30013=LINE ( 'NONE', #5605, #15894 ) ;
#30015=CARTESIAN_POINT ( 'NONE',  ( -12.00000000000001066, 108.9999999999999858, -175.0000000000000284 ) ) ;
#30017=ORIENTED_EDGE ( 'NONE', *, *, #761, .F. ) ;
#30023=AXIS2_PLACEMENT_3D ( 'NONE', #10839, #30057, #2286 ) ;
#30031=CARTESIAN_POINT ( 'NONE',  ( -500.0000000000000000, -113.0000000000000000, 159.0000000000000000 ) ) ;
#30032=LINE ( 'NONE', #19015, #26804 ) ;
#30038=ORIENTED_EDGE ( 'NONE', *, *, #33628, .F. ) ;
#30043=DIRECTION ( 'NONE',  ( 0.000000000000000000, -1.310824597558155437E-49, -1.000000000000000000 ) ) ;
#30044=LINE ( 'NONE', #7634, #31005 ) ;
#30050=EDGE_LOOP ( 'NONE', ( #849, #3423, #11912, #28535, #32357, #34287, #33405, #31924 ) ) ;
#30052=LINE ( 'NONE', #32529, #14447 ) ;
#30055=ADVANCED_FACE ( 'NONE', ( #29513 ), #28979, .F. ) ;
#30056=VECTOR ( 'NONE', #27175, 1000.000000000000000 ) ;
#30057=DIRECTION ( 'NONE',  ( 1.000000000000000000, 0.000000000000000000, 0.000000000000000000 ) ) ;
#30058=ADVANCED_FACE ( 'NONE', ( #18153 ), #20970, .F. ) ;
#30064=EDGE_LOOP ( 'NONE', ( #8071, #7859, #16302, #13332 ) ) ;
#30066=CARTESIAN_POINT ( 'NONE',  ( -365.0000000000000000, -135.0000000000000000, 126.0000000000000000 ) ) ;
#30068=CYLINDRICAL_SURFACE ( 'NONE', #17356, 4.000000000000003553 ) ;
#30069=VECTOR ( 'NONE', #9373, 1000.000000000000000 ) ;
#30072=CYLINDRICAL_SURFACE ( 'NONE', #30515, 7.999999999999979572 ) ;
#30075=CARTESIAN_POINT ( 'NONE',  ( 11.99999999999999645, -115.0000000000000000, 162.9999999999999716 ) ) ;
#30076=VERTEX_POINT ( 'NONE', #26304 ) ;
#30077=STYLED_ITEM('',(#35254),#10767);
#30079=LINE ( 'NONE', #21885, #25960 ) ;
#30081=VERTEX_POINT ( 'NONE', #18668 ) ;
#30083=DIRECTION ( 'NONE',  ( 0.000000000000000000, 0.000000000000000000, -1.000000000000000000 ) ) ;
#30086=LINE ( 'NONE', #29560, #4864 ) ;
#30089=EDGE_CURVE ( 'NONE', #108, #2320, #26830, .T. ) ;
#30090=EDGE_CURVE ( 'NONE', #19038, #14635, #1915, .T. ) ;
#30091=ORIENTED_EDGE ( 'NONE', *, *, #28074, .F. ) ;
#30099=ORIENTED_EDGE ( 'NONE', *, *, #24145, .F. ) ;
#30102=CARTESIAN_POINT ( 'NONE',  ( -12.00000000000001066, 144.9999999999999716, -154.9999999999999716 ) ) ;
#30103=PLANE ( 'NONE',  #11870 ) ;
#30109=DIRECTION ( 'NONE',  ( 1.000000000000000000, -0.000000000000000000, -0.000000000000000000 ) ) ;
#30111=ORIENTED_EDGE ( 'NONE', *, *, #4940, .F. ) ;
#30113=CARTESIAN_POINT ( 'NONE',  ( -499.9999999999999432, 108.9999999999999858, -187.0000000000000000 ) ) ;
#30115=AXIS2_PLACEMENT_3D ( 'NONE', #7284, #1611, #26338 ) ;
#30117=CARTESIAN_POINT ( 'NONE',  ( -445.9999999999999432, 105.0000000000000142, 162.9999999999999716 ) ) ;
#30121=DIRECTION ( 'NONE',  ( 0.000000000000000000, 0.000000000000000000, 1.000000000000000000 ) ) ;
#30122=ORIENTED_EDGE ( 'NONE', *, *, #3155, .T. ) ;
#30123=LINE ( 'NONE', #24419, #30396 ) ;
#30125=CARTESIAN_POINT ( 'NONE',  ( -19.99999999999998934, -56.99999999999997868, -175.0000000000000000 ) ) ;
#30133=FACE_OUTER_BOUND ( 'NONE', #21372, .T. ) ;
#30134=EDGE_LOOP ( 'NONE', ( #26586, #26770, #16837, #25860 ) ) ;
#30135=VERTEX_POINT ( 'NONE', #15993 ) ;
#30138=CYLINDRICAL_SURFACE ( 'NONE', #7259, 3.999999999999982681 ) ;
#30142=CARTESIAN_POINT ( 'NONE',  ( 19.99999999999996092, -134.9999999999999716, 162.9999999999999716 ) ) ;
#30143=CARTESIAN_POINT ( 'NONE',  ( -365.0000000000000000, 134.9999999999999716, 113.9999999999999858 ) ) ;
#30146=EDGE_LOOP ( 'NONE', ( #15982, #24970, #18506, #16218, #33186 ) ) ;
#30148=CARTESIAN_POINT ( 'NONE',  ( -12.00000000000001066, 124.9999999999999716, 155.0000000000000000 ) ) ;
#30149=CARTESIAN_POINT ( 'NONE',  ( -500.0000000000000000, -109.0000000000000142, 187.0000000000000000 ) ) ;
#30150=EDGE_LOOP ( 'NONE', ( #12345, #2638, #31557, #34458 ) ) ;
#30153=CARTESIAN_POINT ( 'NONE',  ( 19.99999999999998934, -137.0000000000000000, 174.9999999999999432 ) ) ;
#30154=LINE ( 'NONE', #21625, #25716 ) ;
#30158=DIRECTION ( 'NONE',  ( 0.000000000000000000, 0.000000000000000000, 1.000000000000000000 ) ) ;
#30159=VERTEX_POINT ( 'NONE', #32340 ) ;
#30160=DIRECTION ( 'NONE',  ( 1.000000000000000000, 0.000000000000000000, 0.000000000000000000 ) ) ;
#30164=ORIENTED_EDGE ( 'NONE', *, *, #19369, .F. ) ;
#30166=DIRECTION ( 'NONE',  ( 0.000000000000000000, 0.000000000000000000, 1.000000000000000000 ) ) ;
#30167=AXIS2_PLACEMENT_3D ( 'NONE', #8606, #26953, #24803 ) ;
#30170=VERTEX_POINT ( 'NONE', #1745 ) ;
#30171=VECTOR ( 'NONE', #31416, 1000.000000000000000 ) ;
#30172=EDGE_CURVE ( 'NONE', #22441, #34152, #30032, .T. ) ;
#30173=ADVANCED_FACE ( 'NONE', ( #29860 ), #13487, .T. ) ;
#30177=ORIENTED_EDGE ( 'NONE', *, *, #29739, .T. ) ;
#30178=VERTEX_POINT ( 'NONE', #32509 ) ;
#30180=EDGE_CURVE ( 'NONE', #6409, #30837, #16026, .T. ) ;
#30183=VECTOR ( 'NONE', #22850, 1000.000000000000000 ) ;
#30184=DIRECTION ( 'NONE',  ( 0.000000000000000000, 1.000000000000000000, 5.053935297177146739E-49 ) ) ;
#30186=EDGE_LOOP ( 'NONE', ( #18900, #18333, #7522, #30672, #16557, #7000, #16990, #34891 ) ) ;
#30188=FACE_OUTER_BOUND ( 'NONE', #17565, .T. ) ;
#30189=DIRECTION ( 'NONE',  ( 1.000000000000000000, 0.000000000000000000, 5.546364386991661285E-52 ) ) ;
#30195=CYLINDRICAL_SURFACE ( 'NONE', #5036, 7.999999999999979572 ) ;
#30197=VECTOR ( 'NONE', #29760, 1000.000000000000000 ) ;
#30198=CARTESIAN_POINT ( 'NONE',  ( -500.0000000000000000, -137.0000000000000000, 159.0000000000000000 ) ) ;
#30202=ORIENTED_EDGE ( 'NONE', *, *, #6531, .F. ) ;
#30207=CIRCLE ( 'NONE', #4596, 2.000000000000001776 ) ;
#30209=VECTOR ( 'NONE', #2932, 1000.000000000000000 ) ;
#30210=CARTESIAN_POINT ( 'NONE',  ( -442.0000000000000000, -105.0000000000000142, 155.0000000000000000 ) ) ;
#30212=DIRECTION ( 'NONE',  ( -0.000000000000000000, 1.000000000000000000, -0.000000000000000000 ) ) ;
#30215=EDGE_CURVE ( 'NONE', #27224, #27344, #5796, .T. ) ;
#30220=DIRECTION ( 'NONE',  ( -1.000000000000000000, 0.000000000000000000, 0.000000000000000000 ) ) ;
#30223=FACE_OUTER_BOUND ( 'NONE', #12128, .T. ) ;
#30225=ORIENTED_EDGE ( 'NONE', *, *, #21523, .F. ) ;
#30226=ORIENTED_EDGE ( 'NONE', *, *, #29850, .T. ) ;
#30228=CARTESIAN_POINT ( 'NONE',  ( -442.0000000000000000, 105.0000000000000142, -109.9999999999999574 ) ) ;
#30231=AXIS2_PLACEMENT_3D ( 'NONE', #19942, #16408, #27237 ) ;
#30234=VERTEX_POINT ( 'NONE', #32692 ) ;
#30236=CARTESIAN_POINT ( 'NONE',  ( -449.9999999999999432, -137.0000000000000000, 155.0000000000000000 ) ) ;
#30240=ADVANCED_FACE ( 'NONE', ( #27705 ), #27347, .T. ) ;
#30242=DIRECTION ( 'NONE',  ( 0.000000000000000000, 1.000000000000000000, 1.224646799147353207E-16 ) ) ;
#30247=LINE ( 'NONE', #11037, #29703 ) ;
#30248=EDGE_LOOP ( 'NONE', ( #10387, #28376, #13272, #3382 ) ) ;
#30252=DIRECTION ( 'NONE',  ( 0.000000000000000000, -1.000000000000000000, -2.465190328815662439E-32 ) ) ;
#30253=FACE_OUTER_BOUND ( 'NONE', #496, .T. ) ;
#30255=DIRECTION ( 'NONE',  ( 0.000000000000000000, 0.000000000000000000, 1.000000000000000000 ) ) ;
#30256=PLANE ( 'NONE',  #34280 ) ;
#30259=CIRCLE ( 'NONE', #8664, 3.999999999999976019 ) ;
#30264=AXIS2_PLACEMENT_3D ( 'NONE', #132, #32868, #5625 ) ;
#30265=ORIENTED_EDGE ( 'NONE', *, *, #32473, .T. ) ;
#30267=DIRECTION ( 'NONE',  ( 1.000000000000000000, -0.000000000000000000, -0.000000000000000000 ) ) ;
#30272=( NAMED_UNIT ( * ) SI_UNIT ( $, .STERADIAN. ) SOLID_ANGLE_UNIT ( ) );
#30275=FACE_OUTER_BOUND ( 'NONE', #7743, .T. ) ;
#30280=CARTESIAN_POINT ( 'NONE',  ( -418.0000000000000000, 124.9999999999999574, -190.9999999999999716 ) ) ;
#30282=ORIENTED_EDGE ( 'NONE', *, *, #19412, .F. ) ;
#30285=DIRECTION ( 'NONE',  ( 0.000000000000000000, 0.000000000000000000, -1.000000000000000000 ) ) ;
#30286=CARTESIAN_POINT ( 'NONE',  ( 11.99999999999999645, 134.9999999999999432, -194.9999999999999432 ) ) ;
#30288=CARTESIAN_POINT ( 'NONE',  ( -11.99999999999998224, -134.9999999999999716, 194.9999999999999716 ) ) ;
#30289=AXIS2_PLACEMENT_3D ( 'NONE', #5107, #24328, #7255 ) ;
#30290=CIRCLE ( 'NONE', #10392, 7.999999999999979572 ) ;
#30296=LINE ( 'NONE', #1107, #25901 ) ;
#30297=CARTESIAN_POINT ( 'NONE',  ( 11.99999999999999645, 144.9999999999999147, 194.9999999999999716 ) ) ;
#30299=DIRECTION ( 'NONE',  ( 0.000000000000000000, 1.310824597558155437E-49, 1.000000000000000000 ) ) ;
#30302=VERTEX_POINT ( 'NONE', #490 ) ;
#30305=CIRCLE ( 'NONE', #9282, 4.000000000000003553 ) ;
#30307=ORIENTED_EDGE ( 'NONE', *, *, #16496, .T. ) ;
#30308=DIRECTION ( 'NONE',  ( 1.000000000000000000, 0.000000000000000000, 0.000000000000000000 ) ) ;
#30315=CARTESIAN_POINT ( 'NONE',  ( -410.0000000000000568, -105.0000000000000142, -101.9999999999999858 ) ) ;
#30317=ORIENTED_EDGE ( 'NONE', *, *, #32400, .F. ) ;
#30319=CARTESIAN_POINT ( 'NONE',  ( -414.0000000000000568, -105.0000000000000142, 187.0000000000000000 ) ) ;
#30322=EDGE_CURVE ( 'NONE', #18216, #8179, #33221, .T. ) ;
#30326=EDGE_CURVE ( 'NONE', #24869, #14949, #1538, .T. ) ;
#30328=EDGE_CURVE ( 'NONE', #7557, #904, #12060, .T. ) ;
#30329=AXIS2_PLACEMENT_3D ( 'NONE', #4211, #20602, #28784 ) ;
#30330=LINE ( 'NONE', #30149, #7921 ) ;
#30335=LINE ( 'NONE', #30153, #4927 ) ;
#30337=ORIENTED_EDGE ( 'NONE', *, *, #28977, .F. ) ;
#30338=VECTOR ( 'NONE', #34951, 1000.000000000000000 ) ;
#30339=CIRCLE ( 'NONE', #6439, 4.750000000000004441 ) ;
#30340=FACE_OUTER_BOUND ( 'NONE', #17196, .T. ) ;
#30341=VERTEX_POINT ( 'NONE', #6333 ) ;
#30347=ORIENTED_EDGE ( 'NONE', *, *, #14333, .F. ) ;
#30350=AXIS2_PLACEMENT_3D ( 'NONE', #14716, #28742, #20394 ) ;
#30351=ORIENTED_EDGE ( 'NONE', *, *, #20015, .T. ) ;
#30353=LINE ( 'NONE', #11325, #5087 ) ;
#30355=ORIENTED_EDGE ( 'NONE', *, *, #23070, .T. ) ;
#30357=CIRCLE ( 'NONE', #4778, 3.999999999999976019 ) ;
#30359=LINE ( 'NONE', #27686, #23273 ) ;
#30363=ORIENTED_EDGE ( 'NONE', *, *, #18944, .T. ) ;
#30364=ORIENTED_EDGE ( 'NONE', *, *, #22058, .T. ) ;
#30366=ADVANCED_FACE ( 'NONE', ( #20413, #33399 ), #17415, .T. ) ;
#30378=ORIENTED_EDGE ( 'NONE', *, *, #2083, .T. ) ;
#30380=LINE ( 'NONE', #30031, #32186 ) ;
#30384=AXIS2_PLACEMENT_3D ( 'NONE', #8426, #19300, #16994 ) ;
#30385=EDGE_CURVE ( 'NONE', #23416, #726, #22734, .T. ) ;
#30392=ADVANCED_FACE ( 'NONE', ( #22903 ), #8843, .F. ) ;
#30396=VECTOR ( 'NONE', #2715, 1000.000000000000000 ) ;
#30399=FACE_OUTER_BOUND ( 'NONE', #16904, .T. ) ;
#30402=LINE ( 'NONE', #5998, #24397 ) ;
#30412=VERTEX_POINT ( 'NONE', #3492 ) ;
#30419=ORIENTED_EDGE ( 'NONE', *, *, #32329, .T. ) ;
#30420=CIRCLE ( 'NONE', #15090, 7.999999999999979572 ) ;
#30424=DIRECTION ( 'NONE',  ( 8.433758354584418579E-81, -1.000000000000000000, -3.421138828918010427E-49 ) ) ;
#30426=DIRECTION ( 'NONE',  ( -1.000000000000000000, 0.000000000000000000, -5.546364386991661285E-52 ) ) ;
#30429=CARTESIAN_POINT ( 'NONE',  ( -414.0000000000000568, 124.9999999999999574, -187.0000000000000000 ) ) ;
#30431=EDGE_CURVE ( 'NONE', #11988, #7322, #28062, .T. ) ;
#30432=FACE_OUTER_BOUND ( 'NONE', #5092, .T. ) ;
#30433=EDGE_LOOP ( 'NONE', ( #236, #2087, #26252, #6842 ) ) ;
#30435=DIRECTION ( 'NONE',  ( 1.000000000000000000, 0.000000000000000000, 0.000000000000000000 ) ) ;
#30436=CARTESIAN_POINT ( 'NONE',  ( -442.0000000000000000, -125.0000000000000000, 159.0000000000000000 ) ) ;
#30437=DIRECTION ( 'NONE',  ( 0.000000000000000000, 0.000000000000000000, 1.000000000000000000 ) ) ;
#30440=LINE ( 'NONE', #14252, #8586 ) ;
#30442=LINE ( 'NONE', #3377, #9204 ) ;
#30444=EDGE_CURVE ( 'NONE', #17160, #23318, #25092, .T. ) ;
#30445=ORIENTED_EDGE ( 'NONE', *, *, #25717, .T. ) ;
#30447=VERTEX_POINT ( 'NONE', #14736 ) ;
#30452=EDGE_CURVE ( 'NONE', #9496, #28106, #12240, .T. ) ;
#30453=EDGE_CURVE ( 'NONE', #22841, #28422, #23088, .T. ) ;
#30454=CARTESIAN_POINT ( 'NONE',  ( -410.0000000000000568, -124.9999999999999858, -77.99999999999997158 ) ) ;
#30467=LINE ( 'NONE', #6060, #16568 ) ;
#30468=CARTESIAN_POINT ( 'NONE',  ( -12.00000000000001066, -145.0000000000000000, -158.9999999999999716 ) ) ;
#30469=VERTEX_POINT ( 'NONE', #25204 ) ;
#30470=DIRECTION ( 'NONE',  ( -1.232595164407830946E-32, 0.000000000000000000, -1.000000000000000000 ) ) ;
#30472=CARTESIAN_POINT ( 'NONE',  ( -365.0000000000000000, 114.9999999999999716, 126.0000000000000000 ) ) ;
#30473=ADVANCED_FACE ( 'NONE', ( #4190 ), #23932, .T. ) ;
#30481=CARTESIAN_POINT ( 'NONE',  ( -355.0000000000000000, 132.9999999999999716, 113.9999999999999858 ) ) ;
#30484=DIRECTION ( 'NONE',  ( 0.000000000000000000, 1.000000000000000000, 0.000000000000000000 ) ) ;
#30485=ORIENTED_EDGE ( 'NONE', *, *, #17901, .T. ) ;
#30486=CARTESIAN_POINT ( 'NONE',  ( -361.0000000000000000, -135.0000000000000000, 126.0000000000000000 ) ) ;
#30487=DIRECTION ( 'NONE',  ( 0.000000000000000000, -6.123233995736766036E-17, -1.000000000000000000 ) ) ;
#30488=AXIS2_PLACEMENT_3D ( 'NONE', #15724, #29583, #29045 ) ;
#30489=EDGE_LOOP ( 'NONE', ( #18598, #14173, #9001, #32801, #19652, #24079, #24799, #7143 ) ) ;
#30492=EDGE_LOOP ( 'NONE', ( #352, #11383, #17272, #9924 ) ) ;
#30493=EDGE_CURVE ( 'NONE', #34152, #707, #30259, .T. ) ;
#30494=ADVANCED_FACE ( 'NONE', ( #12574 ), #15423, .T. ) ;
#30498=EDGE_LOOP ( 'NONE', ( #35071, #6591, #26060, #2482, #26866, #14524, #1265, #32720 ) ) ;
#30502=VERTEX_POINT ( 'NONE', #23418 ) ;
#30506=ORIENTED_EDGE ( 'NONE', *, *, #26178, .T. ) ;
#30508=EDGE_CURVE ( 'NONE', #14034, #13474, #3528, .T. ) ;
#30512=CYLINDRICAL_SURFACE ( 'NONE', #25038, 7.999999999999979572 ) ;
#30513=CARTESIAN_POINT ( 'NONE',  ( -418.0000000000000000, -105.0000000000000142, 104.0000000000000142 ) ) ;
#30514=ORIENTED_EDGE ( 'NONE', *, *, #5891, .T. ) ;
#30515=AXIS2_PLACEMENT_3D ( 'NONE', #5662, #13696, #16558 ) ;
#30519=ORIENTED_EDGE ( 'NONE', *, *, #26787, .F. ) ;
#30525=DIRECTION ( 'NONE',  ( 0.000000000000000000, 0.000000000000000000, -1.000000000000000000 ) ) ;
#30526=VERTEX_POINT ( 'NONE', #18270 ) ;
#30533=CARTESIAN_POINT ( 'NONE',  ( -20.00000000000007461, 140.9999999999999716, -187.0000000000000000 ) ) ;
#30536=ORIENTED_EDGE ( 'NONE', *, *, #5207, .F. ) ;
#30539=VECTOR ( 'NONE', #29948, 1000.000000000000000 ) ;
#30540=EDGE_CURVE ( 'NONE', #19565, #26015, #26434, .T. ) ;
#30541=VERTEX_POINT ( 'NONE', #31941 ) ;
#30546=AXIS2_PLACEMENT_3D ( 'NONE', #28792, #15633, #2090 ) ;
#30547=CARTESIAN_POINT ( 'NONE',  ( 11.99999999999999645, -145.0000000000000000, 190.9999999999999716 ) ) ;
#30548=DIRECTION ( 'NONE',  ( 0.000000000000000000, 1.000000000000000000, 0.000000000000000000 ) ) ;
#30550=ORIENTED_EDGE ( 'NONE', *, *, #32480, .F. ) ;
#30554=AXIS2_PLACEMENT_3D ( 'NONE', #33206, #17040, #8297 ) ;
#30555=DIRECTION ( 'NONE',  ( 1.000000000000000000, 0.000000000000000000, 1.300283923313630633E-47 ) ) ;
#30556=DIRECTION ( 'NONE',  ( 0.000000000000000000, 1.000000000000000000, 1.224646799147353207E-16 ) ) ;
#30558=DIRECTION ( 'NONE',  ( 0.000000000000000000, 0.000000000000000000, -1.000000000000000000 ) ) ;
#30560=FACE_OUTER_BOUND ( 'NONE', #14081, .T. ) ;
#30562=VECTOR ( 'NONE', #13083, 1000.000000000000000 ) ;
#30563=CYLINDRICAL_SURFACE ( 'NONE', #16871, 4.000000000000003553 ) ;
#30565=LINE ( 'NONE', #17056, #24000 ) ;
#30566=EDGE_LOOP ( 'NONE', ( #9011, #18529, #19206, #13072, #22795, #12439, #3717, #5163 ) ) ;
#30567=VECTOR ( 'NONE', #29591, 1000.000000000000000 ) ;
#30571=DIRECTION ( 'NONE',  ( -0.000000000000000000, -0.000000000000000000, -1.000000000000000000 ) ) ;
#30572=FACE_OUTER_BOUND ( 'NONE', #34703, .T. ) ;
#30574=FACE_OUTER_BOUND ( 'NONE', #12509, .T. ) ;
#30576=FACE_OUTER_BOUND ( 'NONE', #24915, .T. ) ;
#30578=ORIENTED_EDGE ( 'NONE', *, *, #15762, .T. ) ;
#30580=VECTOR ( 'NONE', #31201, 1000.000000000000000 ) ;
#30588=DIRECTION ( 'NONE',  ( 0.000000000000000000, 1.131431318426415506E-52, 1.000000000000000000 ) ) ;
#30594=EDGE_CURVE ( 'NONE', #22581, #29789, #28934, .T. ) ;
#30595=CARTESIAN_POINT ( 'NONE',  ( -365.0000000000000000, -135.0000000000000000, 113.9999999999999858 ) ) ;
#30599=ORIENTED_EDGE ( 'NONE', *, *, #6264, .F. ) ;
#30600=VERTEX_POINT ( 'NONE', #21278 ) ;
#30602=VERTEX_POINT ( 'NONE', #18624 ) ;
#30603=CARTESIAN_POINT ( 'NONE',  ( -20.00000000000007461, -113.0000000000000000, -159.0000000000000000 ) ) ;
#30605=VERTEX_POINT ( 'NONE', #29466 ) ;
#30606=ORIENTED_EDGE ( 'NONE', *, *, #20256, .F. ) ;
#30607=DIRECTION ( 'NONE',  ( 1.000000000000000000, 0.000000000000000000, -1.848892746611746966E-32 ) ) ;
#30609=CARTESIAN_POINT ( 'NONE',  ( -499.9999999999999432, 108.9999999999999858, 162.9999999999999716 ) ) ;
#30611=CARTESIAN_POINT ( 'NONE',  ( -500.0000000000000000, -141.0000000000000000, 162.9999999999999716 ) ) ;
#30615=VECTOR ( 'NONE', #1432, 1000.000000000000000 ) ;
#30616=PLANE ( 'NONE',  #6875 ) ;
#30620=ORIENTED_EDGE ( 'NONE', *, *, #20683, .T. ) ;
#30621=CIRCLE ( 'NONE', #29478, 3.999999999999976019 ) ;
#30626=ORIENTED_EDGE ( 'NONE', *, *, #29780, .F. ) ;
#30627=ADVANCED_FACE ( 'NONE', ( #24279 ), #5938, .F. ) ;
#30628=CARTESIAN_POINT ( 'NONE',  ( -441.9999999999999432, -105.0000000000000142, 139.9999999999999716 ) ) ;
#30629=VECTOR ( 'NONE', #6683, 1000.000000000000000 ) ;
#30631=DIRECTION ( 'NONE',  ( -0.000000000000000000, 0.000000000000000000, -1.000000000000000000 ) ) ;
#30634=DIRECTION ( 'NONE',  ( 0.000000000000000000, 0.000000000000000000, -1.000000000000000000 ) ) ;
#30637=MECHANICAL_DESIGN_GEOMETRIC_PRESENTATION_REPRESENTATION('',(#15869),#2752);
#30638=CARTESIAN_POINT ( 'NONE',  ( -418.0000000000000568, 105.0000000000000142, 159.0000000000000000 ) ) ;
#30644=LINE ( 'NONE', #22279, #9733 ) ;
#30645=EDGE_CURVE ( 'NONE', #4681, #14225, #11130, .T. ) ;
#30646=LINE ( 'NONE', #11253, #9300 ) ;
#30652=ORIENTED_EDGE ( 'NONE', *, *, #10574, .F. ) ;
#30656=DIRECTION ( 'NONE',  ( 0.000000000000000000, 6.123233995736766036E-17, 1.000000000000000000 ) ) ;
#30659=UNCERTAINTY_MEASURE_WITH_UNIT (LENGTH_MEASURE( 1.000000000000000082E-05 ), #18957, 'distance_accuracy_value', 'NONE');
#30660=CARTESIAN_POINT ( 'NONE',  ( -15.99999999999998579, 144.9999999999999716, 187.0000000000000000 ) ) ;
#30661=ORIENTED_EDGE ( 'NONE', *, *, #32618, .F. ) ;
#30662=CARTESIAN_POINT ( 'NONE',  ( -430.0000000000000000, -119.0000000000000000, 109.9999999999999858 ) ) ;
#30663=FACE_OUTER_BOUND ( 'NONE', #15939, .T. ) ;
#30664=VECTOR ( 'NONE', #34836, 1000.000000000000000 ) ;
#30667=AXIS2_PLACEMENT_3D ( 'NONE', #8266, #21620, #7915 ) ;
#30669=EDGE_CURVE ( 'NONE', #10216, #34042, #24448, .T. ) ;
#30671=DIRECTION ( 'NONE',  ( 1.000000000000000000, 0.000000000000000000, -1.232595164407831220E-32 ) ) ;
#30672=ORIENTED_EDGE ( 'NONE', *, *, #16978, .F. ) ;
#30676=EDGE_LOOP ( 'NONE', ( #17108, #7409, #14060, #8511 ) ) ;
#30678=CARTESIAN_POINT ( 'NONE',  ( -20.00000000000007461, 136.9999999999999432, 194.9999999999999716 ) ) ;
#30681=DIRECTION ( 'NONE',  ( 0.000000000000000000, 1.000000000000000000, -1.131431318426415506E-52 ) ) ;
#30682=CARTESIAN_POINT ( 'NONE',  ( -441.9999999999999432, -105.0000000000000142, -69.99999999999998579 ) ) ;
#30687=ORIENTED_EDGE ( 'NONE', *, *, #28029, .F. ) ;
#30690=ORIENTED_EDGE ( 'NONE', *, *, #2134, .F. ) ;
#30699=DIRECTION ( 'NONE',  ( -1.000000000000000000, 0.000000000000000000, 0.000000000000000000 ) ) ;
#30706=ADVANCED_FACE ( 'NONE', ( #21451 ), #8448, .F. ) ;
#30707=ORIENTED_EDGE ( 'NONE', *, *, #7167, .F. ) ;
#30710=ORIENTED_EDGE ( 'NONE', *, *, #6575, .T. ) ;
#30714=VERTEX_POINT ( 'NONE', #10604 ) ;
#30715=VERTEX_POINT ( 'NONE', #13447 ) ;
#30716=PLANE ( 'NONE',  #12189 ) ;
#30721=ORIENTED_EDGE ( 'NONE', *, *, #31833, .T. ) ;
#30724=DIRECTION ( 'NONE',  ( 3.040835319149746090E-31, 1.000000000000000000, -3.748118910144520367E-63 ) ) ;
#30726=DIRECTION ( 'NONE',  ( 1.000000000000000000, -0.000000000000000000, -0.000000000000000000 ) ) ;
#30727=LINE ( 'NONE', #14729, #11398 ) ;
#30728=DIRECTION ( 'NONE',  ( 0.000000000000000000, -1.000000000000000000, -5.053935297177146739E-49 ) ) ;
#30730=VERTEX_POINT ( 'NONE', #16655 ) ;
#30731=CARTESIAN_POINT ( 'NONE',  ( 19.99999999999998934, 4.559999999999909015, 177.7400000000000091 ) ) ;
#30735=ORIENTED_EDGE ( 'NONE', *, *, #9731, .T. ) ;
#30737=CARTESIAN_POINT ( 'NONE',  ( -442.0000000000000000, -125.0000000000000000, 162.9999999999999716 ) ) ;
#30738=ORIENTED_EDGE ( 'NONE', *, *, #33182, .T. ) ;
#30742=AXIS2_PLACEMENT_3D ( 'NONE', #19344, #30184, #5259 ) ;
#30744=DIRECTION ( 'NONE',  ( 0.000000000000000000, 0.000000000000000000, -1.000000000000000000 ) ) ;
#30746=CARTESIAN_POINT ( 'NONE',  ( -365.0000000000000000, -135.0000000000000000, 113.9999999999999858 ) ) ;
#30750=CIRCLE ( 'NONE', #13128, 7.999999999999979572 ) ;
#30753=DIRECTION ( 'NONE',  ( 0.000000000000000000, 1.000000000000000000, 0.000000000000000000 ) ) ;
#30755=DIRECTION ( 'NONE',  ( 0.000000000000000000, -1.000000000000000000, -1.224646799147353207E-16 ) ) ;
#30756=CARTESIAN_POINT ( 'NONE',  ( -365.0000000000000000, -125.0000000000000284, 168.9999999999999716 ) ) ;
#30757=ORIENTED_EDGE ( 'NONE', *, *, #29893, .F. ) ;
#30761=( NAMED_UNIT ( * ) SI_UNIT ( $, .STERADIAN. ) SOLID_ANGLE_UNIT ( ) );
#30762=PLANE ( 'NONE',  #32476 ) ;
#30764=CYLINDRICAL_SURFACE ( 'NONE', #23573, 2.000000000000001776 ) ;
#30766=ORIENTED_EDGE ( 'NONE', *, *, #2391, .T. ) ;
#30769=DIRECTION ( 'NONE',  ( 0.000000000000000000, 0.000000000000000000, 1.000000000000000000 ) ) ;
#30770=VERTEX_POINT ( 'NONE', #33176 ) ;
#30775=ORIENTED_EDGE ( 'NONE', *, *, #31504, .T. ) ;
#30776=VERTEX_POINT ( 'NONE', #25517 ) ;
#30780=DIRECTION ( 'NONE',  ( -1.000000000000000000, -3.040835319149746528E-31, -1.232595164407830946E-32 ) ) ;
#30782=EDGE_LOOP ( 'NONE', ( #31966, #19180, #29183, #24842 ) ) ;
#30784=VECTOR ( 'NONE', #16973, 1000.000000000000000 ) ;
#30787=DIRECTION ( 'NONE',  ( 0.000000000000000000, 1.000000000000000000, 5.053935297177146739E-49 ) ) ;
#30790=DIRECTION ( 'NONE',  ( 0.000000000000000000, 1.000000000000000000, 1.224646799147353207E-16 ) ) ;
#30792=AXIS2_PLACEMENT_3D ( 'NONE', #9588, #25417, #22761 ) ;
#30796=ORIENTED_EDGE ( 'NONE', *, *, #33045, .T. ) ;
#30799=DIRECTION ( 'NONE',  ( 1.000000000000000000, 0.000000000000000000, 5.546364386991661285E-52 ) ) ;
#30801=FACE_OUTER_BOUND ( 'NONE', #21765, .T. ) ;
#30804=ORIENTED_EDGE ( 'NONE', *, *, #19861, .T. ) ;
#30809=DIRECTION ( 'NONE',  ( -1.000000000000000000, 0.000000000000000000, 0.000000000000000000 ) ) ;
#30814=EDGE_CURVE ( 'NONE', #7154, #21502, #31382, .T. ) ;
#30816=CARTESIAN_POINT ( 'NONE',  ( -500.0000000000000000, -105.0000000000000142, 162.9999999999999716 ) ) ;
#30817=DIRECTION ( 'NONE',  ( 0.000000000000000000, 0.000000000000000000, 1.000000000000000000 ) ) ;
#30823=EDGE_CURVE ( 'NONE', #6516, #10776, #3969, .T. ) ;
#30832=DIRECTION ( 'NONE',  ( 1.000000000000000000, -3.540705920434608777E-32, 2.891205793294675368E-16 ) ) ;
#30834=ORIENTED_EDGE ( 'NONE', *, *, #13303, .T. ) ;
#30837=VERTEX_POINT ( 'NONE', #17371 ) ;
#30839=EDGE_LOOP ( 'NONE', ( #1734, #15661, #6963, #26895 ) ) ;
#30841=CARTESIAN_POINT ( 'NONE',  ( 11.99999999999999645, -145.0000000000000000, -158.9999999999999716 ) ) ;
#30842=VERTEX_POINT ( 'NONE', #8798 ) ;
#30844=FACE_OUTER_BOUND ( 'NONE', #23234, .T. ) ;
#30853=DIRECTION ( 'NONE',  ( 0.000000000000000000, 1.000000000000000000, 1.224646799147353207E-16 ) ) ;
#30855=DIRECTION ( 'NONE',  ( 1.000000000000000000, 0.000000000000000000, 0.000000000000000000 ) ) ;
#30859=DIRECTION ( 'NONE',  ( -1.848892746611746419E-32, -6.842277657836020854E-49, 1.000000000000000000 ) ) ;
#30860=DIRECTION ( 'NONE',  ( 1.300283923313630633E-47, 0.000000000000000000, -1.000000000000000000 ) ) ;
#30866=CARTESIAN_POINT ( 'NONE',  ( -441.9999999999999432, 105.0000000000000142, 190.9999999999999716 ) ) ;
#30871=ORIENTED_EDGE ( 'NONE', *, *, #21961, .T. ) ;
#30873=CARTESIAN_POINT ( 'NONE',  ( -442.0000000000000000, 104.9999999999999858, -159.0000000000000000 ) ) ;
#30881=ORIENTED_EDGE ( 'NONE', *, *, #20259, .T. ) ;
#30882=VERTEX_POINT ( 'NONE', #3800 ) ;
#30888=LINE ( 'NONE', #17730, #8756 ) ;
#30891=EDGE_CURVE ( 'NONE', #22434, #17624, #6820, .T. ) ;
#30895=FACE_OUTER_BOUND ( 'NONE', #6450, .T. ) ;
#30897=ORIENTED_EDGE ( 'NONE', *, *, #19899, .F. ) ;
#30898=DIRECTION ( 'NONE',  ( 0.000000000000000000, -5.145227585319922065E-49, -1.000000000000000000 ) ) ;
#30900=CARTESIAN_POINT ( 'NONE',  ( -355.0000000000000000, 114.9999999999999716, 126.0000000000000000 ) ) ;
#30901=EDGE_CURVE ( 'NONE', #14883, #6108, #29723, .T. ) ;
#30902=CARTESIAN_POINT ( 'NONE',  ( 12.00000000000001066, -32.99999999999997158, 154.9999999999999716 ) ) ;
#30903=CARTESIAN_POINT ( 'NONE',  ( -418.0000000000000000, 113.0000000000000000, -155.0000000000000000 ) ) ;
#30906=AXIS2_PLACEMENT_3D ( 'NONE', #13624, #19323, #10949 ) ;
#30908=ORIENTED_EDGE ( 'NONE', *, *, #30452, .T. ) ;
#30911=DIRECTION ( 'NONE',  ( 0.000000000000000000, 7.888609052210118054E-31, 1.000000000000000000 ) ) ;
#30912=EDGE_LOOP ( 'NONE', ( #1680, #3551, #1644, #29445 ) ) ;
#30914=EDGE_CURVE ( 'NONE', #13611, #9466, #27415, .T. ) ;
#30915=DIRECTION ( 'NONE',  ( 0.000000000000000000, 0.000000000000000000, -1.000000000000000000 ) ) ;
#30917=DIRECTION ( 'NONE',  ( 0.000000000000000000, 5.145227585319922065E-49, 1.000000000000000000 ) ) ;
#30919=VECTOR ( 'NONE', #10366, 1000.000000000000000 ) ;
#30920=ORIENTED_EDGE ( 'NONE', *, *, #18806, .T. ) ;
#30922=PLANE ( 'NONE',  #23060 ) ;
#30928=DIRECTION ( 'NONE',  ( 0.000000000000000000, 1.000000000000000000, 5.053935297177146739E-49 ) ) ;
#30929=EDGE_LOOP ( 'NONE', ( #28805, #10631, #7176, #29006, #1346 ) ) ;
#30939=ORIENTED_EDGE ( 'NONE', *, *, #21608, .F. ) ;
#30940=ORIENTED_EDGE ( 'NONE', *, *, #30431, .T. ) ;
#30946=ORIENTED_EDGE ( 'NONE', *, *, #1447, .F. ) ;
#30951=AXIS2_PLACEMENT_3D ( 'NONE', #30986, #33649, #17488 ) ;
#30952=CYLINDRICAL_SURFACE ( 'NONE', #6088, 7.999999999999992895 ) ;
#30955=ORIENTED_EDGE ( 'NONE', *, *, #28480, .F. ) ;
#30957=CIRCLE ( 'NONE', #23555, 7.999999999999979572 ) ;
#30962=DIRECTION ( 'NONE',  ( -1.000000000000000000, 0.000000000000000000, 0.000000000000000000 ) ) ;
#30963=CIRCLE ( 'NONE', #10509, 7.999999999999979572 ) ;
#30968=DIRECTION ( 'NONE',  ( 0.000000000000000000, 0.000000000000000000, 1.000000000000000000 ) ) ;
#30969=ORIENTED_EDGE ( 'NONE', *, *, #18667, .F. ) ;
#30973=ORIENTED_EDGE ( 'NONE', *, *, #22091, .F. ) ;
#30974=VECTOR ( 'NONE', #14764, 1000.000000000000000 ) ;
#30975=ADVANCED_FACE ( 'NONE', ( #24198 ), #7648, .T. ) ;
#30976=VECTOR ( 'NONE', #22113, 1000.000000000000000 ) ;
#30979=ADVANCED_FACE ( 'NONE', ( #8178 ), #35077, .F. ) ;
#30980=VECTOR ( 'NONE', #19720, 1000.000000000000000 ) ;
#30985=CLOSED_SHELL ( 'NONE', ( #34850, #24059, #1992, #28098, #20623, #16811, #15007, #21706, #14880, #170, #20808, #31739, #18866, #5330, #34230, #1838, #31578, #26432 ) ) ;
#30986=CARTESIAN_POINT ( 'NONE',  ( -349.0000000000000000, -125.0000000000000284, 181.0000000000000000 ) ) ;
#30987=LINE ( 'NONE', #19789, #12427 ) ;
#30988=ORIENTED_EDGE ( 'NONE', *, *, #23464, .T. ) ;
#30989=ORIENTED_EDGE ( 'NONE', *, *, #29998, .F. ) ;
#30990=CARTESIAN_POINT ( 'NONE',  ( -19.99999999999998934, 4.559999999999909015, 177.7400000000000091 ) ) ;
#30996=DIRECTION ( 'NONE',  ( 1.000000000000000000, 0.000000000000000000, 0.000000000000000000 ) ) ;
#30997=AXIS2_PLACEMENT_3D ( 'NONE', #2395, #13446, #32295 ) ;
#31004=DIRECTION ( 'NONE',  ( 0.000000000000000000, 0.000000000000000000, -1.000000000000000000 ) ) ;
#31005=VECTOR ( 'NONE', #19031, 1000.000000000000000 ) ;
#31009=VECTOR ( 'NONE', #20220, 1000.000000000000000 ) ;
#31014=ORIENTED_EDGE ( 'NONE', *, *, #1007, .F. ) ;
#31019=AXIS2_PLACEMENT_3D ( 'NONE', #20055, #5968, #30898 ) ;
#31020=ADVANCED_FACE ( 'NONE', ( #5328 ), #27052, .T. ) ;
#31021=CARTESIAN_POINT ( 'NONE',  ( -361.0000000000000000, 134.9999999999999716, 128.0000000000000000 ) ) ;
#31022=ORIENTED_EDGE ( 'NONE', *, *, #20187, .F. ) ;
#31026=EDGE_CURVE ( 'NONE', #31513, #28476, #28718, .T. ) ;
#31031=CYLINDRICAL_SURFACE ( 'NONE', #3284, 7.999999999999979572 ) ;
#31032=FACE_OUTER_BOUND ( 'NONE', #22988, .T. ) ;
#31035=DIRECTION ( 'NONE',  ( 0.000000000000000000, 0.000000000000000000, 1.000000000000000000 ) ) ;
#31040=CARTESIAN_POINT ( 'NONE',  ( -442.0000000000000000, 145.0000000000000000, -175.0000000000000000 ) ) ;
#31042=ORIENTED_EDGE ( 'NONE', *, *, #10214, .T. ) ;
#31050=DIRECTION ( 'NONE',  ( 0.000000000000000000, 0.000000000000000000, -1.000000000000000000 ) ) ;
#31051=PLANE ( 'NONE',  #16766 ) ;
#31052=FACE_OUTER_BOUND ( 'NONE', #22353, .T. ) ;
#31053=AXIS2_PLACEMENT_3D ( 'NONE', #3266, #33346, #14140 ) ;
#31055=ORIENTED_EDGE ( 'NONE', *, *, #9724, .T. ) ;
#31059=AXIS2_PLACEMENT_3D ( 'NONE', #13577, #24936, #571 ) ;
#31069=ORIENTED_EDGE ( 'NONE', *, *, #7540, .T. ) ;
#31071=DIRECTION ( 'NONE',  ( 0.000000000000000000, -0.000000000000000000, -1.000000000000000000 ) ) ;
#31073=ADVANCED_FACE ( 'NONE', ( #30432 ), #889, .F. ) ;
#31076=CARTESIAN_POINT ( 'NONE',  ( -499.9999999999999432, 136.9999999999999432, 162.9999999999999716 ) ) ;
#31077=CARTESIAN_POINT ( 'NONE',  ( 19.99999999999998224, 134.9999999999999432, -162.9999999999999432 ) ) ;
#31079=EDGE_LOOP ( 'NONE', ( #16458, #4163, #11151, #3771 ) ) ;
#31080=EDGE_CURVE ( 'NONE', #8775, #18155, #22605, .T. ) ;
#31082=LINE ( 'NONE', #28922, #18543 ) ;
#31083=CARTESIAN_POINT ( 'NONE',  ( -70.00000000000000000, 75.55999999999990280, 177.7400000000000091 ) ) ;
#31087=CARTESIAN_POINT ( 'NONE',  ( -442.0000000000000000, 105.0000000000000142, 162.9999999999999716 ) ) ;
#31090=EDGE_LOOP ( 'NONE', ( #2301, #24363 ) ) ;
#31091=VECTOR ( 'NONE', #24821, 1000.000000000000000 ) ;
#31093=CARTESIAN_POINT ( 'NONE',  ( -355.0000000000000000, 134.9999999999999716, 113.9999999999999858 ) ) ;
#31094=EDGE_CURVE ( 'NONE', #27019, #22138, #5825, .T. ) ;
#31097=CARTESIAN_POINT ( 'NONE',  ( -445.9999999999999432, -125.0000000000000000, 107.9999999999999858 ) ) ;
#31104=ORIENTED_EDGE ( 'NONE', *, *, #18667, .T. ) ;
#31105=CARTESIAN_POINT ( 'NONE',  ( 11.99999999999999645, 124.9999999999999716, 155.0000000000000000 ) ) ;
#31108=VERTEX_POINT ( 'NONE', #30609 ) ;
#31113=VERTEX_POINT ( 'NONE', #25252 ) ;
#31116=CARTESIAN_POINT ( 'NONE',  ( 15.99999999999998579, 4.559999999999909015, 177.7400000000000091 ) ) ;
#31117=DIRECTION ( 'NONE',  ( 0.000000000000000000, 1.000000000000000000, 5.053935297177146739E-49 ) ) ;
#31121=ADVANCED_FACE ( 'NONE', ( #24898 ), #6028, .T. ) ;
#31124=CARTESIAN_POINT ( 'NONE',  ( -414.0000000000000568, 105.0000000000000142, 187.0000000000000000 ) ) ;
#31128=DIRECTION ( 'NONE',  ( -0.000000000000000000, 1.000000000000000000, -0.000000000000000000 ) ) ;
#31135=ORIENTED_EDGE ( 'NONE', *, *, #29893, .T. ) ;
#31138=ORIENTED_EDGE ( 'NONE', *, *, #1601, .F. ) ;
#31139=CARTESIAN_POINT ( 'NONE',  ( -355.0000000000000000, -135.0000000000000000, 113.9999999999999858 ) ) ;
#31140=CARTESIAN_POINT ( 'NONE',  ( 15.99999999999998579, -115.0000000000000000, 174.9999999999999432 ) ) ;
#31142=CARTESIAN_POINT ( 'NONE',  ( -500.0000000000000000, -137.0000000000000000, 187.0000000000000000 ) ) ;
#31143=EDGE_CURVE ( 'NONE', #26377, #5208, #30247, .T. ) ;
#31145=VECTOR ( 'NONE', #17405, 1000.000000000000000 ) ;
#31148=PLANE ( 'NONE',  #13756 ) ;
#31156=ORIENTED_EDGE ( 'NONE', *, *, #32694, .F. ) ;
#31159=LINE ( 'NONE', #17646, #20477 ) ;
#31161=CARTESIAN_POINT ( 'NONE',  ( -418.0000000000000000, 105.0000000000000000, -69.99999999999998579 ) ) ;
#31166=ORIENTED_EDGE ( 'NONE', *, *, #32887, .T. ) ;
#31169=DIRECTION ( 'NONE',  ( 1.000000000000000000, 0.000000000000000000, 0.000000000000000000 ) ) ;
#31170=PLANE ( 'NONE',  #20540 ) ;
#31171=ORIENTED_EDGE ( 'NONE', *, *, #5480, .F. ) ;
#31173=CYLINDRICAL_SURFACE ( 'NONE', #8904, 7.999999999999986677 ) ;
#31174=MECHANICAL_DESIGN_GEOMETRIC_PRESENTATION_REPRESENTATION('',(#18605),#26614);
#31176=CARTESIAN_POINT ( 'NONE',  ( -19.99999999999998934, -145.0000000000000000, 187.0000000000000000 ) ) ;
#31177=DIRECTION ( 'NONE',  ( -1.000000000000000000, 0.000000000000000000, 1.232595164407831220E-32 ) ) ;
#31181=DIRECTION ( 'NONE',  ( -0.000000000000000000, 1.000000000000000000, -0.000000000000000000 ) ) ;
#31183=EDGE_CURVE ( 'NONE', #22142, #24957, #23299, .T. ) ;
#31187=DIRECTION ( 'NONE',  ( 0.000000000000000000, 0.000000000000000000, -1.000000000000000000 ) ) ;
#31191=VERTEX_POINT ( 'NONE', #9429 ) ;
#31195=ORIENTED_EDGE ( 'NONE', *, *, #18673, .F. ) ;
#31196=ORIENTED_EDGE ( 'NONE', *, *, #26968, .T. ) ;
#31200=ORIENTED_EDGE ( 'NONE', *, *, #21912, .T. ) ;
#31201=DIRECTION ( 'NONE',  ( 1.000000000000000000, -0.000000000000000000, -0.000000000000000000 ) ) ;
#31202=FACE_OUTER_BOUND ( 'NONE', #32168, .T. ) ;
#31203=ORIENTED_EDGE ( 'NONE', *, *, #7752, .F. ) ;
#31206=DIRECTION ( 'NONE',  ( -1.000000000000000000, 0.000000000000000000, 0.000000000000000000 ) ) ;
#31207=CARTESIAN_POINT ( 'NONE',  ( -12.00000000000001243, 134.9999999999998863, 194.9999999999999716 ) ) ;
#31208=DIRECTION ( 'NONE',  ( 1.000000000000000000, 3.040835319149746090E-31, 1.232595164407830946E-32 ) ) ;
#31211=FACE_OUTER_BOUND ( 'NONE', #2132, .T. ) ;
#31213=VECTOR ( 'NONE', #17407, 1000.000000000000000 ) ;
#31214=CARTESIAN_POINT ( 'NONE',  ( -355.0000000000000000, 118.9999999999999716, 126.0000000000000000 ) ) ;
#31218=EDGE_CURVE ( 'NONE', #6516, #27008, #20285, .T. ) ;
#31219=DIRECTION ( 'NONE',  ( 1.000000000000000000, 0.000000000000000000, 0.000000000000000000 ) ) ;
#31223=CIRCLE ( 'NONE', #11899, 4.750000000000004441 ) ;
#31226=EDGE_LOOP ( 'NONE', ( #6447, #32070, #34608, #9690, #27885, #17000, #2728, #17521, #28070 ) ) ;
#31227=EDGE_CURVE ( 'NONE', #423, #24841, #5244, .T. ) ;
#31228=DIRECTION ( 'NONE',  ( 0.000000000000000000, 0.000000000000000000, -1.000000000000000000 ) ) ;
#31229=DIRECTION ( 'NONE',  ( 3.040835319149746090E-31, 1.000000000000000000, -3.748118910144520367E-63 ) ) ;
#31231=VECTOR ( 'NONE', #19489, 1000.000000000000000 ) ;
#31232=VERTEX_POINT ( 'NONE', #17279 ) ;
#31236=ORIENTED_EDGE ( 'NONE', *, *, #5235, .T. ) ;
#31239=ORIENTED_EDGE ( 'NONE', *, *, #5611, .F. ) ;
#31242=DIRECTION ( 'NONE',  ( 0.000000000000000000, 0.000000000000000000, -1.000000000000000000 ) ) ;
#31246=CARTESIAN_POINT ( 'NONE',  ( -449.9999999999999432, -105.0000000000000142, 107.9999999999999574 ) ) ;
#31247=DIRECTION ( 'NONE',  ( 0.000000000000000000, 0.000000000000000000, -1.000000000000000000 ) ) ;
#31252=DIRECTION ( 'NONE',  ( -1.000000000000000000, 0.000000000000000000, -1.300283923313630633E-47 ) ) ;
#31254=ORIENTED_EDGE ( 'NONE', *, *, #18673, .T. ) ;
#31256=DIRECTION ( 'NONE',  ( -3.469446951953832974E-18, -1.000000000000000000, -7.888609052210116302E-31 ) ) ;
#31257=EDGE_CURVE ( 'NONE', #29621, #28835, #18366, .T. ) ;
#31258=CARTESIAN_POINT ( 'NONE',  ( -70.00000000000000000, 75.55999999999990280, -172.9900000000000091 ) ) ;
#31259=EDGE_LOOP ( 'NONE', ( #11031, #21991, #8019, #16899, #29005 ) ) ;
#31262=ORIENTED_EDGE ( 'NONE', *, *, #3327, .F. ) ;
#31263=EDGE_CURVE ( 'NONE', #34740, #3207, #3720, .T. ) ;
#31264=CARTESIAN_POINT ( 'NONE',  ( -500.0000000000000000, 104.9999999999999858, 155.0000000000000000 ) ) ;
#31272=CARTESIAN_POINT ( 'NONE',  ( -449.9999999999999432, -104.9999999999999858, -162.9999999999999716 ) ) ;
#31273=EDGE_CURVE ( 'NONE', #7312, #25172, #6384, .T. ) ;
#31280=DIRECTION ( 'NONE',  ( 1.000000000000000000, 0.000000000000000000, -1.848892746611746966E-32 ) ) ;
#31283=FACE_OUTER_BOUND ( 'NONE', #28348, .T. ) ;
#31284=ORIENTED_EDGE ( 'NONE', *, *, #26746, .F. ) ;
#31285=ORIENTED_EDGE ( 'NONE', *, *, #33516, .T. ) ;
#31291=DIRECTION ( 'NONE',  ( 0.000000000000000000, 0.000000000000000000, -1.000000000000000000 ) ) ;
#31293=VECTOR ( 'NONE', #18657, 1000.000000000000000 ) ;
#31296=ORIENTED_EDGE ( 'NONE', *, *, #18312, .F. ) ;
#31297=DIRECTION ( 'NONE',  ( 0.000000000000000000, 0.000000000000000000, -1.000000000000000000 ) ) ;
#31300=EDGE_CURVE ( 'NONE', #1893, #26714, #14960, .T. ) ;
#31301=FACE_OUTER_BOUND ( 'NONE', #32518, .T. ) ;
#31302=AXIS2_PLACEMENT_3D ( 'NONE', #22638, #33311, #33124 ) ;
#31303=EDGE_CURVE ( 'NONE', #30004, #3035, #1850, .T. ) ;
#31308=CARTESIAN_POINT ( 'NONE',  ( 19.99999999999998934, 4.559999999999908127, -177.7400000000000091 ) ) ;
#31310=ORIENTED_EDGE ( 'NONE', *, *, #22745, .T. ) ;
#31312=CIRCLE ( 'NONE', #28475, 8.000000000000007105 ) ;
#31316=LINE ( 'NONE', #19040, #7856 ) ;
#31319=EDGE_LOOP ( 'NONE', ( #21883, #14438, #19576, #27433 ) ) ;
#31320=LINE ( 'NONE', #20131, #29851 ) ;
#31323=EDGE_CURVE ( 'NONE', #28665, #15358, #26132, .T. ) ;
#31325=LINE ( 'NONE', #6933, #34918 ) ;
#31326=DIRECTION ( 'NONE',  ( -0.000000000000000000, -1.000000000000000000, -0.000000000000000000 ) ) ;
#31328=ORIENTED_EDGE ( 'NONE', *, *, #5604, .F. ) ;
#31329=VERTEX_POINT ( 'NONE', #19933 ) ;
#31336=VERTEX_POINT ( 'NONE', #15830 ) ;
#31339=ORIENTED_EDGE ( 'NONE', *, *, #33877, .F. ) ;
#31340=CARTESIAN_POINT ( 'NONE',  ( -12.00000000000003908, -134.9999999999999716, -154.9999999999999716 ) ) ;
#31342=VECTOR ( 'NONE', #23197, 1000.000000000000000 ) ;
#31343=DIRECTION ( 'NONE',  ( 0.000000000000000000, -1.000000000000000000, 6.123233995736766036E-17 ) ) ;
#31346=EDGE_CURVE ( 'NONE', #1780, #6336, #7603, .T. ) ;
#31352=EDGE_LOOP ( 'NONE', ( #18390, #28912, #1379, #4166, #4290, #11458, #30091, #32817 ) ) ;
#31355=VECTOR ( 'NONE', #31439, 1000.000000000000000 ) ;
#31356=AXIS2_PLACEMENT_3D ( 'NONE', #14875, #31573, #1339 ) ;
#31365=AXIS2_PLACEMENT_3D ( 'NONE', #654, #12054, #23081 ) ;
#31366=EDGE_CURVE ( 'NONE', #11554, #29991, #27014, .T. ) ;
#31372=ORIENTED_EDGE ( 'NONE', *, *, #2133, .T. ) ;
#31374=DIRECTION ( 'NONE',  ( -0.000000000000000000, 0.000000000000000000, 1.000000000000000000 ) ) ;
#31378=EDGE_LOOP ( 'NONE', ( #13211, #24136, #12536, #23457 ) ) ;
#31379=MECHANICAL_DESIGN_GEOMETRIC_PRESENTATION_REPRESENTATION('',(#4071),#8073);
#31380=CARTESIAN_POINT ( 'NONE',  ( 0.000000000000000000, -115.0000000000000000, 0.000000000000000000 ) ) ;
#31382=CIRCLE ( 'NONE', #29119, 7.999999999999979572 ) ;
#31383=DIRECTION ( 'NONE',  ( -1.000000000000000000, 0.000000000000000000, -5.546364386991661285E-52 ) ) ;
#31385=CIRCLE ( 'NONE', #703, 7.999999999999952038 ) ;
#31389=CARTESIAN_POINT ( 'NONE',  ( 0.000000000000000000, -55.00000000000000711, 0.000000000000000000 ) ) ;
#31391=LINE ( 'NONE', #17891, #33131 ) ;
#31397=DIRECTION ( 'NONE',  ( -0.000000000000000000, -0.000000000000000000, 1.000000000000000000 ) ) ;
#31403=ORIENTED_EDGE ( 'NONE', *, *, #19412, .T. ) ;
#31407=VERTEX_POINT ( 'NONE', #2445 ) ;
#31409=ORIENTED_EDGE ( 'NONE', *, *, #27436, .T. ) ;
#31411=DIRECTION ( 'NONE',  ( -1.000000000000000000, 0.000000000000000000, -5.546364386991661285E-52 ) ) ;
#31412=EDGE_CURVE ( 'NONE', #25358, #13175, #4125, .T. ) ;
#31415=DIRECTION ( 'NONE',  ( 0.000000000000000000, 0.000000000000000000, 1.000000000000000000 ) ) ;
#31416=DIRECTION ( 'NONE',  ( -3.469446951953832974E-18, -1.000000000000000000, -7.888609052210116302E-31 ) ) ;
#31417=VERTEX_POINT ( 'NONE', #1919 ) ;
#31418=ORIENTED_EDGE ( 'NONE', *, *, #9583, .T. ) ;
#31419=CARTESIAN_POINT ( 'NONE',  ( 19.99999999999998934, -124.9999999999999432, -186.9999999999999716 ) ) ;
#31420=DIRECTION ( 'NONE',  ( 1.000000000000000000, 3.469446951953834515E-18, 0.000000000000000000 ) ) ;
#31421=CARTESIAN_POINT ( 'NONE',  ( -12.00000000000001066, -28.99999999999999645, -175.0000000000000000 ) ) ;
#31424=ORIENTED_EDGE ( 'NONE', *, *, #21585, .F. ) ;
#31433=AXIS2_PLACEMENT_3D ( 'NONE', #19771, #13895, #16580 ) ;
#31436=CARTESIAN_POINT ( 'NONE',  ( 11.99999999999999645, 144.9999999999999716, 190.9999999999999716 ) ) ;
#31439=DIRECTION ( 'NONE',  ( 2.891205793294675861E-16, 0.000000000000000000, 1.000000000000000000 ) ) ;
#31441=ORIENTED_EDGE ( 'NONE', *, *, #22901, .F. ) ;
#31444=EDGE_CURVE ( 'NONE', #9057, #26143, #10114, .T. ) ;
#31448=DIRECTION ( 'NONE',  ( -1.000000000000000000, -3.469446951953834515E-18, 0.000000000000000000 ) ) ;
#31449=EDGE_CURVE ( 'NONE', #26588, #26110, #20976, .T. ) ;
#31453=AXIS2_PLACEMENT_3D ( 'NONE', #15784, #26615, #26262 ) ;
#31461=ADVANCED_FACE ( 'NONE', ( #7783 ), #32345, .F. ) ;
#31462=CARTESIAN_POINT ( 'NONE',  ( -12.00000000000001066, 124.9999999999999716, 155.0000000000000000 ) ) ;
#31464=DIRECTION ( 'NONE',  ( -0.000000000000000000, -1.000000000000000000, -0.000000000000000000 ) ) ;
#31465=DIRECTION ( 'NONE',  ( 1.000000000000000000, 3.469446951953834515E-18, 0.000000000000000000 ) ) ;
#31470=CARTESIAN_POINT ( 'NONE',  ( -418.0000000000000568, -105.0000000000000142, -109.9999999999999574 ) ) ;
#31472=ORIENTED_EDGE ( 'NONE', *, *, #11577, .T. ) ;
#31473=VECTOR ( 'NONE', #19210, 1000.000000000000000 ) ;
#31474=CARTESIAN_POINT ( 'NONE',  ( 19.99999999999998934, -56.99999999999997868, 154.9999999999999716 ) ) ;
#31485=ORIENTED_EDGE ( 'NONE', *, *, #27234, .T. ) ;
#31487=EDGE_LOOP ( 'NONE', ( #13773, #28546, #30445, #3599 ) ) ;
#31493=DIRECTION ( 'NONE',  ( -3.040835319149746528E-31, -1.000000000000000000, 0.000000000000000000 ) ) ;
#31495=VECTOR ( 'NONE', #16596, 1000.000000000000000 ) ;
#31498=DIRECTION ( 'NONE',  ( 0.000000000000000000, 0.000000000000000000, 1.000000000000000000 ) ) ;
#31500=AXIS2_PLACEMENT_3D ( 'NONE', #7338, #6648, #34060 ) ;
#31504=EDGE_CURVE ( 'NONE', #26019, #4201, #13833, .T. ) ;
#31513=VERTEX_POINT ( 'NONE', #16702 ) ;
#31518=DIRECTION ( 'NONE',  ( 1.000000000000000000, 0.000000000000000000, -1.300283923313630633E-47 ) ) ;
#31520=CIRCLE ( 'NONE', #5917, 7.999999999999979572 ) ;
#31521=DIRECTION ( 'NONE',  ( 0.000000000000000000, 0.000000000000000000, 1.000000000000000000 ) ) ;
#31525=DIRECTION ( 'NONE',  ( 0.000000000000000000, 0.000000000000000000, -1.000000000000000000 ) ) ;
#31526=ADVANCED_FACE ( 'NONE', ( #11529 ), #3149, .F. ) ;
#31531=ORIENTED_EDGE ( 'NONE', *, *, #34880, .F. ) ;
#31534=VERTEX_POINT ( 'NONE', #135 ) ;
#31539=ORIENTED_EDGE ( 'NONE', *, *, #17226, .T. ) ;
#31543=ORIENTED_EDGE ( 'NONE', *, *, #13301, .F. ) ;
#31544=EDGE_CURVE ( 'NONE', #7548, #24819, #32871, .T. ) ;
#31546=LINE ( 'NONE', #9497, #25916 ) ;
#31547=PLANE ( 'NONE',  #10680 ) ;
#31549=EDGE_CURVE ( 'NONE', #26511, #20630, #8667, .T. ) ;
#31551=DIRECTION ( 'NONE',  ( 1.000000000000000000, 0.000000000000000000, 0.000000000000000000 ) ) ;
#31553=DIRECTION ( 'NONE',  ( 1.000000000000000000, 0.000000000000000000, 0.000000000000000000 ) ) ;
#31554=CARTESIAN_POINT ( 'NONE',  ( -418.0000000000000000, -105.0000000000000142, 194.9999999999999716 ) ) ;
#31555=VECTOR ( 'NONE', #24165, 1000.000000000000000 ) ;
#31556=FACE_OUTER_BOUND ( 'NONE', #27239, .T. ) ;
#31557=ORIENTED_EDGE ( 'NONE', *, *, #5856, .F. ) ;
#31568=CARTESIAN_POINT ( 'NONE',  ( -500.0000000000000000, -105.0000000000000142, 187.0000000000000000 ) ) ;
#31569=EDGE_CURVE ( 'NONE', #26932, #23700, #10422, .T. ) ;
#31572=ORIENTED_EDGE ( 'NONE', *, *, #28692, .T. ) ;
#31573=DIRECTION ( 'NONE',  ( 0.000000000000000000, 1.000000000000000000, 1.224646799147353207E-16 ) ) ;
#31575=ADVANCED_FACE ( 'NONE', ( #666 ), #21667, .T. ) ;
#31576=ORIENTED_EDGE ( 'NONE', *, *, #373, .T. ) ;
#31578=ADVANCED_FACE ( 'NONE', ( #27710, #33226 ), #14386, .T. ) ;
#31579=ORIENTED_EDGE ( 'NONE', *, *, #5750, .F. ) ;
#31580=CARTESIAN_POINT ( 'NONE',  ( -361.0000000000000000, -125.0000000000000284, 112.0000000000000000 ) ) ;
#31582=ORIENTED_EDGE ( 'NONE', *, *, #23047, .T. ) ;
#31583=CARTESIAN_POINT ( 'NONE',  ( -442.0000000000000000, 104.9999999999999858, -162.9999999999999716 ) ) ;
#31585=DIRECTION ( 'NONE',  ( 0.000000000000000000, -1.000000000000000000, 0.000000000000000000 ) ) ;
#31588=ORIENTED_EDGE ( 'NONE', *, *, #21125, .F. ) ;
#31589=CARTESIAN_POINT ( 'NONE',  ( 11.99999999999999645, -55.00000000000002132, 155.0000000000000000 ) ) ;
#31590=DIRECTION ( 'NONE',  ( 0.000000000000000000, -0.000000000000000000, 1.000000000000000000 ) ) ;
#31593=CARTESIAN_POINT ( 'NONE',  ( -418.0000000000000000, -104.9999999999999716, -190.9999999999999716 ) ) ;
#31594=ORIENTED_EDGE ( 'NONE', *, *, #10363, .T. ) ;
#31597=LINE ( 'NONE', #25555, #32133 ) ;
#31600=ADVANCED_FACE ( 'NONE', ( #19197 ), #19021, .T. ) ;
#31602=DIRECTION ( 'NONE',  ( 0.000000000000000000, 0.000000000000000000, -1.000000000000000000 ) ) ;
#31603=FACE_OUTER_BOUND ( 'NONE', #21301, .T. ) ;
#31604=ORIENTED_EDGE ( 'NONE', *, *, #20665, .T. ) ;
#31607=DIRECTION ( 'NONE',  ( 0.000000000000000000, 0.000000000000000000, -1.000000000000000000 ) ) ;
#31608=LINE ( 'NONE', #1714, #25355 ) ;
#31612=EDGE_CURVE ( 'NONE', #6974, #28627, #2970, .T. ) ;
#31614=ORIENTED_EDGE ( 'NONE', *, *, #25788, .T. ) ;
#31616=DIRECTION ( 'NONE',  ( 0.000000000000000000, 1.000000000000000000, 5.145227585319922065E-49 ) ) ;
#31617=ORIENTED_EDGE ( 'NONE', *, *, #5078, .T. ) ;
#31620=VERTEX_POINT ( 'NONE', #6339 ) ;
#31625=DIRECTION ( 'NONE',  ( 0.000000000000000000, 1.000000000000000000, 5.053935297177146739E-49 ) ) ;
#31628=ORIENTED_EDGE ( 'NONE', *, *, #13498, .F. ) ;
#31630=VERTEX_POINT ( 'NONE', #17241 ) ;
#31631=( GEOMETRIC_REPRESENTATION_CONTEXT ( 3 ) GLOBAL_UNCERTAINTY_ASSIGNED_CONTEXT ( ( #20916 ) ) GLOBAL_UNIT_ASSIGNED_CONTEXT ( ( #5764, #16662, #26973 ) ) REPRESENTATION_CONTEXT ( 'NONE', 'WORKASPACE' ) );
#31632=LINE ( 'NONE', #18143, #19446 ) ;
#31633=CARTESIAN_POINT ( 'NONE',  ( -418.0000000000000568, -109.0000000000000142, -155.0000000000000000 ) ) ;
#31634=FACE_OUTER_BOUND ( 'NONE', #30782, .T. ) ;
#31636=FACE_OUTER_BOUND ( 'NONE', #4427, .T. ) ;
#31641=DIRECTION ( 'NONE',  ( 0.000000000000000000, 6.123233995736766036E-17, 1.000000000000000000 ) ) ;
#31642=ORIENTED_EDGE ( 'NONE', *, *, #20455, .F. ) ;
#31646=EDGE_CURVE ( 'NONE', #493, #22138, #17938, .T. ) ;
#31648=EDGE_CURVE ( 'NONE', #22205, #11568, #20075, .T. ) ;
#31655=EDGE_LOOP ( 'NONE', ( #13298, #20544, #14767, #20917 ) ) ;
#31664=ORIENTED_EDGE ( 'NONE', *, *, #32523, .T. ) ;
#31665=CARTESIAN_POINT ( 'NONE',  ( -361.0000000000000000, 134.9999999999999716, 112.0000000000000000 ) ) ;
#31670=VERTEX_POINT ( 'NONE', #3672 ) ;
#31672=ORIENTED_EDGE ( 'NONE', *, *, #26429, .T. ) ;
#31673=PLANE ( 'NONE',  #30115 ) ;
#31676=DIRECTION ( 'NONE',  ( -0.000000000000000000, -0.000000000000000000, 1.000000000000000000 ) ) ;
#31677=CIRCLE ( 'NONE', #16368, 2.000000000000001776 ) ;
#31679=ORIENTED_EDGE ( 'NONE', *, *, #22948, .T. ) ;
#31680=DIRECTION ( 'NONE',  ( 1.000000000000000000, 3.469446951953834515E-18, 0.000000000000000000 ) ) ;
#31681=( NAMED_UNIT ( * ) SI_UNIT ( $, .STERADIAN. ) SOLID_ANGLE_UNIT ( ) );
#31682=EDGE_CURVE ( 'NONE', #19198, #12986, #17588, .T. ) ;
#31685=DIRECTION ( 'NONE',  ( -1.000000000000000000, 0.000000000000000000, 0.000000000000000000 ) ) ;
#31686=VECTOR ( 'NONE', #32423, 1000.000000000000000 ) ;
#31691=CARTESIAN_POINT ( 'NONE',  ( -445.9999999999999432, -125.0000000000000000, 162.9999999999999716 ) ) ;
#31692=ADVANCED_FACE ( 'NONE', ( #14560 ), #28766, .T. ) ;
#31693=EDGE_CURVE ( 'NONE', #13074, #9444, #30305, .T. ) ;
#31695=VERTEX_POINT ( 'NONE', #4366 ) ;
#31696=ADVANCED_FACE ( 'NONE', ( #25744, #17420 ), #23093, .F. ) ;
#31697=EDGE_CURVE ( 'NONE', #26094, #26996, #28246, .T. ) ;
#31702=PLANE ( 'NONE',  #3418 ) ;
#31706=CARTESIAN_POINT ( 'NONE',  ( -442.0000000000000000, -125.0000000000000000, 190.9999999999999716 ) ) ;
#31717=CARTESIAN_POINT ( 'NONE',  ( -19.99999999999998934, -137.0000000000000000, 159.0000000000000000 ) ) ;
#31727=CARTESIAN_POINT ( 'NONE',  ( 11.99999999999999645, 144.9999999999999716, -186.9999999999999716 ) ) ;
#31736=LINE ( 'NONE', #1672, #953 ) ;
#31738=VERTEX_POINT ( 'NONE', #33935 ) ;
#31739=ADVANCED_FACE ( 'NONE', ( #25563 ), #1188, .T. ) ;
#31740=EDGE_CURVE ( 'NONE', #31336, #30159, #17756, .T. ) ;
#31742=EDGE_LOOP ( 'NONE', ( #16587, #23801, #33642, #7026, #27381, #823, #5941, #15267 ) ) ;
#31746=ORIENTED_EDGE ( 'NONE', *, *, #34140, .T. ) ;
#31753=LINE ( 'NONE', #7018, #33605 ) ;
#31755=VERTEX_POINT ( 'NONE', #33404 ) ;
#31759=ADVANCED_FACE ( 'NONE', ( #9026 ), #19895, .T. ) ;
#31761=CARTESIAN_POINT ( 'NONE',  ( -365.0000000000000000, 134.9999999999999716, 113.9999999999999716 ) ) ;
#31764=EDGE_LOOP ( 'NONE', ( #19719, #23541, #24961, #8287 ) ) ;
#31766=ADVANCED_FACE ( 'NONE', ( #7211 ), #34637, .F. ) ;
#31767=DIRECTION ( 'NONE',  ( 0.000000000000000000, -1.000000000000000000, 6.123233995736766036E-17 ) ) ;
#31768=DIRECTION ( 'NONE',  ( 0.000000000000000000, 2.309213040847544338E-50, 1.000000000000000000 ) ) ;
#31770=DIRECTION ( 'NONE',  ( 0.000000000000000000, 0.000000000000000000, -1.000000000000000000 ) ) ;
#31771=ADVANCED_FACE ( 'NONE', ( #7386 ), #18275, .F. ) ;
#31772=DIRECTION ( 'NONE',  ( 0.000000000000000000, -1.000000000000000000, 1.310824597558155437E-49 ) ) ;
#31773=DIRECTION ( 'NONE',  ( 0.000000000000000000, 1.000000000000000000, 0.000000000000000000 ) ) ;
#31775=CIRCLE ( 'NONE', #17049, 2.000000000000001776 ) ;
#31777=ORIENTED_EDGE ( 'NONE', *, *, #10574, .T. ) ;
#31780=DIRECTION ( 'NONE',  ( 1.000000000000000000, 0.000000000000000000, 0.000000000000000000 ) ) ;
#31785=CARTESIAN_POINT ( 'NONE',  ( -365.0000000000000000, 124.9999999999999432, 168.9999999999999716 ) ) ;
#31788=ORIENTED_EDGE ( 'NONE', *, *, #27270, .F. ) ;
#31792=DIRECTION ( 'NONE',  ( 1.000000000000000000, 0.000000000000000000, -0.000000000000000000 ) ) ;
#31793=VERTEX_POINT ( 'NONE', #12935 ) ;
#31796=CYLINDRICAL_SURFACE ( 'NONE', #25490, 7.999999999999979572 ) ;
#31798=CARTESIAN_POINT ( 'NONE',  ( -349.0000000000000000, -125.0000000000000284, 185.0000000000000000 ) ) ;
#31799=VERTEX_POINT ( 'NONE', #15426 ) ;
#31802=CARTESIAN_POINT ( 'NONE',  ( -20.00000000000007461, 144.9999999999999716, 187.0000000000000000 ) ) ;
#31806=PLANE ( 'NONE',  #23027 ) ;
#31809=CARTESIAN_POINT ( 'NONE',  ( -12.00000000000001066, -145.0000000000000000, 162.9999999999999716 ) ) ;
#31810=ORIENTED_EDGE ( 'NONE', *, *, #20729, .F. ) ;
#31814=EDGE_LOOP ( 'NONE', ( #11362, #12242, #24492, #30485 ) ) ;
#31818=DIRECTION ( 'NONE',  ( 0.000000000000000000, -1.000000000000000000, 5.145227585319922065E-49 ) ) ;
#31820=ORIENTED_EDGE ( 'NONE', *, *, #17772, .T. ) ;
#31821=CARTESIAN_POINT ( 'NONE',  ( -20.00000000000004619, -137.0000000000000000, -190.9999999999999716 ) ) ;
#31822=DIRECTION ( 'NONE',  ( 0.000000000000000000, -1.000000000000000000, 6.123233995736766036E-17 ) ) ;
#31825=ORIENTED_EDGE ( 'NONE', *, *, #25543, .T. ) ;
#31830=DIRECTION ( 'NONE',  ( 0.000000000000000000, 0.000000000000000000, 1.000000000000000000 ) ) ;
#31833=EDGE_CURVE ( 'NONE', #11932, #13361, #2457, .T. ) ;
#31836=CARTESIAN_POINT ( 'NONE',  ( -418.0000000000000000, 105.0000000000000142, 107.9999999999999858 ) ) ;
#31838=EDGE_LOOP ( 'NONE', ( #26967, #581, #22534, #17178 ) ) ;
#31845=VERTEX_POINT ( 'NONE', #13105 ) ;
#31847=CIRCLE ( 'NONE', #8054, 3.999999999999976019 ) ;
#31848=STYLED_ITEM('',(#35254),#23516);
#31850=DIRECTION ( 'NONE',  ( 0.000000000000000000, 1.000000000000000000, 1.224646799147353207E-16 ) ) ;
#31853=DIRECTION ( 'NONE',  ( 0.000000000000000000, 1.131431318426415506E-52, 1.000000000000000000 ) ) ;
#31857=CARTESIAN_POINT ( 'NONE',  ( -20.00000000000007461, -113.0000000000000000, -162.9999999999999716 ) ) ;
#31863=ORIENTED_EDGE ( 'NONE', *, *, #26150, .T. ) ;
#31868=EDGE_CURVE ( 'NONE', #18104, #22914, #26880, .T. ) ;
#31869=ORIENTED_EDGE ( 'NONE', *, *, #11762, .T. ) ;
#31876=LINE ( 'NONE', #15531, #8417 ) ;
#31878=ORIENTED_EDGE ( 'NONE', *, *, #17194, .F. ) ;
#31883=EDGE_CURVE ( 'NONE', #26418, #23829, #20117, .T. ) ;
#31887=ORIENTED_EDGE ( 'NONE', *, *, #29422, .F. ) ;
#31891=EDGE_CURVE ( 'NONE', #173, #8775, #9858, .T. ) ;
#31893=DIRECTION ( 'NONE',  ( 1.848892746611746419E-32, 6.842277657836020854E-49, -1.000000000000000000 ) ) ;
#31894=EDGE_CURVE ( 'NONE', #13396, #26094, #14433, .T. ) ;
#31897=CARTESIAN_POINT ( 'NONE',  ( -414.0000000000000568, 105.0000000000000000, 132.0000000000000000 ) ) ;
#31904=FACE_OUTER_BOUND ( 'NONE', #11297, .T. ) ;
#31909=DIRECTION ( 'NONE',  ( 0.000000000000000000, -1.000000000000000000, 2.309213040847544338E-50 ) ) ;
#31915=ORIENTED_EDGE ( 'NONE', *, *, #7138, .T. ) ;
#31917=PLANE ( 'NONE',  #18490 ) ;
#31919=( GEOMETRIC_REPRESENTATION_CONTEXT ( 3 ) GLOBAL_UNCERTAINTY_ASSIGNED_CONTEXT ( ( #6746 ) ) GLOBAL_UNIT_ASSIGNED_CONTEXT ( ( #22080, #6211, #5680 ) ) REPRESENTATION_CONTEXT ( 'NONE', 'WORKASPACE' ) );
#31920=DIRECTION ( 'NONE',  ( 0.000000000000000000, -0.000000000000000000, -1.000000000000000000 ) ) ;
#31922=DIRECTION ( 'NONE',  ( 0.000000000000000000, -1.310824597558155437E-49, -1.000000000000000000 ) ) ;
#31923=EDGE_LOOP ( 'NONE', ( #13997, #33859, #15281, #10973 ) ) ;
#31924=ORIENTED_EDGE ( 'NONE', *, *, #1055, .T. ) ;
#31927=LINE ( 'NONE', #15581, #31495 ) ;
#31928=VECTOR ( 'NONE', #2271, 1000.000000000000000 ) ;
#31929=CARTESIAN_POINT ( 'NONE',  ( -499.9999999999999432, -137.0000000000000000, -194.9999999999999716 ) ) ;
#31932=DIRECTION ( 'NONE',  ( 0.000000000000000000, -1.000000000000000000, -5.053935297177146739E-49 ) ) ;
#31935=CARTESIAN_POINT ( 'NONE',  ( -500.0000000000000000, -137.0000000000000000, 162.9999999999999716 ) ) ;
#31936=EDGE_CURVE ( 'NONE', #30882, #24475, #23423, .T. ) ;
#31937=ADVANCED_FACE ( 'NONE', ( #91 ), #3105, .T. ) ;
#31939=ORIENTED_EDGE ( 'NONE', *, *, #20624, .T. ) ;
#31940=DIRECTION ( 'NONE',  ( 0.000000000000000000, 0.000000000000000000, -1.000000000000000000 ) ) ;
#31941=CARTESIAN_POINT ( 'NONE',  ( -365.0000000000000000, -119.0000000000000000, 128.0000000000000000 ) ) ;
#31944=DIRECTION ( 'NONE',  ( 1.000000000000000000, 0.000000000000000000, 0.000000000000000000 ) ) ;
#31946=DIRECTION ( 'NONE',  ( -3.469446951953832974E-18, -1.000000000000000000, 7.888609052210118054E-31 ) ) ;
#31948=DIRECTION ( 'NONE',  ( -0.000000000000000000, 1.000000000000000000, -0.000000000000000000 ) ) ;
#31957=FACE_OUTER_BOUND ( 'NONE', #26133, .T. ) ;
#31959=EDGE_CURVE ( 'NONE', #12542, #8355, #621, .T. ) ;
#31961=EDGE_CURVE ( 'NONE', #30502, #6872, #5760, .T. ) ;
#31964=ORIENTED_EDGE ( 'NONE', *, *, #33516, .F. ) ;
#31965=CARTESIAN_POINT ( 'NONE',  ( -361.0000000000000000, 134.9999999999999716, 126.0000000000000000 ) ) ;
#31966=ORIENTED_EDGE ( 'NONE', *, *, #19808, .T. ) ;
#31967=CARTESIAN_POINT ( 'NONE',  ( -70.00000000000000000, 4.559999999999908127, -172.9900000000000091 ) ) ;
#31968=EDGE_CURVE ( 'NONE', #9649, #10216, #29197, .T. ) ;
#31970=DIRECTION ( 'NONE',  ( -0.000000000000000000, 1.000000000000000000, -0.000000000000000000 ) ) ;
#31971=DIRECTION ( 'NONE',  ( 0.000000000000000000, 1.000000000000000000, 1.224646799147353207E-16 ) ) ;
#31973=ORIENTED_EDGE ( 'NONE', *, *, #817, .T. ) ;
#31974=ORIENTED_EDGE ( 'NONE', *, *, #17782, .T. ) ;
#31975=ORIENTED_EDGE ( 'NONE', *, *, #33232, .T. ) ;
#31980=DIRECTION ( 'NONE',  ( 0.000000000000000000, 0.000000000000000000, -1.000000000000000000 ) ) ;
#31985=CIRCLE ( 'NONE', #16667, 4.000000000000003553 ) ;
#31987=VERTEX_POINT ( 'NONE', #24988 ) ;
#31990=FACE_OUTER_BOUND ( 'NONE', #4881, .T. ) ;
#31991=ORIENTED_EDGE ( 'NONE', *, *, #27408, .F. ) ;
#31993=ORIENTED_EDGE ( 'NONE', *, *, #1199, .T. ) ;
#31996=AXIS2_PLACEMENT_3D ( 'NONE', #23214, #17545, #31219 ) ;
#31997=ORIENTED_EDGE ( 'NONE', *, *, #31693, .F. ) ;
#32004=ADVANCED_FACE ( 'NONE', ( #30340 ), #2925, .F. ) ;
#32005=VERTEX_POINT ( 'NONE', #11483 ) ;
#32006=AXIS2_PLACEMENT_3D ( 'NONE', #2233, #21102, #9896 ) ;
#32012=CARTESIAN_POINT ( 'NONE',  ( -12.00000000000001066, -145.0000000000000000, -190.9999999999999432 ) ) ;
#32015=VERTEX_POINT ( 'NONE', #5942 ) ;
#32019=CARTESIAN_POINT ( 'NONE',  ( -19.99999999999998934, 134.9999999999999432, -186.9999999999999716 ) ) ;
#32022=ORIENTED_EDGE ( 'NONE', *, *, #9414, .F. ) ;
#32024=ORIENTED_EDGE ( 'NONE', *, *, #18712, .T. ) ;
#32026=LINE ( 'NONE', #27047, #32460 ) ;
#32029=DIRECTION ( 'NONE',  ( 0.000000000000000000, 7.888609052210118054E-31, 1.000000000000000000 ) ) ;
#32043=EDGE_CURVE ( 'NONE', #26108, #23877, #2579, .T. ) ;
#32045=EDGE_CURVE ( 'NONE', #20392, #26810, #12019, .T. ) ;
#32046=EDGE_LOOP ( 'NONE', ( #19945, #26734, #3788, #2410 ) ) ;
#32050=LINE ( 'NONE', #16074, #33588 ) ;
#32061=DIRECTION ( 'NONE',  ( 0.000000000000000000, 0.000000000000000000, -1.000000000000000000 ) ) ;
#32065=DIRECTION ( 'NONE',  ( -1.000000000000000000, 0.000000000000000000, 0.000000000000000000 ) ) ;
#32070=ORIENTED_EDGE ( 'NONE', *, *, #1136, .T. ) ;
#32071=CYLINDRICAL_SURFACE ( 'NONE', #5536, 4.750000000000004441 ) ;
#32072=FACE_OUTER_BOUND ( 'NONE', #24327, .T. ) ;
#32073=VECTOR ( 'NONE', #3425, 1000.000000000000000 ) ;
#32074=AXIS2_PLACEMENT_3D ( 'NONE', #14452, #33117, #390 ) ;
#32076=CARTESIAN_POINT ( 'NONE',  ( -442.0000000000000000, 124.9999999999999432, -162.9999999999999716 ) ) ;
#32080=DIRECTION ( 'NONE',  ( -0.000000000000000000, 0.000000000000000000, 1.000000000000000000 ) ) ;
#32082=VECTOR ( 'NONE', #413, 1000.000000000000000 ) ;
#32087=LINE ( 'NONE', #29601, #5246 ) ;
#32088=CARTESIAN_POINT ( 'NONE',  ( -349.0000000000000000, 134.9999999999999716, 130.0000000000000000 ) ) ;
#32089=AXIS2_PLACEMENT_3D ( 'NONE', #16722, #30588, #14041 ) ;
#32092=ORIENTED_EDGE ( 'NONE', *, *, #31833, .F. ) ;
#32093=CARTESIAN_POINT ( 'NONE',  ( -418.0000000000000000, -104.9999999999999716, -190.9999999999999716 ) ) ;
#32096=AXIS2_PLACEMENT_3D ( 'NONE', #386, #11240, #25097 ) ;
#32100=EDGE_LOOP ( 'NONE', ( #34832, #30735, #28281, #15593 ) ) ;
#32103=EDGE_CURVE ( 'NONE', #25412, #30341, #11850, .T. ) ;
#32109=VERTEX_POINT ( 'NONE', #33897 ) ;
#32110=CIRCLE ( 'NONE', #18504, 4.000000000000003553 ) ;
#32112=DIRECTION ( 'NONE',  ( 1.000000000000000000, 0.000000000000000000, 0.000000000000000000 ) ) ;
#32113=CARTESIAN_POINT ( 'NONE',  ( -12.00000000000001066, -145.0000000000000000, -158.9999999999999716 ) ) ;
#32116=LINE ( 'NONE', #31761, #22227 ) ;
#32118=CARTESIAN_POINT ( 'NONE',  ( -361.0000000000000000, -125.0000000000000284, 168.9999999999999716 ) ) ;
#32120=VERTEX_POINT ( 'NONE', #20028 ) ;
#32122=DIRECTION ( 'NONE',  ( 0.000000000000000000, 0.000000000000000000, -1.000000000000000000 ) ) ;
#32124=ORIENTED_EDGE ( 'NONE', *, *, #13583, .T. ) ;
#32126=EDGE_LOOP ( 'NONE', ( #27334, #7212, #9027, #9061 ) ) ;
#32133=VECTOR ( 'NONE', #6685, 1000.000000000000000 ) ;
#32134=LINE ( 'NONE', #18634, #10269 ) ;
#32144=ORIENTED_EDGE ( 'NONE', *, *, #5963, .T. ) ;
#32146=EDGE_CURVE ( 'NONE', #29515, #13784, #27843, .T. ) ;
#32152=CARTESIAN_POINT ( 'NONE',  ( 15.99999999999998579, 136.9999999999999716, -155.0000000000000000 ) ) ;
#32153=CIRCLE ( 'NONE', #12861, 3.999999999999976019 ) ;
#32157=VERTEX_POINT ( 'NONE', #9339 ) ;
#32159=DIRECTION ( 'NONE',  ( 0.000000000000000000, 0.000000000000000000, 1.000000000000000000 ) ) ;
#32168=EDGE_LOOP ( 'NONE', ( #16888, #27815, #16157, #14316 ) ) ;
#32173=CARTESIAN_POINT ( 'NONE',  ( -410.0000000000000568, -137.0000000000000000, 154.9999999999999716 ) ) ;
#32174=EDGE_LOOP ( 'NONE', ( #33805, #18628, #14138, #8721, #26088, #11125, #20167, #31915, #21497, #32741, #11497, #8329, #12063, #26427, #7518, #27323 ) ) ;
#32175=EDGE_CURVE ( 'NONE', #29708, #890, #14868, .T. ) ;
#32176=EDGE_CURVE ( 'NONE', #19981, #11239, #7579, .T. ) ;
#32177=CARTESIAN_POINT ( 'NONE',  ( -20.00000000000004619, -134.9999999999999716, -162.9999999999999432 ) ) ;
#32179=DIRECTION ( 'NONE',  ( -0.000000000000000000, -1.000000000000000000, -0.000000000000000000 ) ) ;
#32180=CARTESIAN_POINT ( 'NONE',  ( -12.00000000000001066, -145.0000000000000000, -162.9999999999999432 ) ) ;
#32181=AXIS2_PLACEMENT_3D ( 'NONE', #28537, #6805, #20358 ) ;
#32182=EDGE_LOOP ( 'NONE', ( #20512, #8252, #33344, #8924 ) ) ;
#32183=CARTESIAN_POINT ( 'NONE',  ( -15.99999999999998579, -32.99999999999997158, -175.0000000000000000 ) ) ;
#32184=DIRECTION ( 'NONE',  ( 1.000000000000000000, 0.000000000000000000, 0.000000000000000000 ) ) ;
#32186=VECTOR ( 'NONE', #19890, 1000.000000000000000 ) ;
#32187=EDGE_LOOP ( 'NONE', ( #30519, #12037, #25503, #7722 ) ) ;
#32190=EDGE_CURVE ( 'NONE', #21633, #7246, #17715, .T. ) ;
#32193=CARTESIAN_POINT ( 'NONE',  ( -355.0000000000000000, -117.0000000000000000, 126.0000000000000000 ) ) ;
#32195=VECTOR ( 'NONE', #29602, 1000.000000000000000 ) ;
#32196=DIRECTION ( 'NONE',  ( 1.000000000000000000, 0.000000000000000000, -1.848892746611746966E-32 ) ) ;
#32201=CARTESIAN_POINT ( 'NONE',  ( -12.00000000000001066, -109.0000000000000142, 174.9999999999999432 ) ) ;
#32204=DIRECTION ( 'NONE',  ( 0.000000000000000000, 0.000000000000000000, 1.000000000000000000 ) ) ;
#32206=ORIENTED_EDGE ( 'NONE', *, *, #20455, .T. ) ;
#32215=EDGE_CURVE ( 'NONE', #31108, #32651, #26399, .T. ) ;
#32216=CARTESIAN_POINT ( 'NONE',  ( 11.99999999999999645, 134.9999999999998863, 155.0000000000000000 ) ) ;
#32221=EDGE_CURVE ( 'NONE', #5645, #28398, #4185, .T. ) ;
#32229=STYLED_ITEM('',(#35254),#21945);
#32231=VECTOR ( 'NONE', #18865, 1000.000000000000000 ) ;
#32238=VERTEX_POINT ( 'NONE', #23381 ) ;
#32239=CARTESIAN_POINT ( 'NONE',  ( 19.99999999999998934, 4.559999999999908127, -172.9900000000000091 ) ) ;
#32242=AXIS2_PLACEMENT_3D ( 'NONE', #4514, #27430, #7365 ) ;
#32245=CARTESIAN_POINT ( 'NONE',  ( 12.00000000000001066, -134.9999999999999716, 194.9999999999999716 ) ) ;
#32246=CARTESIAN_POINT ( 'NONE',  ( -365.0000000000000000, -125.0000000000000284, 113.9999999999999858 ) ) ;
#32250=VERTEX_POINT ( 'NONE', #28898 ) ;
#32252=FACE_OUTER_BOUND ( 'NONE', #29043, .T. ) ;
#32253=VECTOR ( 'NONE', #24483, 1000.000000000000000 ) ;
#32256=EDGE_CURVE ( 'NONE', #11246, #15089, #3068, .T. ) ;
#32259=FACE_OUTER_BOUND ( 'NONE', #27577, .T. ) ;
#32265=FACE_OUTER_BOUND ( 'NONE', #14597, .T. ) ;
#32270=CARTESIAN_POINT ( 'NONE',  ( -70.00000000000000000, 4.559999999999909015, 177.7400000000000091 ) ) ;
#32271=ORIENTED_EDGE ( 'NONE', *, *, #4080, .T. ) ;
#32275=CARTESIAN_POINT ( 'NONE',  ( -345.0000000000000000, -135.0000000000000000, 126.0000000000000000 ) ) ;
#32280=FACE_OUTER_BOUND ( 'NONE', #24751, .T. ) ;
#32283=CARTESIAN_POINT ( 'NONE',  ( -365.0000000000000000, 130.9999999999999716, 128.0000000000000000 ) ) ;
#32285=EDGE_CURVE ( 'NONE', #16248, #10505, #5026, .T. ) ;
#32286=FACE_OUTER_BOUND ( 'NONE', #21073, .T. ) ;
#32287=CARTESIAN_POINT ( 'NONE',  ( 11.99999999999999645, 144.9999999999999716, 187.0000000000000000 ) ) ;
#32288=ORIENTED_EDGE ( 'NONE', *, *, #31682, .T. ) ;
#32289=CARTESIAN_POINT ( 'NONE',  ( 19.99999999999998934, -145.0000000000000000, -186.9999999999999716 ) ) ;
#32291=VECTOR ( 'NONE', #9457, 1000.000000000000000 ) ;
#32295=DIRECTION ( 'NONE',  ( 1.232595164407830946E-32, 3.421138828918010427E-49, -1.000000000000000000 ) ) ;
#32299=DIRECTION ( 'NONE',  ( 1.000000000000000000, 0.000000000000000000, 0.000000000000000000 ) ) ;
#32300=ORIENTED_EDGE ( 'NONE', *, *, #5379, .F. ) ;
#32301=VECTOR ( 'NONE', #23315, 1000.000000000000000 ) ;
#32302=VECTOR ( 'NONE', #21869, 1000.000000000000000 ) ;
#32305=LINE ( 'NONE', #7745, #23350 ) ;
#32308=CIRCLE ( 'NONE', #22081, 2.000000000000001776 ) ;
#32312=VERTEX_POINT ( 'NONE', #17895 ) ;
#32313=CIRCLE ( 'NONE', #9617, 3.999999999999976019 ) ;
#32319=DIRECTION ( 'NONE',  ( -1.232595164407830946E-32, -3.421138828918010427E-49, 1.000000000000000000 ) ) ;
#32320=VECTOR ( 'NONE', #34298, 1000.000000000000000 ) ;
#32323=VERTEX_POINT ( 'NONE', #10030 ) ;
#32324=ORIENTED_EDGE ( 'NONE', *, *, #15479, .T. ) ;
#32326=ORIENTED_EDGE ( 'NONE', *, *, #33541, .F. ) ;
#32329=EDGE_CURVE ( 'NONE', #173, #9401, #15922, .T. ) ;
#32340=CARTESIAN_POINT ( 'NONE',  ( -12.00000000000001243, 144.9999999999999147, 194.9999999999999716 ) ) ;
#32342=ORIENTED_EDGE ( 'NONE', *, *, #6255, .T. ) ;
#32344=EDGE_CURVE ( 'NONE', #20271, #33601, #34595, .T. ) ;
#32345=PLANE ( 'NONE',  #18388 ) ;
#32348=ADVANCED_FACE ( 'NONE', ( #10206 ), #29253, .F. ) ;
#32357=ORIENTED_EDGE ( 'NONE', *, *, #14858, .T. ) ;
#32362=CYLINDRICAL_SURFACE ( 'NONE', #27171, 2.000000000000001776 ) ;
#32363=AXIS2_PLACEMENT_3D ( 'NONE', #25104, #14806, #739 ) ;
#32367=VERTEX_POINT ( 'NONE', #15742 ) ;
#32371=EDGE_LOOP ( 'NONE', ( #15335, #30363, #14301, #33262 ) ) ;
#32373=CARTESIAN_POINT ( 'NONE',  ( -12.00000000000001066, 140.9999999999999716, -155.0000000000000000 ) ) ;
#32377=CARTESIAN_POINT ( 'NONE',  ( -418.0000000000000000, 105.0000000000000142, 107.9999999999999858 ) ) ;
#32378=ORIENTED_EDGE ( 'NONE', *, *, #13517, .F. ) ;
#32379=CIRCLE ( 'NONE', #11936, 7.999999999999979572 ) ;
#32382=EDGE_CURVE ( 'NONE', #14594, #2181, #27627, .T. ) ;
#32383=EDGE_CURVE ( 'NONE', #29500, #5880, #235, .T. ) ;
#32386=CARTESIAN_POINT ( 'NONE',  ( -12.00000000000001066, -141.0000000000000000, -154.9999999999999716 ) ) ;
#32387=CARTESIAN_POINT ( 'NONE',  ( 11.99999999999995559, -134.9999999999999716, -154.9999999999999716 ) ) ;
#32400=EDGE_CURVE ( 'NONE', #11811, #17161, #19461, .T. ) ;
#32401=ORIENTED_EDGE ( 'NONE', *, *, #16453, .T. ) ;
#32404=DIRECTION ( 'NONE',  ( 0.000000000000000000, -1.000000000000000000, 0.000000000000000000 ) ) ;
#32407=CARTESIAN_POINT ( 'NONE',  ( -442.0000000000000000, -125.0000000000000000, -109.9999999999999574 ) ) ;
#32412=AXIS2_PLACEMENT_3D ( 'NONE', #10277, #20616, #31980 ) ;
#32414=VERTEX_POINT ( 'NONE', #24417 ) ;
#32417=FACE_BOUND ( 'NONE', #31742, .T. ) ;
#32418=DIRECTION ( 'NONE',  ( 0.000000000000000000, -1.131431318426415506E-52, -1.000000000000000000 ) ) ;
#32421=CARTESIAN_POINT ( 'NONE',  ( -414.0000000000000568, 113.0000000000000000, -175.0000000000000000 ) ) ;
#32423=DIRECTION ( 'NONE',  ( 1.000000000000000000, 3.040835319149746090E-31, 1.232595164407830946E-32 ) ) ;
#32429=CARTESIAN_POINT ( 'NONE',  ( -500.0000000000000000, -113.0000000000000000, 187.0000000000000000 ) ) ;
#32431=CARTESIAN_POINT ( 'NONE',  ( 19.99999999999998934, 75.55999999999990280, 172.9900000000000091 ) ) ;
#32433=DIRECTION ( 'NONE',  ( -3.040835319149746528E-31, -1.000000000000000000, 0.000000000000000000 ) ) ;
#32437=PLANE ( 'NONE',  #20042 ) ;
#32438=AXIS2_PLACEMENT_3D ( 'NONE', #10786, #13109, #23941 ) ;
#32439=ORIENTED_EDGE ( 'NONE', *, *, #8934, .T. ) ;
#32445=ORIENTED_EDGE ( 'NONE', *, *, #12230, .T. ) ;
#32446=VECTOR ( 'NONE', #7727, 1000.000000000000000 ) ;
#32448=AXIS2_PLACEMENT_3D ( 'NONE', #18431, #29273, #18779 ) ;
#32449=DIRECTION ( 'NONE',  ( 0.000000000000000000, 1.000000000000000000, 5.053935297177146739E-49 ) ) ;
#32450=CARTESIAN_POINT ( 'NONE',  ( -410.0000000000000568, -112.9999999999999858, -174.9999999999999716 ) ) ;
#32451=ORIENTED_EDGE ( 'NONE', *, *, #5810, .F. ) ;
#32453=CARTESIAN_POINT ( 'NONE',  ( -441.9999999999999432, 105.0000000000000000, 135.9999999999999716 ) ) ;
#32454=EDGE_CURVE ( 'NONE', #28176, #10430, #27455, .T. ) ;
#32458=EDGE_LOOP ( 'NONE', ( #23324, #27380 ) ) ;
#32460=VECTOR ( 'NONE', #2481, 1000.000000000000000 ) ;
#32462=ORIENTED_EDGE ( 'NONE', *, *, #29202, .T. ) ;
#32463=VECTOR ( 'NONE', #12113, 1000.000000000000000 ) ;
#32467=DIRECTION ( 'NONE',  ( 0.000000000000000000, 1.000000000000000000, -1.310824597558155437E-49 ) ) ;
#32468=DIRECTION ( 'NONE',  ( 0.000000000000000000, -1.000000000000000000, -2.465190328815662439E-32 ) ) ;
#32470=EDGE_LOOP ( 'NONE', ( #7362, #14559, #12406, #31964, #7541, #20333, #34295, #27918 ) ) ;
#32473=EDGE_CURVE ( 'NONE', #32015, #31695, #5900, .T. ) ;
#32476=AXIS2_PLACEMENT_3D ( 'NONE', #19918, #873, #20444 ) ;
#32480=EDGE_CURVE ( 'NONE', #9466, #6872, #24779, .T. ) ;
#32490=VERTEX_POINT ( 'NONE', #3244 ) ;
#32491=VECTOR ( 'NONE', #7082, 1000.000000000000000 ) ;
#32493=DIRECTION ( 'NONE',  ( 0.000000000000000000, 0.000000000000000000, -1.000000000000000000 ) ) ;
#32494=DIRECTION ( 'NONE',  ( -1.000000000000000000, -3.040835319149746090E-31, -1.232595164407830946E-32 ) ) ;
#32496=VERTEX_POINT ( 'NONE', #30297 ) ;
#32499=CARTESIAN_POINT ( 'NONE',  ( -15.99999999999998579, 4.559999999999908127, -172.9900000000000091 ) ) ;
#32501=CARTESIAN_POINT ( 'NONE',  ( -418.0000000000000000, -105.0000000000000142, 162.9999999999999716 ) ) ;
#32503=CARTESIAN_POINT ( 'NONE',  ( -349.0000000000000000, -125.0000000000000284, 183.0000000000000000 ) ) ;
#32504=CARTESIAN_POINT ( 'NONE',  ( 15.99999999999998579, -137.0000000000000000, 174.9999999999999432 ) ) ;
#32507=ORIENTED_EDGE ( 'NONE', *, *, #17340, .T. ) ;
#32508=DIRECTION ( 'NONE',  ( -1.000000000000000000, 0.000000000000000000, 0.000000000000000000 ) ) ;
#32509=CARTESIAN_POINT ( 'NONE',  ( -365.0000000000000000, -117.0000000000000000, 126.0000000000000000 ) ) ;
#32511=VERTEX_POINT ( 'NONE', #28128 ) ;
#32514=CARTESIAN_POINT ( 'NONE',  ( -418.0000000000000000, 105.0000000000000142, -175.0000000000000000 ) ) ;
#32516=CARTESIAN_POINT ( 'NONE',  ( -441.9999999999999432, -105.0000000000000142, 190.9999999999999716 ) ) ;
#32518=EDGE_LOOP ( 'NONE', ( #2980, #14413, #13320, #26988, #24785, #24184, #33387, #17564 ) ) ;
#32519=ADVANCED_FACE ( 'NONE', ( #5545 ), #27274, .T. ) ;
#32520=DIRECTION ( 'NONE',  ( 0.000000000000000000, -1.224646799147353207E-16, 1.000000000000000000 ) ) ;
#32521=DIRECTION ( 'NONE',  ( -0.000000000000000000, -0.000000000000000000, -1.000000000000000000 ) ) ;
#32522=DIRECTION ( 'NONE',  ( -1.000000000000000000, 0.000000000000000000, 0.000000000000000000 ) ) ;
#32523=EDGE_CURVE ( 'NONE', #30447, #18562, #6245, .T. ) ;
#32526=ORIENTED_EDGE ( 'NONE', *, *, #8099, .T. ) ;
#32529=CARTESIAN_POINT ( 'NONE',  ( -355.0000000000000000, 130.9999999999999716, 111.9999999999999858 ) ) ;
#32530=ADVANCED_FACE ( 'NONE', ( #16979 ), #4104, .T. ) ;
#32535=LINE ( 'NONE', #10675, #15047 ) ;
#32540=CIRCLE ( 'NONE', #20073, 7.999999999999979572 ) ;
#32542=DIRECTION ( 'NONE',  ( 0.000000000000000000, 1.131431318426415506E-52, 1.000000000000000000 ) ) ;
#32545=CARTESIAN_POINT ( 'NONE',  ( -70.00000000000000000, 4.559999999999908127, -177.7400000000000091 ) ) ;
#32549=ORIENTED_EDGE ( 'NONE', *, *, #15853, .T. ) ;
#32552=ORIENTED_EDGE ( 'NONE', *, *, #26914, .T. ) ;
#32555=CARTESIAN_POINT ( 'NONE',  ( -355.0000000000000000, 130.9999999999999716, 126.0000000000000000 ) ) ;
#32564=VECTOR ( 'NONE', #34589, 1000.000000000000000 ) ;
#32566=DIRECTION ( 'NONE',  ( 1.000000000000000000, 0.000000000000000000, 0.000000000000000000 ) ) ;
#32571=ADVANCED_FACE ( 'NONE', ( #25123 ), #33142, .T. ) ;
#32573=ORIENTED_EDGE ( 'NONE', *, *, #33140, .T. ) ;
#32576=EDGE_CURVE ( 'NONE', #27211, #26816, #14994, .T. ) ;
#32578=ADVANCED_FACE ( 'NONE', ( #25480 ), #22476, .F. ) ;
#32582=CARTESIAN_POINT ( 'NONE',  ( -19.99999999999998934, -32.99999999999997158, -154.9999999999999716 ) ) ;
#32584=CARTESIAN_POINT ( 'NONE',  ( -19.99999999999996092, 125.0000000000000568, 162.9999999999999716 ) ) ;
#32586=EDGE_LOOP ( 'NONE', ( #13841, #21128, #2366, #10684, #25057, #8930, #3868, #29525 ) ) ;
#32589=CARTESIAN_POINT ( 'NONE',  ( 19.99999999999998224, 134.9999999999998863, 162.9999999999999716 ) ) ;
#32591=DIRECTION ( 'NONE',  ( -3.469446951953832974E-18, -1.000000000000000000, -7.888609052210116302E-31 ) ) ;
#32592=DIRECTION ( 'NONE',  ( -0.000000000000000000, 1.000000000000000000, -0.000000000000000000 ) ) ;
#32593=EDGE_CURVE ( 'NONE', #30730, #13606, #33324, .T. ) ;
#32595=VERTEX_POINT ( 'NONE', #30660 ) ;
#32596=DIRECTION ( 'NONE',  ( 2.736911063134582149E-48, -7.888609052210118054E-31, -1.000000000000000000 ) ) ;
#32601=DIRECTION ( 'NONE',  ( 0.000000000000000000, 0.000000000000000000, -1.000000000000000000 ) ) ;
#32602=CARTESIAN_POINT ( 'NONE',  ( -499.9999999999999432, 136.9999999999999432, -187.0000000000000000 ) ) ;
#32604=DIRECTION ( 'NONE',  ( 0.000000000000000000, -1.131431318426415506E-52, -1.000000000000000000 ) ) ;
#32607=ADVANCED_FACE ( 'NONE', ( #6783 ), #33494, .T. ) ;
#32611=DIRECTION ( 'NONE',  ( -1.000000000000000000, 0.000000000000000000, -0.000000000000000000 ) ) ;
#32614=VECTOR ( 'NONE', #13939, 1000.000000000000000 ) ;
#32616=ORIENTED_EDGE ( 'NONE', *, *, #10376, .T. ) ;
#32618=EDGE_CURVE ( 'NONE', #4151, #4421, #1283, .T. ) ;
#32619=ORIENTED_EDGE ( 'NONE', *, *, #4485, .T. ) ;
#32620=CARTESIAN_POINT ( 'NONE',  ( -442.0000000000000000, 124.9999999999999574, -187.0000000000000000 ) ) ;
#32628=CARTESIAN_POINT ( 'NONE',  ( -361.0000000000000000, -125.0000000000000284, 126.0000000000000000 ) ) ;
#32631=DIRECTION ( 'NONE',  ( 1.000000000000000000, 3.040835319149746528E-31, 1.232595164407830946E-32 ) ) ;
#32636=CARTESIAN_POINT ( 'NONE',  ( 11.99999999999999645, 112.9999999999999574, -155.0000000000000000 ) ) ;
#32642=VECTOR ( 'NONE', #4505, 1000.000000000000000 ) ;
#32645=CARTESIAN_POINT ( 'NONE',  ( -19.99999999999998934, -145.0000000000000000, -162.9999999999999432 ) ) ;
#32649=ADVANCED_FACE ( 'NONE', ( #28679 ), #23690, .T. ) ;
#32651=VERTEX_POINT ( 'NONE', #4804 ) ;
#32654=( LENGTH_UNIT ( ) NAMED_UNIT ( * ) SI_UNIT ( .MILLI., .METRE. ) );
#32656=AXIS2_PLACEMENT_3D ( 'NONE', #14491, #6798, #3947 ) ;
#32658=ORIENTED_EDGE ( 'NONE', *, *, #21255, .T. ) ;
#32660=EDGE_CURVE ( 'NONE', #25172, #19146, #13886, .T. ) ;
#32663=ORIENTED_EDGE ( 'NONE', *, *, #28807, .T. ) ;
#32664=ORIENTED_EDGE ( 'NONE', *, *, #2470, .T. ) ;
#32665=EDGE_LOOP ( 'NONE', ( #9726, #1295, #2029, #13963, #7112, #10009, #5811, #32693 ) ) ;
#32668=VERTEX_POINT ( 'NONE', #18196 ) ;
#32671=ORIENTED_EDGE ( 'NONE', *, *, #7106, .T. ) ;
#32673=CARTESIAN_POINT ( 'NONE',  ( 11.99999999999999645, -145.0000000000000000, 190.9999999999999716 ) ) ;
#32674=AXIS2_PLACEMENT_3D ( 'NONE', #3694, #6714, #17610 ) ;
#32678=VERTEX_POINT ( 'NONE', #15342 ) ;
#32680=DIRECTION ( 'NONE',  ( 0.000000000000000000, 0.000000000000000000, -1.000000000000000000 ) ) ;
#32686=CARTESIAN_POINT ( 'NONE',  ( -418.0000000000000000, 105.0000000000000142, 155.0000000000000000 ) ) ;
#32687=DIRECTION ( 'NONE',  ( -0.000000000000000000, 1.000000000000000000, -0.000000000000000000 ) ) ;
#32688=ORIENTED_EDGE ( 'NONE', *, *, #14532, .T. ) ;
#32692=CARTESIAN_POINT ( 'NONE',  ( -19.99999999999998934, 134.9999999999998863, 162.9999999999999716 ) ) ;
#32693=ORIENTED_EDGE ( 'NONE', *, *, #30328, .T. ) ;
#32694=EDGE_CURVE ( 'NONE', #15311, #423, #4617, .T. ) ;
#32695=PLANE ( 'NONE',  #8105 ) ;
#32697=EDGE_CURVE ( 'NONE', #6316, #20279, #10162, .T. ) ;
#32704=DIRECTION ( 'NONE',  ( 0.000000000000000000, 0.000000000000000000, -1.000000000000000000 ) ) ;
#32706=DIRECTION ( 'NONE',  ( 0.000000000000000000, 0.000000000000000000, 1.000000000000000000 ) ) ;
#32707=LINE ( 'NONE', #26668, #16233 ) ;
#32708=LINE ( 'NONE', #27194, #17208 ) ;
#32709=EDGE_LOOP ( 'NONE', ( #5308, #22177, #26276, #3636, #26100, #8668, #9660, #14932 ) ) ;
#32711=VERTEX_POINT ( 'NONE', #26529 ) ;
#32713=CARTESIAN_POINT ( 'NONE',  ( -442.0000000000000000, 105.0000000000000142, 187.0000000000000000 ) ) ;
#32714=ORIENTED_EDGE ( 'NONE', *, *, #26617, .F. ) ;
#32715=AXIS2_PLACEMENT_3D ( 'NONE', #3440, #27658, #25157 ) ;
#32717=CARTESIAN_POINT ( 'NONE',  ( -442.0000000000000000, -104.9999999999999858, -155.0000000000000000 ) ) ;
#32720=ORIENTED_EDGE ( 'NONE', *, *, #25061, .T. ) ;
#32724=VECTOR ( 'NONE', #34018, 1000.000000000000000 ) ;
#32726=AXIS2_PLACEMENT_3D ( 'NONE', #17736, #1170, #31415 ) ;
#32728=ORIENTED_EDGE ( 'NONE', *, *, #31646, .F. ) ;
#32731=VERTEX_POINT ( 'NONE', #29020 ) ;
#32735=ORIENTED_EDGE ( 'NONE', *, *, #27209, .T. ) ;
#32738=FACE_OUTER_BOUND ( 'NONE', #23915, .T. ) ;
#32741=ORIENTED_EDGE ( 'NONE', *, *, #31891, .T. ) ;
#32742=EDGE_CURVE ( 'NONE', #28976, #26108, #26957, .T. ) ;
#32743=CARTESIAN_POINT ( 'NONE',  ( 15.99999999999998579, 124.9999999999999716, 162.9999999999999716 ) ) ;
#32746=CARTESIAN_POINT ( 'NONE',  ( -19.99999999999998934, -112.9999999999999858, 174.9999999999999432 ) ) ;
#32749=PLANE ( 'NONE',  #31433 ) ;
#32750=AXIS2_PLACEMENT_3D ( 'NONE', #32746, #23856, #6 ) ;
#32751=VERTEX_POINT ( 'NONE', #23175 ) ;
#32755=ORIENTED_EDGE ( 'NONE', *, *, #4935, .T. ) ;
#32756=VECTOR ( 'NONE', #11788, 1000.000000000000000 ) ;
#32757=DIRECTION ( 'NONE',  ( 0.000000000000000000, 0.000000000000000000, -1.000000000000000000 ) ) ;
#32763=PLANE ( 'NONE',  #27138 ) ;
#32766=ORIENTED_EDGE ( 'NONE', *, *, #16910, .F. ) ;
#32767=DIRECTION ( 'NONE',  ( -0.000000000000000000, -1.000000000000000000, -0.000000000000000000 ) ) ;
#32768=DIRECTION ( 'NONE',  ( 0.000000000000000000, 1.000000000000000000, 0.000000000000000000 ) ) ;
#32769=CIRCLE ( 'NONE', #19159, 3.999999999999976019 ) ;
#32775=CARTESIAN_POINT ( 'NONE',  ( 19.99999999999998934, 4.559999999999908127, 172.9900000000000091 ) ) ;
#32777=LINE ( 'NONE', #24058, #30976 ) ;
#32786=EDGE_CURVE ( 'NONE', #23404, #10477, #28381, .T. ) ;
#32788=DIRECTION ( 'NONE',  ( 0.000000000000000000, 1.000000000000000000, -3.374343856708137958E-53 ) ) ;
#32789=ORIENTED_EDGE ( 'NONE', *, *, #2326, .T. ) ;
#32790=CYLINDRICAL_SURFACE ( 'NONE', #23008, 7.999999999999979572 ) ;
#32796=AXIS2_PLACEMENT_3D ( 'NONE', #24839, #30548, #21646 ) ;
#32798=VERTEX_POINT ( 'NONE', #14696 ) ;
#32800=ORIENTED_EDGE ( 'NONE', *, *, #24121, .T. ) ;
#32801=ORIENTED_EDGE ( 'NONE', *, *, #7106, .F. ) ;
#32803=AXIS2_PLACEMENT_3D ( 'NONE', #31809, #2095, #7593 ) ;
#32805=DIRECTION ( 'NONE',  ( 1.000000000000000000, 0.000000000000000000, 0.000000000000000000 ) ) ;
#32806=LINE ( 'NONE', #32450, #2319 ) ;
#32810=CARTESIAN_POINT ( 'NONE',  ( -418.0000000000000000, -125.0000000000000000, -105.9999999999999574 ) ) ;
#32813=VERTEX_POINT ( 'NONE', #20373 ) ;
#32817=ORIENTED_EDGE ( 'NONE', *, *, #12070, .F. ) ;
#32821=DIRECTION ( 'NONE',  ( 1.000000000000000000, 0.000000000000000000, -1.848892746611746966E-32 ) ) ;
#32824=EDGE_CURVE ( 'NONE', #6833, #31113, #15038, .T. ) ;
#32825=ADVANCED_FACE ( 'NONE', ( #17892 ), #31051, .F. ) ;
#32830=VECTOR ( 'NONE', #27030, 1000.000000000000000 ) ;
#32835=EDGE_LOOP ( 'NONE', ( #33268, #32206, #29897, #19949 ) ) ;
#32843=CARTESIAN_POINT ( 'NONE',  ( 19.99999999999998224, 144.9999999999999147, 187.0000000000000000 ) ) ;
#32844=EDGE_CURVE ( 'NONE', #18562, #19944, #11657, .T. ) ;
#32848=CIRCLE ( 'NONE', #22070, 7.999999999999979572 ) ;
#32851=ORIENTED_EDGE ( 'NONE', *, *, #14033, .F. ) ;
#32852=ORIENTED_EDGE ( 'NONE', *, *, #16945, .T. ) ;
#32853=CARTESIAN_POINT ( 'NONE',  ( -365.0000000000000000, -114.9999999999999858, 113.9999999999999858 ) ) ;
#32854=CARTESIAN_POINT ( 'NONE',  ( -355.0000000000000000, -119.0000000000000000, 111.9999999999999858 ) ) ;
#32856=EDGE_CURVE ( 'NONE', #7282, #16746, #28722, .T. ) ;
#32861=DIRECTION ( 'NONE',  ( 1.000000000000000000, 0.000000000000000000, 0.000000000000000000 ) ) ;
#32862=CARTESIAN_POINT ( 'NONE',  ( -418.0000000000000000, 104.9999999999999858, -194.9999999999999716 ) ) ;
#32865=DIRECTION ( 'NONE',  ( 1.000000000000000000, 0.000000000000000000, 1.300283923313630633E-47 ) ) ;
#32867=AXIS2_PLACEMENT_3D ( 'NONE', #12701, #31374, #34399 ) ;
#32868=DIRECTION ( 'NONE',  ( 2.530127506375325574E-80, -1.000000000000000000, -6.842277657836020854E-49 ) ) ;
#32869=VERTEX_POINT ( 'NONE', #4321 ) ;
#32870=EDGE_CURVE ( 'NONE', #28035, #22441, #34349, .T. ) ;
#32871=LINE ( 'NONE', #13659, #15532 ) ;
#32876=AXIS2_PLACEMENT_3D ( 'NONE', #20480, #31326, #17825 ) ;
#32881=ORIENTED_EDGE ( 'NONE', *, *, #29304, .F. ) ;
#32885=DIRECTION ( 'NONE',  ( 0.000000000000000000, 0.000000000000000000, 1.000000000000000000 ) ) ;
#32887=EDGE_CURVE ( 'NONE', #17261, #35062, #13356, .T. ) ;
#32888=CARTESIAN_POINT ( 'NONE',  ( 19.99999999999998934, -115.0000000000000000, 162.9999999999999716 ) ) ;
#32892=LINE ( 'NONE', #14222, #854 ) ;
#32895=EDGE_LOOP ( 'NONE', ( #23904, #7219, #33682, #20800 ) ) ;
#32904=DIRECTION ( 'NONE',  ( 0.000000000000000000, 1.000000000000000000, 0.000000000000000000 ) ) ;
#32907=LINE ( 'NONE', #356, #16002 ) ;
#32909=CIRCLE ( 'NONE', #7913, 3.999999999999976019 ) ;
#32911=CARTESIAN_POINT ( 'NONE',  ( -499.9999999999999432, 140.9999999999999716, -162.9999999999999716 ) ) ;
#32917=AXIS2_PLACEMENT_3D ( 'NONE', #22509, #30860, #8794 ) ;
#32922=FACE_BOUND ( 'NONE', #31090, .T. ) ;
#32924=ORIENTED_EDGE ( 'NONE', *, *, #13301, .T. ) ;
#32927=ORIENTED_EDGE ( 'NONE', *, *, #14484, .T. ) ;
#32935=EDGE_CURVE ( 'NONE', #30302, #31113, #13237, .T. ) ;
#32937=LINE ( 'NONE', #19788, #23548 ) ;
#32939=ORIENTED_EDGE ( 'NONE', *, *, #13717, .F. ) ;
#32942=CARTESIAN_POINT ( 'NONE',  ( -20.00000000000004619, 124.9999999999999716, 162.9999999999999716 ) ) ;
#32946=DIRECTION ( 'NONE',  ( -3.040835319149746090E-31, -1.000000000000000000, 3.748118910144520367E-63 ) ) ;
#32947=DIRECTION ( 'NONE',  ( 0.000000000000000000, 1.310824597558155437E-49, 1.000000000000000000 ) ) ;
#32948=LINE ( 'NONE', #2528, #22617 ) ;
#32951=CARTESIAN_POINT ( 'NONE',  ( -410.0000000000000568, 124.9999999999999574, -187.0000000000000000 ) ) ;
#32952=DIRECTION ( 'NONE',  ( -0.000000000000000000, -0.000000000000000000, -1.000000000000000000 ) ) ;
#32953=CARTESIAN_POINT ( 'NONE',  ( -365.0000000000000000, -135.0000000000000000, 126.0000000000000000 ) ) ;
#32956=VERTEX_POINT ( 'NONE', #2536 ) ;
#32958=FACE_BOUND ( 'NONE', #21559, .T. ) ;
#32962=ORIENTED_EDGE ( 'NONE', *, *, #15153, .T. ) ;
#32965=CARTESIAN_POINT ( 'NONE',  ( -418.0000000000000000, -124.9999999999999858, -77.99999999999997158 ) ) ;
#32967=VERTEX_POINT ( 'NONE', #2188 ) ;
#32972=CARTESIAN_POINT ( 'NONE',  ( 11.99999999999999645, 112.9999999999999574, -175.0000000000000284 ) ) ;
#32976=ORIENTED_EDGE ( 'NONE', *, *, #5875, .F. ) ;
#32977=DIRECTION ( 'NONE',  ( 1.000000000000000000, 0.000000000000000000, 0.000000000000000000 ) ) ;
#32978=LINE ( 'NONE', #11293, #9564 ) ;
#32982=ORIENTED_EDGE ( 'NONE', *, *, #9437, .F. ) ;
#32983=AXIS2_PLACEMENT_3D ( 'NONE', #17963, #15279, #1729 ) ;
#32989=CARTESIAN_POINT ( 'NONE',  ( -414.0000000000000568, 104.9999999999999858, -187.0000000000000000 ) ) ;
#32991=DIRECTION ( 'NONE',  ( 1.000000000000000000, 0.000000000000000000, 0.000000000000000000 ) ) ;
#32992=EDGE_LOOP ( 'NONE', ( #8548, #22436, #32976, #15229 ) ) ;
#32995=DIRECTION ( 'NONE',  ( 2.891205793294675861E-16, 0.000000000000000000, 1.000000000000000000 ) ) ;
#32998=LINE ( 'NONE', #94, #23682 ) ;
#33002=AXIS2_PLACEMENT_3D ( 'NONE', #33216, #9188, #6148 ) ;
#33004=AXIS2_PLACEMENT_3D ( 'NONE', #25904, #1858, #9698 ) ;
#33006=ORIENTED_EDGE ( 'NONE', *, *, #12423, .F. ) ;
#33009=ORIENTED_EDGE ( 'NONE', *, *, #10037, .T. ) ;
#33011=CARTESIAN_POINT ( 'NONE',  ( -499.9999999999999432, -137.0000000000000000, -187.0000000000000000 ) ) ;
#33013=CARTESIAN_POINT ( 'NONE',  ( 19.99999999999990763, -134.9999999999999716, -186.9999999999999716 ) ) ;
#33025=CIRCLE ( 'NONE', #13729, 3.999999999999976019 ) ;
#33030=DIRECTION ( 'NONE',  ( 0.000000000000000000, 5.145227585319922065E-49, 1.000000000000000000 ) ) ;
#33031=CARTESIAN_POINT ( 'NONE',  ( -410.0000000000000568, -105.0000000000000142, 187.0000000000000000 ) ) ;
#33033=AXIS2_PLACEMENT_3D ( 'NONE', #25685, #606, #25509 ) ;
#33035=CARTESIAN_POINT ( 'NONE',  ( -12.00000000000001066, 134.9999999999999432, -162.9999999999999432 ) ) ;
#33037=VECTOR ( 'NONE', #33258, 1000.000000000000000 ) ;
#33043=DIRECTION ( 'NONE',  ( 0.000000000000000000, 0.000000000000000000, -1.000000000000000000 ) ) ;
#33045=EDGE_CURVE ( 'NONE', #17362, #12453, #30957, .T. ) ;
#33047=AXIS2_PLACEMENT_3D ( 'NONE', #27221, #30426, #6023 ) ;
#33049=CIRCLE ( 'NONE', #4055, 7.999999999999979572 ) ;
#33052=CARTESIAN_POINT ( 'NONE',  ( 15.99999999999998579, 136.9999999999999716, -175.0000000000000284 ) ) ;
#33059=CARTESIAN_POINT ( 'NONE',  ( -442.0000000000000000, 105.0000000000000142, 100.0000000000000000 ) ) ;
#33062=CARTESIAN_POINT ( 'NONE',  ( -15.99999999999998579, 75.55999999999990280, -168.2400000000000091 ) ) ;
#33066=ORIENTED_EDGE ( 'NONE', *, *, #5241, .T. ) ;
#33067=EDGE_CURVE ( 'NONE', #8689, #16065, #4782, .T. ) ;
#33070=VERTEX_POINT ( 'NONE', #32953 ) ;
#33072=( LENGTH_UNIT ( ) NAMED_UNIT ( * ) SI_UNIT ( .MILLI., .METRE. ) );
#33073=ADVANCED_FACE ( 'NONE', ( #27977 ), #16618, .F. ) ;
#33076=CARTESIAN_POINT ( 'NONE',  ( -20.00000000000007461, 104.9999999999999858, -187.0000000000000000 ) ) ;
#33085=CARTESIAN_POINT ( 'NONE',  ( -499.9999999999999432, 136.9999999999999432, -155.0000000000000000 ) ) ;
#33086=VERTEX_POINT ( 'NONE', #13935 ) ;
#33087=ORIENTED_EDGE ( 'NONE', *, *, #10348, .F. ) ;
#33099=FACE_OUTER_BOUND ( 'NONE', #7741, .T. ) ;
#33107=ADVANCED_FACE ( 'NONE', ( #14294 ), #27271, .T. ) ;
#33112=DIRECTION ( 'NONE',  ( 0.000000000000000000, 1.000000000000000000, 5.145227585319922065E-49 ) ) ;
#33117=DIRECTION ( 'NONE',  ( -3.469446951953832974E-18, -1.000000000000000000, -7.888609052210116302E-31 ) ) ;
#33120=ORIENTED_EDGE ( 'NONE', *, *, #29581, .T. ) ;
#33123=FACE_OUTER_BOUND ( 'NONE', #29785, .T. ) ;
#33124=DIRECTION ( 'NONE',  ( -1.000000000000000000, 0.000000000000000000, 0.000000000000000000 ) ) ;
#33125=LINE ( 'NONE', #30468, #7016 ) ;
#33127=CARTESIAN_POINT ( 'NONE',  ( -500.0000000000000000, -109.0000000000000142, 187.0000000000000000 ) ) ;
#33131=VECTOR ( 'NONE', #4659, 1000.000000000000000 ) ;
#33132=ORIENTED_EDGE ( 'NONE', *, *, #22190, .F. ) ;
#33135=CARTESIAN_POINT ( 'NONE',  ( -499.9999999999998863, -109.0000000000000142, -162.9999999999999716 ) ) ;
#33138=DIRECTION ( 'NONE',  ( 0.000000000000000000, 0.000000000000000000, -1.000000000000000000 ) ) ;
#33139=DIRECTION ( 'NONE',  ( 1.000000000000000000, 0.000000000000000000, 0.000000000000000000 ) ) ;
#33140=EDGE_CURVE ( 'NONE', #19088, #28627, #16976, .T. ) ;
#33141=UNCERTAINTY_MEASURE_WITH_UNIT (LENGTH_MEASURE( 1.000000000000000082E-05 ), #29332, 'distance_accuracy_value', 'NONE');
#33142=PLANE ( 'NONE',  #14454 ) ;
#33144=LINE ( 'NONE', #8760, #21849 ) ;
#33145=PLANE ( 'NONE',  #9759 ) ;
#33147=CIRCLE ( 'NONE', #25185, 3.999999999999976019 ) ;
#33149=ORIENTED_EDGE ( 'NONE', *, *, #19455, .F. ) ;
#33151=AXIS2_PLACEMENT_3D ( 'NONE', #33761, #20247, #20417 ) ;
#33153=ORIENTED_EDGE ( 'NONE', *, *, #19986, .T. ) ;
#33155=EDGE_LOOP ( 'NONE', ( #14668, #569, #3554, #5285 ) ) ;
#33156=ORIENTED_EDGE ( 'NONE', *, *, #21891, .F. ) ;
#33157=LINE ( 'NONE', #24430, #32073 ) ;
#33160=DIRECTION ( 'NONE',  ( 0.000000000000000000, -1.310824597558155437E-49, -1.000000000000000000 ) ) ;
#33161=DIRECTION ( 'NONE',  ( -1.000000000000000000, 0.000000000000000000, 0.000000000000000000 ) ) ;
#33163=EDGE_LOOP ( 'NONE', ( #15364, #15952, #29052, #14623 ) ) ;
#33164=LINE ( 'NONE', #11292, #2052 ) ;
#33167=CARTESIAN_POINT ( 'NONE',  ( -430.0000000000000000, -119.0000000000000000, 128.0000000000000000 ) ) ;
#33168=CARTESIAN_POINT ( 'NONE',  ( -19.99999999999998934, 75.55999999999990280, -168.2400000000000091 ) ) ;
#33171=AXIS2_PLACEMENT_3D ( 'NONE', #25290, #9101, #22639 ) ;
#33176=CARTESIAN_POINT ( 'NONE',  ( -430.0000000000000000, 130.9999999999999716, 128.0000000000000000 ) ) ;
#33177=EDGE_CURVE ( 'NONE', #32711, #14881, #29951, .T. ) ;
#33178=LINE ( 'NONE', #27135, #18603 ) ;
#33181=CYLINDRICAL_SURFACE ( 'NONE', #3127, 3.999999999999976019 ) ;
#33182=EDGE_CURVE ( 'NONE', #11239, #30715, #25477, .T. ) ;
#33184=AXIS2_PLACEMENT_3D ( 'NONE', #15924, #5028, #26574 ) ;
#33186=ORIENTED_EDGE ( 'NONE', *, *, #18312, .T. ) ;
#33196=VERTEX_POINT ( 'NONE', #28848 ) ;
#33197=CARTESIAN_POINT ( 'NONE',  ( -70.00000000000000000, 4.559999999999908127, 168.2400000000000091 ) ) ;
#33199=ORIENTED_EDGE ( 'NONE', *, *, #25602, .T. ) ;
#33203=AXIS2_PLACEMENT_3D ( 'NONE', #290, #13994, #11153 ) ;
#33206=CARTESIAN_POINT ( 'NONE',  ( 11.99999999999995559, -145.0000000000000000, 162.9999999999999716 ) ) ;
#33207=CARTESIAN_POINT ( 'NONE',  ( -499.9999999999999432, 136.9999999999999432, -155.0000000000000000 ) ) ;
#33208=ORIENTED_EDGE ( 'NONE', *, *, #4038, .F. ) ;
#33214=CIRCLE ( 'NONE', #26961, 2.000000000000001776 ) ;
#33216=CARTESIAN_POINT ( 'NONE',  ( -442.0000000000000000, -105.0000000000000142, 187.0000000000000000 ) ) ;
#33217=CARTESIAN_POINT ( 'NONE',  ( -442.0000000000000000, -105.0000000000000142, 162.9999999999999716 ) ) ;
#33220=FACE_BOUND ( 'NONE', #18261, .T. ) ;
#33221=LINE ( 'NONE', #12408, #11471 ) ;
#33222=EDGE_CURVE ( 'NONE', #27222, #32157, #25276, .T. ) ;
#33224=ORIENTED_EDGE ( 'NONE', *, *, #28057, .T. ) ;
#33226=FACE_OUTER_BOUND ( 'NONE', #4204, .T. ) ;
#33230=CIRCLE ( 'NONE', #20737, 7.999999999999979572 ) ;
#33231=PLANE ( 'NONE',  #17765 ) ;
#33232=EDGE_CURVE ( 'NONE', #32751, #3477, #28338, .T. ) ;
#33235=EDGE_LOOP ( 'NONE', ( #20751, #18726, #17269, #16676 ) ) ;
#33237=EDGE_CURVE ( 'NONE', #23877, #28310, #28130, .T. ) ;
#33238=VECTOR ( 'NONE', #3896, 1000.000000000000000 ) ;
#33241=CARTESIAN_POINT ( 'NONE',  ( -500.0000000000000000, -113.0000000000000000, -155.0000000000000000 ) ) ;
#33243=ORIENTED_EDGE ( 'NONE', *, *, #22676, .F. ) ;
#33246=ORIENTED_EDGE ( 'NONE', *, *, #34109, .F. ) ;
#33248=ADVANCED_FACE ( 'NONE', ( #9109 ), #22818, .F. ) ;
#33251=FACE_OUTER_BOUND ( 'NONE', #28526, .T. ) ;
#33252=CARTESIAN_POINT ( 'NONE',  ( -347.0000000000000000, -125.0000000000000284, 181.0000000000000000 ) ) ;
#33254=ORIENTED_EDGE ( 'NONE', *, *, #8348, .T. ) ;
#33255=ORIENTED_EDGE ( 'NONE', *, *, #10011, .F. ) ;
#33256=DIRECTION ( 'NONE',  ( 0.000000000000000000, 2.309213040847544338E-50, 1.000000000000000000 ) ) ;
#33258=DIRECTION ( 'NONE',  ( 0.000000000000000000, 1.000000000000000000, -6.842277657836020854E-49 ) ) ;
#33259=DIRECTION ( 'NONE',  ( 0.000000000000000000, 1.000000000000000000, 1.224646799147353207E-16 ) ) ;
#33261=VERTEX_POINT ( 'NONE', #3929 ) ;
#33262=ORIENTED_EDGE ( 'NONE', *, *, #5883, .T. ) ;
#33263=FACE_OUTER_BOUND ( 'NONE', #21929, .T. ) ;
#33267=CARTESIAN_POINT ( 'NONE',  ( -20.00000000000004619, 112.9999999999999574, 155.0000000000000000 ) ) ;
#33268=ORIENTED_EDGE ( 'NONE', *, *, #23510, .F. ) ;
#33271=DIRECTION ( 'NONE',  ( -0.000000000000000000, -0.000000000000000000, 1.000000000000000000 ) ) ;
#33275=DIRECTION ( 'NONE',  ( -0.000000000000000000, 1.000000000000000000, -0.000000000000000000 ) ) ;
#33276=LINE ( 'NONE', #6865, #29918 ) ;
#33279=EDGE_CURVE ( 'NONE', #30178, #30541, #13937, .T. ) ;
#33280=VECTOR ( 'NONE', #25516, 1000.000000000000000 ) ;
#33283=PLANE ( 'NONE',  #29084 ) ;
#33293=CARTESIAN_POINT ( 'NONE',  ( -499.9999999999999432, -137.0000000000000000, -190.9999999999999716 ) ) ;
#33296=VERTEX_POINT ( 'NONE', #34017 ) ;
#33297=DIRECTION ( 'NONE',  ( 1.000000000000000000, 0.000000000000000000, 5.546364386991661285E-52 ) ) ;
#33299=ADVANCED_FACE ( 'NONE', ( #26004, #1622 ), #23336, .T. ) ;
#33303=DIRECTION ( 'NONE',  ( 0.000000000000000000, -6.123233995736766036E-17, -1.000000000000000000 ) ) ;
#33305=ORIENTED_EDGE ( 'NONE', *, *, #33922, .F. ) ;
#33306=ORIENTED_EDGE ( 'NONE', *, *, #27125, .T. ) ;
#33308=VECTOR ( 'NONE', #29859, 1000.000000000000000 ) ;
#33311=DIRECTION ( 'NONE',  ( 0.000000000000000000, -0.000000000000000000, -1.000000000000000000 ) ) ;
#33313=ORIENTED_EDGE ( 'NONE', *, *, #31412, .F. ) ;
#33314=CARTESIAN_POINT ( 'NONE',  ( -499.9999999999999432, 112.9999999999999574, -190.9999999999999716 ) ) ;
#33315=DIRECTION ( 'NONE',  ( 1.000000000000000000, 0.000000000000000000, 5.546364386991661285E-52 ) ) ;
#33318=AXIS2_PLACEMENT_3D ( 'NONE', #25259, #15085, #3545 ) ;
#33324=LINE ( 'NONE', #20331, #21272 ) ;
#33325=VERTEX_POINT ( 'NONE', #26352 ) ;
#33327=CYLINDRICAL_SURFACE ( 'NONE', #16666, 7.999999999999979572 ) ;
#33329=AXIS2_PLACEMENT_3D ( 'NONE', #9795, #9098, #20657 ) ;
#33330=ORIENTED_EDGE ( 'NONE', *, *, #25717, .F. ) ;
#33331=AXIS2_PLACEMENT_3D ( 'NONE', #5059, #16124, #31940 ) ;
#33332=ORIENTED_EDGE ( 'NONE', *, *, #5675, .F. ) ;
#33335=ORIENTED_EDGE ( 'NONE', *, *, #13932, .F. ) ;
#33337=DIRECTION ( 'NONE',  ( -1.000000000000000000, -3.469446951953834515E-18, 0.000000000000000000 ) ) ;
#33338=AXIS2_PLACEMENT_3D ( 'NONE', #29820, #5422, #21631 ) ;
#33339=ADVANCED_FACE ( 'NONE', ( #15697 ), #24022, .F. ) ;
#33343=CARTESIAN_POINT ( 'NONE',  ( -349.0000000000000000, -125.0000000000000284, 185.0000000000000000 ) ) ;
#33344=ORIENTED_EDGE ( 'NONE', *, *, #26968, .F. ) ;
#33346=DIRECTION ( 'NONE',  ( -1.000000000000000000, 2.530127506375325948E-80, -1.848892746611746419E-32 ) ) ;
#33350=DIRECTION ( 'NONE',  ( 0.000000000000000000, 1.000000000000000000, 1.224646799147353207E-16 ) ) ;
#33353=VECTOR ( 'NONE', #27044, 1000.000000000000000 ) ;
#33356=VERTEX_POINT ( 'NONE', #14023 ) ;
#33357=LINE ( 'NONE', #789, #3777 ) ;
#33360=CARTESIAN_POINT ( 'NONE',  ( 19.99999999999998224, 134.9999999999999432, -162.9999999999999432 ) ) ;
#33364=EDGE_LOOP ( 'NONE', ( #16502, #1258 ) ) ;
#33365=CARTESIAN_POINT ( 'NONE',  ( -20.00000000000001776, -113.0000000000000000, 187.0000000000000000 ) ) ;
#33366=LINE ( 'NONE', #19858, #6876 ) ;
#33374=VECTOR ( 'NONE', #6068, 1000.000000000000000 ) ;
#33376=CARTESIAN_POINT ( 'NONE',  ( -410.0000000000000568, 137.0000000000000000, -175.0000000000000000 ) ) ;
#33377=EDGE_LOOP ( 'NONE', ( #6356, #8876, #23440, #22812 ) ) ;
#33379=CARTESIAN_POINT ( 'NONE',  ( -19.99999999999998934, 134.9999999999998863, 162.9999999999999716 ) ) ;
#33380=ADVANCED_FACE ( 'NONE', ( #5630 ), #12847, .F. ) ;
#33381=AXIS2_PLACEMENT_3D ( 'NONE', #9880, #23586, #1695 ) ;
#33383=EDGE_CURVE ( 'NONE', #15713, #26361, #18502, .T. ) ;
#33387=ORIENTED_EDGE ( 'NONE', *, *, #34373, .F. ) ;
#33392=LINE ( 'NONE', #19051, #3332 ) ;
#33394=DIRECTION ( 'NONE',  ( 0.000000000000000000, -1.000000000000000000, 3.374343856708137958E-53 ) ) ;
#33397=VERTEX_POINT ( 'NONE', #13195 ) ;
#33398=DIRECTION ( 'NONE',  ( 1.000000000000000000, 0.000000000000000000, 0.000000000000000000 ) ) ;
#33399=FACE_OUTER_BOUND ( 'NONE', #5687, .T. ) ;
#33402=VECTOR ( 'NONE', #12991, 1000.000000000000000 ) ;
#33404=CARTESIAN_POINT ( 'NONE',  ( -363.0000000000000000, 124.9999999999999432, 168.9999999999999716 ) ) ;
#33405=ORIENTED_EDGE ( 'NONE', *, *, #2955, .T. ) ;
#33407=DIRECTION ( 'NONE',  ( 0.000000000000000000, -2.309213040847544338E-50, -1.000000000000000000 ) ) ;
#33411=DIRECTION ( 'NONE',  ( 0.000000000000000000, -1.310824597558155437E-49, -1.000000000000000000 ) ) ;
#33413=ORIENTED_EDGE ( 'NONE', *, *, #17908, .F. ) ;
#33418=DIRECTION ( 'NONE',  ( 1.000000000000000000, -1.270085550689488560E-30, -2.891205793294675368E-16 ) ) ;
#33420=CARTESIAN_POINT ( 'NONE',  ( -442.0000000000000000, -109.0000000000000142, -155.0000000000000000 ) ) ;
#33422=VECTOR ( 'NONE', #21525, 1000.000000000000000 ) ;
#33433=DIRECTION ( 'NONE',  ( 1.000000000000000000, 0.000000000000000000, 0.000000000000000000 ) ) ;
#33435=EDGE_LOOP ( 'NONE', ( #31604, #2887, #9340, #28937 ) ) ;
#33437=CARTESIAN_POINT ( 'NONE',  ( -12.00000000000001066, 144.9999999999999716, -155.0000000000000000 ) ) ;
#33438=CARTESIAN_POINT ( 'NONE',  ( -418.0000000000000000, 105.0000000000000142, -101.9999999999999858 ) ) ;
#33444=ORIENTED_EDGE ( 'NONE', *, *, #21571, .F. ) ;
#33447=AXIS2_PLACEMENT_3D ( 'NONE', #32584, #24756, #22100 ) ;
#33450=DIRECTION ( 'NONE',  ( 0.000000000000000000, 0.000000000000000000, -1.000000000000000000 ) ) ;
#33452=DIRECTION ( 'NONE',  ( 0.000000000000000000, 1.000000000000000000, 2.465190328815662439E-32 ) ) ;
#33455=CYLINDRICAL_SURFACE ( 'NONE', #28686, 7.999999999999979572 ) ;
#33456=DIRECTION ( 'NONE',  ( 0.000000000000000000, 0.000000000000000000, 1.000000000000000000 ) ) ;
#33458=AXIS2_PLACEMENT_3D ( 'NONE', #7418, #10279, #28975 ) ;
#33459=ORIENTED_EDGE ( 'NONE', *, *, #20323, .T. ) ;
#33464=CIRCLE ( 'NONE', #16442, 7.999999999999979572 ) ;
#33472=DIRECTION ( 'NONE',  ( 0.000000000000000000, 0.000000000000000000, -1.000000000000000000 ) ) ;
#33489=EDGE_CURVE ( 'NONE', #23786, #16134, #17591, .T. ) ;
#33494=PLANE ( 'NONE',  #9335 ) ;
#33498=CARTESIAN_POINT ( 'NONE',  ( -361.0000000000000000, -135.0000000000000000, 113.9999999999999858 ) ) ;
#33499=EDGE_CURVE ( 'NONE', #23038, #5682, #3500, .T. ) ;
#33501=EDGE_CURVE ( 'NONE', #7081, #16235, #27712, .T. ) ;
#33502=ORIENTED_EDGE ( 'NONE', *, *, #17772, .F. ) ;
#33503=EDGE_CURVE ( 'NONE', #27359, #20509, #22912, .T. ) ;
#33509=CYLINDRICAL_SURFACE ( 'NONE', #17380, 2.000000000000001776 ) ;
#33510=VECTOR ( 'NONE', #26694, 1000.000000000000000 ) ;
#33513=LINE ( 'NONE', #11457, #2347 ) ;
#33516=EDGE_CURVE ( 'NONE', #19582, #6460, #9387, .T. ) ;
#33518=DIRECTION ( 'NONE',  ( 0.000000000000000000, -1.000000000000000000, -1.310824597558155437E-49 ) ) ;
#33521=CARTESIAN_POINT ( 'NONE',  ( 15.99999999999997868, 136.9999999999999716, 155.0000000000000000 ) ) ;
#33522=DIRECTION ( 'NONE',  ( 1.000000000000000000, 3.469446951953834515E-18, 0.000000000000000000 ) ) ;
#33535=CARTESIAN_POINT ( 'NONE',  ( 11.99999999999999645, 144.9999999999999716, -190.9999999999999432 ) ) ;
#33536=ORIENTED_EDGE ( 'NONE', *, *, #26906, .T. ) ;
#33540=EDGE_CURVE ( 'NONE', #27942, #2181, #8848, .T. ) ;
#33541=EDGE_CURVE ( 'NONE', #2254, #30412, #11891, .T. ) ;
#33545=VERTEX_POINT ( 'NONE', #25565 ) ;
#33547=EDGE_CURVE ( 'NONE', #30842, #19088, #27565, .T. ) ;
#33552=FACE_OUTER_BOUND ( 'NONE', #32126, .T. ) ;
#33555=DIRECTION ( 'NONE',  ( 0.000000000000000000, 0.000000000000000000, -1.000000000000000000 ) ) ;
#33558=ORIENTED_EDGE ( 'NONE', *, *, #25662, .T. ) ;
#33559=FACE_OUTER_BOUND ( 'NONE', #16471, .T. ) ;
#33561=LINE ( 'NONE', #30900, #24274 ) ;
#33562=CARTESIAN_POINT ( 'NONE',  ( 12.00000000000001066, 134.9999999999999432, -154.9999999999999716 ) ) ;
#33565=AXIS2_PLACEMENT_3D ( 'NONE', #25592, #22763, #17787 ) ;
#33568=EDGE_CURVE ( 'NONE', #20411, #13771, #19544, .T. ) ;
#33570=CARTESIAN_POINT ( 'NONE',  ( 19.99999999999998934, -115.0000000000000000, 162.9999999999999716 ) ) ;
#33573=CARTESIAN_POINT ( 'NONE',  ( -365.0000000000000000, 118.9999999999999716, 126.0000000000000000 ) ) ;
#33574=ORIENTED_EDGE ( 'NONE', *, *, #30444, .F. ) ;
#33575=AXIS2_PLACEMENT_3D ( 'NONE', #4874, #20574, #15772 ) ;
#33579=CIRCLE ( 'NONE', #32983, 7.999999999999986677 ) ;
#33581=EDGE_CURVE ( 'NONE', #19630, #21502, #27886, .T. ) ;
#33583=DIRECTION ( 'NONE',  ( 1.000000000000000000, 0.000000000000000000, 0.000000000000000000 ) ) ;
#33584=CARTESIAN_POINT ( 'NONE',  ( -363.0000000000000000, 134.9999999999999716, 114.0000000000000000 ) ) ;
#33588=VECTOR ( 'NONE', #29236, 1000.000000000000000 ) ;
#33590=VECTOR ( 'NONE', #20589, 1000.000000000000000 ) ;
#33601=VERTEX_POINT ( 'NONE', #844 ) ;
#33602=CIRCLE ( 'NONE', #22254, 7.999999999999986677 ) ;
#33604=CARTESIAN_POINT ( 'NONE',  ( -499.9999999999999432, -113.0000000000000000, -162.9999999999999716 ) ) ;
#33605=VECTOR ( 'NONE', #1688, 1000.000000000000000 ) ;
#33609=DIRECTION ( 'NONE',  ( 1.000000000000000000, 0.000000000000000000, -1.848892746611746966E-32 ) ) ;
#33610=LINE ( 'NONE', #395, #16995 ) ;
#33611=ORIENTED_EDGE ( 'NONE', *, *, #12621, .F. ) ;
#33613=CARTESIAN_POINT ( 'NONE',  ( -12.00000000000001066, 124.9999999999999716, 187.0000000000000000 ) ) ;
#33615=EDGE_LOOP ( 'NONE', ( #21621, #28146, #3394, #17808 ) ) ;
#33616=ORIENTED_EDGE ( 'NONE', *, *, #31936, .T. ) ;
#33617=DIRECTION ( 'NONE',  ( 1.000000000000000000, 0.000000000000000000, -1.848892746611746966E-32 ) ) ;
#33620=DIRECTION ( 'NONE',  ( 0.000000000000000000, 1.000000000000000000, -3.374343856708137958E-53 ) ) ;
#33621=CIRCLE ( 'NONE', #22830, 2.000000000000001776 ) ;
#33622=ORIENTED_EDGE ( 'NONE', *, *, #34314, .F. ) ;
#33623=STYLED_ITEM('',(#35254),#22535);
#33624=FACE_OUTER_BOUND ( 'NONE', #28490, .T. ) ;
#33628=EDGE_CURVE ( 'NONE', #30776, #12415, #23426, .T. ) ;
#33630=LINE ( 'NONE', #20120, #34978 ) ;
#33632=EDGE_CURVE ( 'NONE', #22581, #27476, #18278, .T. ) ;
#33638=VECTOR ( 'NONE', #14956, 1000.000000000000000 ) ;
#33642=ORIENTED_EDGE ( 'NONE', *, *, #4000, .F. ) ;
#33643=AXIS2_PLACEMENT_3D ( 'NONE', #20964, #31465, #28972 ) ;
#33645=DIRECTION ( 'NONE',  ( 0.000000000000000000, 0.000000000000000000, -1.000000000000000000 ) ) ;
#33649=DIRECTION ( 'NONE',  ( 0.000000000000000000, -1.000000000000000000, 6.123233995736766036E-17 ) ) ;
#33652=EDGE_LOOP ( 'NONE', ( #15813, #23872, #4702, #33616, #5144 ) ) ;
#33662=DIRECTION ( 'NONE',  ( -1.000000000000000000, 0.000000000000000000, 1.848892746611746966E-32 ) ) ;
#33663=DIRECTION ( 'NONE',  ( -1.000000000000000000, 0.000000000000000000, -5.546364386991661285E-52 ) ) ;
#33665=DIRECTION ( 'NONE',  ( -1.000000000000000000, 0.000000000000000000, -0.000000000000000000 ) ) ;
#33666=CARTESIAN_POINT ( 'NONE',  ( -15.99999999999998579, -56.99999999999997868, -175.0000000000000000 ) ) ;
#33674=EDGE_CURVE ( 'NONE', #14836, #5864, #21093, .T. ) ;
#33676=ADVANCED_FACE ( 'NONE', ( #20935 ), #23095, .F. ) ;
#33677=EDGE_CURVE ( 'NONE', #181, #4287, #16570, .T. ) ;
#33682=ORIENTED_EDGE ( 'NONE', *, *, #6264, .T. ) ;
#33688=LINE ( 'NONE', #23196, #10120 ) ;
#33690=DIRECTION ( 'NONE',  ( -0.000000000000000000, -1.000000000000000000, -0.000000000000000000 ) ) ;
#33691=VERTEX_POINT ( 'NONE', #1713 ) ;
#33693=VERTEX_POINT ( 'NONE', #2065 ) ;
#33694=DIRECTION ( 'NONE',  ( 0.000000000000000000, 1.000000000000000000, -3.374343856708137958E-53 ) ) ;
#33700=ADVANCED_FACE ( 'NONE', ( #12580 ), #7565, .F. ) ;
#33703=EDGE_CURVE ( 'NONE', #21709, #10179, #32305, .T. ) ;
#33704=DIRECTION ( 'NONE',  ( 0.000000000000000000, 1.000000000000000000, 5.053935297177146739E-49 ) ) ;
#33715=ORIENTED_EDGE ( 'NONE', *, *, #761, .T. ) ;
#33721=EDGE_LOOP ( 'NONE', ( #18780, #25380, #34491, #30419, #30514, #573, #10842, #30766, #19587, #31055, #5865 ) ) ;
#33723=EDGE_CURVE ( 'NONE', #28881, #17261, #16485, .T. ) ;
#33728=ORIENTED_EDGE ( 'NONE', *, *, #5639, .F. ) ;
#33730=ORIENTED_EDGE ( 'NONE', *, *, #19986, .F. ) ;
#33731=ORIENTED_EDGE ( 'NONE', *, *, #15174, .F. ) ;
#33733=DIRECTION ( 'NONE',  ( 0.000000000000000000, -2.465190328815661892E-32, -1.000000000000000000 ) ) ;
#33739=CARTESIAN_POINT ( 'NONE',  ( -20.00000000000004619, -137.0000000000000000, -159.0000000000000000 ) ) ;
#33740=DIRECTION ( 'NONE',  ( 1.232595164407830946E-32, 0.000000000000000000, 1.000000000000000000 ) ) ;
#33741=LINE ( 'NONE', #31421, #25449 ) ;
#33743=CARTESIAN_POINT ( 'NONE',  ( -20.00000000000001776, -109.0000000000000142, 187.0000000000000000 ) ) ;
#33744=DIRECTION ( 'NONE',  ( 0.000000000000000000, -1.131431318426415506E-52, -1.000000000000000000 ) ) ;
#33747=EDGE_CURVE ( 'NONE', #14902, #13888, #29641, .T. ) ;
#33749=AXIS2_PLACEMENT_3D ( 'NONE', #29473, #5066, #18454 ) ;
#33754=EDGE_CURVE ( 'NONE', #7236, #4465, #26618, .T. ) ;
#33760=ADVANCED_FACE ( 'NONE', ( #29995 ), #5069, .F. ) ;
#33761=CARTESIAN_POINT ( 'NONE',  ( -442.0000000000000000, -125.0000000000000000, -101.9999999999999858 ) ) ;
#33762=ORIENTED_EDGE ( 'NONE', *, *, #13717, .T. ) ;
#33763=CARTESIAN_POINT ( 'NONE',  ( -365.0000000000000000, -133.0000000000000000, 126.0000000000000000 ) ) ;
#33769=CARTESIAN_POINT ( 'NONE',  ( -445.9999999999999432, -112.9999999999999858, -155.0000000000000000 ) ) ;
#33773=AXIS2_PLACEMENT_3D ( 'NONE', #15701, #34193, #31521 ) ;
#33775=VECTOR ( 'NONE', #6654, 1000.000000000000000 ) ;
#33779=AXIS2_PLACEMENT_3D ( 'NONE', #15850, #24350, #34518 ) ;
#33780=LINE ( 'NONE', #23280, #20952 ) ;
#33785=ORIENTED_EDGE ( 'NONE', *, *, #17597, .T. ) ;
#33787=( NAMED_UNIT ( * ) SI_UNIT ( $, .STERADIAN. ) SOLID_ANGLE_UNIT ( ) );
#33788=FACE_OUTER_BOUND ( 'NONE', #32182, .T. ) ;
#33793=CARTESIAN_POINT ( 'NONE',  ( -12.00000000000001066, -137.0000000000000000, 155.0000000000000000 ) ) ;
#33796=EDGE_LOOP ( 'NONE', ( #27641, #31539, #30317, #21388 ) ) ;
#33799=VERTEX_POINT ( 'NONE', #6530 ) ;
#33801=DIRECTION ( 'NONE',  ( 0.000000000000000000, -1.310824597558155437E-49, -1.000000000000000000 ) ) ;
#33802=VECTOR ( 'NONE', #28553, 1000.000000000000000 ) ;
#33805=ORIENTED_EDGE ( 'NONE', *, *, #27755, .F. ) ;
#33808=CARTESIAN_POINT ( 'NONE',  ( 15.99999999999998579, -137.0000000000000000, 174.9999999999999432 ) ) ;
#33810=FACE_OUTER_BOUND ( 'NONE', #29409, .T. ) ;
#33813=AXIS2_PLACEMENT_3D ( 'NONE', #34080, #31071, #12388 ) ;
#33815=ORIENTED_EDGE ( 'NONE', *, *, #27633, .F. ) ;
#33817=ORIENTED_EDGE ( 'NONE', *, *, #24368, .T. ) ;
#33820=CARTESIAN_POINT ( 'NONE',  ( 11.99999999999999645, -115.0000000000000000, 162.9999999999999716 ) ) ;
#33821=AXIS2_PLACEMENT_3D ( 'NONE', #6427, #23171, #9471 ) ;
#33822=PLANE ( 'NONE',  #7965 ) ;
#33824=ORIENTED_EDGE ( 'NONE', *, *, #21412, .T. ) ;
#33825=PLANE ( 'NONE',  #20779 ) ;
#33827=CLOSED_SHELL ( 'NONE', ( #16246, #7814, #24487, #14687, #7838, #21295, #30240, #6219, #24212, #1541 ) ) ;
#33833=ORIENTED_EDGE ( 'NONE', *, *, #29162, .T. ) ;
#33834=DIRECTION ( 'NONE',  ( 0.000000000000000000, 0.000000000000000000, 1.000000000000000000 ) ) ;
#33836=DIRECTION ( 'NONE',  ( 0.000000000000000000, 1.000000000000000000, -3.421138828918010427E-49 ) ) ;
#33838=VERTEX_POINT ( 'NONE', #22873 ) ;
#33841=FACE_OUTER_BOUND ( 'NONE', #30150, .T. ) ;
#33842=AXIS2_PLACEMENT_3D ( 'NONE', #10068, #20923, #31770 ) ;
#33845=VECTOR ( 'NONE', #31252, 1000.000000000000000 ) ;
#33847=FACE_OUTER_BOUND ( 'NONE', #33155, .T. ) ;
#33849=CARTESIAN_POINT ( 'NONE',  ( -355.0000000000000000, -131.0000000000000000, 128.0000000000000000 ) ) ;
#33850=CARTESIAN_POINT ( 'NONE',  ( -499.9999999999999432, -105.0000000000000142, -162.9999999999999716 ) ) ;
#33852=VECTOR ( 'NONE', #20943, 1000.000000000000000 ) ;
#33858=VECTOR ( 'NONE', #23689, 1000.000000000000000 ) ;
#33859=ORIENTED_EDGE ( 'NONE', *, *, #26797, .T. ) ;
#33861=VECTOR ( 'NONE', #28748, 1000.000000000000000 ) ;
#33863=ORIENTED_EDGE ( 'NONE', *, *, #1518, .T. ) ;
#33867=VECTOR ( 'NONE', #20016, 1000.000000000000000 ) ;
#33868=ADVANCED_FACE ( 'NONE', ( #25168 ), #17198, .F. ) ;
#33870=ORIENTED_EDGE ( 'NONE', *, *, #10313, .F. ) ;
#33871=CARTESIAN_POINT ( 'NONE',  ( -12.00000000000001066, -105.0000000000000142, 174.9999999999999432 ) ) ;
#33877=EDGE_CURVE ( 'NONE', #18216, #9649, #14703, .T. ) ;
#33878=AXIS2_PLACEMENT_3D ( 'NONE', #542, #8716, #19413 ) ;
#33881=DIRECTION ( 'NONE',  ( 0.000000000000000000, 0.000000000000000000, -1.000000000000000000 ) ) ;
#33882=FACE_OUTER_BOUND ( 'NONE', #8811, .T. ) ;
#33883=ORIENTED_EDGE ( 'NONE', *, *, #14142, .T. ) ;
#33885=DIRECTION ( 'NONE',  ( -0.000000000000000000, -0.000000000000000000, 1.000000000000000000 ) ) ;
#33888=FACE_BOUND ( 'NONE', #2904, .T. ) ;
#33889=VERTEX_POINT ( 'NONE', #22522 ) ;
#33891=DIRECTION ( 'NONE',  ( -1.000000000000000000, 0.000000000000000000, 0.000000000000000000 ) ) ;
#33897=CARTESIAN_POINT ( 'NONE',  ( -410.0000000000000568, -137.0000000000000000, -155.0000000000000000 ) ) ;
#33903=EDGE_LOOP ( 'NONE', ( #22664, #8517, #13456, #34380 ) ) ;
#33905=VECTOR ( 'NONE', #15926, 1000.000000000000000 ) ;
#33907=ORIENTED_EDGE ( 'NONE', *, *, #30540, .F. ) ;
#33910=ORIENTED_EDGE ( 'NONE', *, *, #29136, .F. ) ;
#33913=DIRECTION ( 'NONE',  ( 0.000000000000000000, -0.000000000000000000, -1.000000000000000000 ) ) ;
#33914=AXIS2_PLACEMENT_3D ( 'NONE', #32636, #21221, #10360 ) ;
#33916=DIRECTION ( 'NONE',  ( 1.000000000000000000, -0.000000000000000000, 0.000000000000000000 ) ) ;
#33918=ORIENTED_EDGE ( 'NONE', *, *, #11590, .F. ) ;
#33920=PLANE ( 'NONE',  #451 ) ;
#33921=CARTESIAN_POINT ( 'NONE',  ( -20.00000000000007461, -113.0000000000000000, -187.0000000000000000 ) ) ;
#33922=EDGE_CURVE ( 'NONE', #7091, #35062, #33366, .T. ) ;
#33923=DIRECTION ( 'NONE',  ( 0.000000000000000000, 1.000000000000000000, 1.224646799147353207E-16 ) ) ;
#33926=LINE ( 'NONE', #6507, #33845 ) ;
#33930=EDGE_LOOP ( 'NONE', ( #24792, #34933, #18680, #2426 ) ) ;
#33935=CARTESIAN_POINT ( 'NONE',  ( -414.0000000000000568, -137.0000000000000000, -155.0000000000000000 ) ) ;
#33937=CARTESIAN_POINT ( 'NONE',  ( -442.0000000000000000, 113.0000000000000000, -175.0000000000000000 ) ) ;
#33939=EDGE_CURVE ( 'NONE', #23404, #32668, #6479, .T. ) ;
#33943=CARTESIAN_POINT ( 'NONE',  ( 19.99999999999996092, -145.0000000000000000, 162.9999999999999716 ) ) ;
#33945=ADVANCED_FACE ( 'NONE', ( #24820 ), #454, .F. ) ;
#33946=ORIENTED_EDGE ( 'NONE', *, *, #4536, .F. ) ;
#33948=ADVANCED_FACE ( 'NONE', ( #23051 ), #23737, .F. ) ;
#33959=ORIENTED_EDGE ( 'NONE', *, *, #15554, .F. ) ;
#33963=VECTOR ( 'NONE', #23885, 1000.000000000000000 ) ;
#33965=CARTESIAN_POINT ( 'NONE',  ( -12.00000000000001066, 136.9999999999999716, -155.0000000000000000 ) ) ;
#33969=CARTESIAN_POINT ( 'NONE',  ( -414.0000000000000568, 124.9999999999999574, -187.0000000000000000 ) ) ;
#33974=DIRECTION ( 'NONE',  ( 0.000000000000000000, 0.000000000000000000, 1.000000000000000000 ) ) ;
#33976=ORIENTED_EDGE ( 'NONE', *, *, #30508, .T. ) ;
#33978=DIRECTION ( 'NONE',  ( 0.000000000000000000, 0.000000000000000000, -1.000000000000000000 ) ) ;
#33979=AXIS2_PLACEMENT_3D ( 'NONE', #429, #29970, #14136 ) ;
#33983=CARTESIAN_POINT ( 'NONE',  ( -12.00000000000001066, 144.9999999999999716, -162.9999999999999432 ) ) ;
#33985=EDGE_CURVE ( 'NONE', #11239, #5234, #6828, .T. ) ;
#33986=CIRCLE ( 'NONE', #16375, 3.999999999999976019 ) ;
#33998=DIRECTION ( 'NONE',  ( -0.000000000000000000, -1.000000000000000000, -0.000000000000000000 ) ) ;
#34000=VECTOR ( 'NONE', #16424, 1000.000000000000000 ) ;
#34004=CARTESIAN_POINT ( 'NONE',  ( 19.99999999999998934, 75.55999999999990280, 172.9900000000000091 ) ) ;
#34006=EDGE_LOOP ( 'NONE', ( #8825, #31239, #14906, #12796 ) ) ;
#34007=CIRCLE ( 'NONE', #18685, 2.000000000000001776 ) ;
#34008=FACE_OUTER_BOUND ( 'NONE', #13007, .T. ) ;
#34012=EDGE_CURVE ( 'NONE', #23038, #26019, #15045, .T. ) ;
#34014=LINE ( 'NONE', #34363, #13158 ) ;
#34015=CARTESIAN_POINT ( 'NONE',  ( -20.00000000000001776, -141.0000000000000000, -162.9999999999999432 ) ) ;
#34017=CARTESIAN_POINT ( 'NONE',  ( -12.00000000000001066, 104.9999999999999858, 154.9999999999999432 ) ) ;
#34018=DIRECTION ( 'NONE',  ( 0.000000000000000000, 1.000000000000000000, 5.053935297177146739E-49 ) ) ;
#34019=CARTESIAN_POINT ( 'NONE',  ( -449.9999999999999432, -137.0000000000000000, -175.0000000000000000 ) ) ;
#34022=CARTESIAN_POINT ( 'NONE',  ( -19.99999999999998934, -137.0000000000000000, -155.0000000000000284 ) ) ;
#34024=AXIS2_PLACEMENT_3D ( 'NONE', #33613, #28103, #6379 ) ;
#34027=VECTOR ( 'NONE', #1531, 1000.000000000000000 ) ;
#34029=ADVANCED_FACE ( 'NONE', ( #23222 ), #9684, .F. ) ;
#34031=ORIENTED_EDGE ( 'NONE', *, *, #14480, .T. ) ;
#34032=AXIS2_PLACEMENT_3D ( 'NONE', #15849, #2813, #2987 ) ;
#34033=DIRECTION ( 'NONE',  ( -1.000000000000000000, 0.000000000000000000, 0.000000000000000000 ) ) ;
#34036=EDGE_LOOP ( 'NONE', ( #1345, #30536, #16356, #26363, #6577, #1549, #16816, #672 ) ) ;
#34037=DIRECTION ( 'NONE',  ( 1.000000000000000000, 3.040835319149746528E-31, 1.232595164407830946E-32 ) ) ;
#34040=CARTESIAN_POINT ( 'NONE',  ( -70.00000000000000000, 75.55999999999990280, -168.2400000000000091 ) ) ;
#34041=CARTESIAN_POINT ( 'NONE',  ( -418.0000000000000000, 105.0000000000000142, -175.0000000000000000 ) ) ;
#34042=VERTEX_POINT ( 'NONE', #23386 ) ;
#34046=DIRECTION ( 'NONE',  ( 1.000000000000000000, -0.000000000000000000, -0.000000000000000000 ) ) ;
#34053=CARTESIAN_POINT ( 'NONE',  ( -19.99999999999998934, -112.9999999999999858, -155.0000000000000284 ) ) ;
#34057=DIRECTION ( 'NONE',  ( 1.000000000000000000, 0.000000000000000000, 0.000000000000000000 ) ) ;
#34060=DIRECTION ( 'NONE',  ( 0.000000000000000000, 0.000000000000000000, 1.000000000000000000 ) ) ;
#34062=VECTOR ( 'NONE', #13999, 1000.000000000000000 ) ;
#34064=DIRECTION ( 'NONE',  ( 0.000000000000000000, -1.000000000000000000, 6.123233995736766036E-17 ) ) ;
#34069=EDGE_CURVE ( 'NONE', #1594, #17242, #15925, .T. ) ;
#34080=CARTESIAN_POINT ( 'NONE',  ( -12.00000000000001066, -32.99999999999997158, -154.9999999999999716 ) ) ;
#34083=DIRECTION ( 'NONE',  ( 0.000000000000000000, -1.000000000000000000, 3.374343856708137958E-53 ) ) ;
#34084=CARTESIAN_POINT ( 'NONE',  ( 11.99999999999999645, 136.9999999999999716, -155.0000000000000000 ) ) ;
#34088=LINE ( 'NONE', #31083, #4385 ) ;
#34092=ORIENTED_EDGE ( 'NONE', *, *, #33723, .F. ) ;
#34093=AXIS2_PLACEMENT_3D ( 'NONE', #31214, #28545, #26208 ) ;
#34099=CYLINDRICAL_SURFACE ( 'NONE', #34252, 4.750000000000004441 ) ;
#34100=ORIENTED_EDGE ( 'NONE', *, *, #29932, .F. ) ;
#34101=CARTESIAN_POINT ( 'NONE',  ( -12.00000000000001243, 134.9999999999998863, 194.9999999999999716 ) ) ;
#34108=LINE ( 'NONE', #33769, #13966 ) ;
#34109=EDGE_CURVE ( 'NONE', #10000, #10965, #32087, .T. ) ;
#34110=ORIENTED_EDGE ( 'NONE', *, *, #8060, .T. ) ;
#34112=EDGE_CURVE ( 'NONE', #7548, #22615, #12672, .T. ) ;
#34113=EDGE_CURVE ( 'NONE', #16065, #22434, #5200, .T. ) ;
#34115=ORIENTED_EDGE ( 'NONE', *, *, #19256, .T. ) ;
#34119=CARTESIAN_POINT ( 'NONE',  ( -418.0000000000000000, -124.9999999999999716, 132.0000000000000000 ) ) ;
#34120=CARTESIAN_POINT ( 'NONE',  ( -12.00000000000001066, -145.0000000000000000, 174.9999999999999432 ) ) ;
#34121=DIRECTION ( 'NONE',  ( 0.000000000000000000, 1.131431318426415506E-52, 1.000000000000000000 ) ) ;
#34124=VERTEX_POINT ( 'NONE', #29432 ) ;
#34125=ORIENTED_EDGE ( 'NONE', *, *, #31936, .F. ) ;
#34126=CARTESIAN_POINT ( 'NONE',  ( -349.0000000000000000, -135.0000000000000000, 128.0000000000000000 ) ) ;
#34129=DIRECTION ( 'NONE',  ( 0.000000000000000000, 0.000000000000000000, -1.000000000000000000 ) ) ;
#34131=LINE ( 'NONE', #34669, #16912 ) ;
#34132=CARTESIAN_POINT ( 'NONE',  ( -349.0000000000000000, -135.0000000000000000, 130.0000000000000000 ) ) ;
#34138=ORIENTED_EDGE ( 'NONE', *, *, #25635, .F. ) ;
#34140=EDGE_CURVE ( 'NONE', #26810, #2032, #14384, .T. ) ;
#34144=CARTESIAN_POINT ( 'NONE',  ( -500.0000000000000000, -109.0000000000000142, 187.0000000000000000 ) ) ;
#34146=CIRCLE ( 'NONE', #18819, 7.999999999999979572 ) ;
#34147=AXIS2_PLACEMENT_3D ( 'NONE', #17943, #4370, #28944 ) ;
#34151=DIRECTION ( 'NONE',  ( 1.232595164407830946E-32, 0.000000000000000000, 1.000000000000000000 ) ) ;
#34152=VERTEX_POINT ( 'NONE', #16446 ) ;
#34153=ORIENTED_EDGE ( 'NONE', *, *, #8706, .T. ) ;
#34154=EDGE_CURVE ( 'NONE', #23829, #18049, #29774, .T. ) ;
#34155=ADVANCED_FACE ( 'NONE', ( #13766 ), #2716, .F. ) ;
#34160=CIRCLE ( 'NONE', #23911, 3.999999999999976019 ) ;
#34161=CARTESIAN_POINT ( 'NONE',  ( -361.0000000000000000, -135.0000000000000000, 112.0000000000000000 ) ) ;
#34173=FACE_OUTER_BOUND ( 'NONE', #7376, .T. ) ;
#34176=CIRCLE ( 'NONE', #18851, 2.000000000000001776 ) ;
#34181=EDGE_CURVE ( 'NONE', #27122, #9925, #16641, .T. ) ;
#34182=CARTESIAN_POINT ( 'NONE',  ( -442.0000000000000000, 113.0000000000000000, 154.9999999999999716 ) ) ;
#34185=FACE_OUTER_BOUND ( 'NONE', #24644, .T. ) ;
#34190=DIRECTION ( 'NONE',  ( 0.000000000000000000, -1.000000000000000000, 0.000000000000000000 ) ) ;
#34193=DIRECTION ( 'NONE',  ( 0.000000000000000000, 1.000000000000000000, 5.053935297177146739E-49 ) ) ;
#34194=ADVANCED_FACE ( 'NONE', ( #414 ), #33327, .T. ) ;
#34196=CARTESIAN_POINT ( 'NONE',  ( -15.99999999999998579, -32.99999999999997158, 154.9999999999999716 ) ) ;
#34199=ORIENTED_EDGE ( 'NONE', *, *, #29581, .F. ) ;
#34200=AXIS2_PLACEMENT_3D ( 'NONE', #28420, #3667, #25739 ) ;
#34201=AXIS2_PLACEMENT_3D ( 'NONE', #29872, #11186, #32520 ) ;
#34206=CYLINDRICAL_SURFACE ( 'NONE', #18187, 4.750000000000004441 ) ;
#34208=ORIENTED_EDGE ( 'NONE', *, *, #30493, .T. ) ;
#34209=ORIENTED_EDGE ( 'NONE', *, *, #34600, .T. ) ;
#34215=DIRECTION ( 'NONE',  ( 0.000000000000000000, 0.000000000000000000, 1.000000000000000000 ) ) ;
#34223=DIRECTION ( 'NONE',  ( 0.000000000000000000, 2.309213040847544338E-50, 1.000000000000000000 ) ) ;
#34224=CARTESIAN_POINT ( 'NONE',  ( -499.9999999999999432, 104.9999999999999858, -187.0000000000000000 ) ) ;
#34226=ADVANCED_FACE ( 'NONE', ( #32958, #25312 ), #33145, .T. ) ;
#34227=VECTOR ( 'NONE', #30212, 1000.000000000000000 ) ;
#34230=ADVANCED_FACE ( 'NONE', ( #30663 ), #16982, .F. ) ;
#34232=LINE ( 'NONE', #34053, #29552 ) ;
#34234=VECTOR ( 'NONE', #13145, 1000.000000000000000 ) ;
#34237=DIRECTION ( 'NONE',  ( 1.232595164407830946E-32, 0.000000000000000000, 1.000000000000000000 ) ) ;
#34238=DIRECTION ( 'NONE',  ( 0.000000000000000000, 1.000000000000000000, 5.145227585319922065E-49 ) ) ;
#34240=CARTESIAN_POINT ( 'NONE',  ( -70.00000000000000000, 4.559999999999908127, 172.9900000000000091 ) ) ;
#34241=ORIENTED_EDGE ( 'NONE', *, *, #5875, .T. ) ;
#34245=VERTEX_POINT ( 'NONE', #11628 ) ;
#34252=AXIS2_PLACEMENT_3D ( 'NONE', #28592, #3494, #6691 ) ;
#34253=ORIENTED_EDGE ( 'NONE', *, *, #10275, .F. ) ;
#34256=ORIENTED_EDGE ( 'NONE', *, *, #13585, .F. ) ;
#34257=DIRECTION ( 'NONE',  ( 1.000000000000000000, 3.469446951953834515E-18, 0.000000000000000000 ) ) ;
#34259=PLANE ( 'NONE',  #33004 ) ;
#34264=FACE_OUTER_BOUND ( 'NONE', #25919, .T. ) ;
#34266=LINE ( 'NONE', #33562, #15298 ) ;
#34275=DIRECTION ( 'NONE',  ( -1.000000000000000000, -3.040835319149746528E-31, -1.232595164407830946E-32 ) ) ;
#34279=VECTOR ( 'NONE', #20586, 1000.000000000000000 ) ;
#34280=AXIS2_PLACEMENT_3D ( 'NONE', #14254, #3022, #19597 ) ;
#34286=ADVANCED_FACE ( 'NONE', ( #17848 ), #28513, .F. ) ;
#34287=ORIENTED_EDGE ( 'NONE', *, *, #16602, .T. ) ;
#34288=DIRECTION ( 'NONE',  ( 0.000000000000000000, -1.000000000000000000, 6.842277657836020854E-49 ) ) ;
#34293=ORIENTED_EDGE ( 'NONE', *, *, #23967, .F. ) ;
#34295=ORIENTED_EDGE ( 'NONE', *, *, #28565, .F. ) ;
#34298=DIRECTION ( 'NONE',  ( 0.000000000000000000, 1.000000000000000000, 1.224646799147353207E-16 ) ) ;
#34303=VERTEX_POINT ( 'NONE', #4108 ) ;
#34308=CARTESIAN_POINT ( 'NONE',  ( -442.0000000000000000, 104.9999999999999858, -155.0000000000000000 ) ) ;
#34309=DIRECTION ( 'NONE',  ( 0.000000000000000000, -1.310824597558155437E-49, -1.000000000000000000 ) ) ;
#34313=VERTEX_POINT ( 'NONE', #34022 ) ;
#34314=EDGE_CURVE ( 'NONE', #32798, #7621, #12157, .T. ) ;
#34319=AXIS2_PLACEMENT_3D ( 'NONE', #21520, #7973, #29698 ) ;
#34323=VERTEX_POINT ( 'NONE', #1627 ) ;
#34325=ADVANCED_FACE ( 'NONE', ( #9646 ), #6788, .T. ) ;
#34326=DIRECTION ( 'NONE',  ( 1.000000000000000000, 0.000000000000000000, -1.300283923313630633E-47 ) ) ;
#34332=LINE ( 'NONE', #1073, #21721 ) ;
#34334=EDGE_CURVE ( 'NONE', #23007, #6336, #26012, .T. ) ;
#34335=EDGE_LOOP ( 'NONE', ( #19661, #241, #17367, #20486, #9867, #1814, #20302, #26901 ) ) ;
#34337=ORIENTED_EDGE ( 'NONE', *, *, #901, .F. ) ;
#34342=ORIENTED_EDGE ( 'NONE', *, *, #13691, .F. ) ;
#34343=MANIFOLD_SOLID_BREP ( 'Boss-Extrude6[2]', #20200 ) ;
#34345=CIRCLE ( 'NONE', #6492, 4.000000000000003553 ) ;
#34349=CIRCLE ( 'NONE', #15061, 3.999999999999976019 ) ;
#34350=VERTEX_POINT ( 'NONE', #6610 ) ;
#34356=LINE ( 'NONE', #23678, #8585 ) ;
#34357=ORIENTED_EDGE ( 'NONE', *, *, #33985, .F. ) ;
#34363=CARTESIAN_POINT ( 'NONE',  ( -500.0000000000000000, 144.9999999999999716, -155.0000000000000000 ) ) ;
#34364=CARTESIAN_POINT ( 'NONE',  ( -361.0000000000000000, 124.9999999999999432, 181.0000000000000000 ) ) ;
#34367=CIRCLE ( 'NONE', #19598, 2.000000000000001776 ) ;
#34371=DIRECTION ( 'NONE',  ( -1.000000000000000000, 0.000000000000000000, -0.000000000000000000 ) ) ;
#34373=EDGE_CURVE ( 'NONE', #18350, #19066, #22340, .T. ) ;
#34374=VECTOR ( 'NONE', #14548, 1000.000000000000000 ) ;
#34380=ORIENTED_EDGE ( 'NONE', *, *, #31549, .F. ) ;
#34387=ORIENTED_EDGE ( 'NONE', *, *, #14292, .T. ) ;
#34388=CARTESIAN_POINT ( 'NONE',  ( -430.0000000000000000, 134.9999999999999716, 126.0000000000000000 ) ) ;
#34392=ORIENTED_EDGE ( 'NONE', *, *, #32176, .T. ) ;
#34393=DIRECTION ( 'NONE',  ( 0.000000000000000000, -1.000000000000000000, -5.145227585319922065E-49 ) ) ;
#34396=ORIENTED_EDGE ( 'NONE', *, *, #1394, .F. ) ;
#34397=CYLINDRICAL_SURFACE ( 'NONE', #16887, 3.999999999999976019 ) ;
#34399=DIRECTION ( 'NONE',  ( 1.000000000000000000, 0.000000000000000000, 0.000000000000000000 ) ) ;
#34403=CARTESIAN_POINT ( 'NONE',  ( -12.00000000000001066, 140.9999999999999716, 155.0000000000000000 ) ) ;
#34404=ORIENTED_EDGE ( 'NONE', *, *, #10768, .T. ) ;
#34409=DIRECTION ( 'NONE',  ( 1.000000000000000000, 0.000000000000000000, -5.546364386991661285E-52 ) ) ;
#34412=CYLINDRICAL_SURFACE ( 'NONE', #28278, 7.999999999999979572 ) ;
#34413=CARTESIAN_POINT ( 'NONE',  ( -499.9999999999999432, 144.9999999999999716, -162.9999999999999716 ) ) ;
#34414=FACE_OUTER_BOUND ( 'NONE', #27744, .T. ) ;
#34415=CARTESIAN_POINT ( 'NONE',  ( 11.99999999999999645, -124.9999999999999432, -194.9999999999999432 ) ) ;
#34420=FACE_OUTER_BOUND ( 'NONE', #10792, .T. ) ;
#34423=AXIS2_PLACEMENT_3D ( 'NONE', #5787, #16684, #27519 ) ;
#34428=EDGE_CURVE ( 'NONE', #25965, #9066, #6979, .T. ) ;
#34435=DIRECTION ( 'NONE',  ( -1.000000000000000000, 0.000000000000000000, 0.000000000000000000 ) ) ;
#34436=CIRCLE ( 'NONE', #905, 4.750000000000004441 ) ;
#34439=ORIENTED_EDGE ( 'NONE', *, *, #27071, .T. ) ;
#34440=EDGE_LOOP ( 'NONE', ( #18001, #10863, #3064, #18987 ) ) ;
#34441=LINE ( 'NONE', #1861, #33861 ) ;
#34442=CARTESIAN_POINT ( 'NONE',  ( 11.99999999999999645, 134.9999999999998863, 194.9999999999999716 ) ) ;
#34444=DIRECTION ( 'NONE',  ( -1.000000000000000000, 0.000000000000000000, 1.848892746611746966E-32 ) ) ;
#34446=ORIENTED_EDGE ( 'NONE', *, *, #418, .F. ) ;
#34448=DIRECTION ( 'NONE',  ( -1.000000000000000000, -3.040835319149746528E-31, -1.232595164407830946E-32 ) ) ;
#34449=CARTESIAN_POINT ( 'NONE',  ( -12.00000000000003908, -145.0000000000000000, -154.9999999999999716 ) ) ;
#34450=ORIENTED_EDGE ( 'NONE', *, *, #22152, .F. ) ;
#34458=ORIENTED_EDGE ( 'NONE', *, *, #22798, .T. ) ;
#34462=CIRCLE ( 'NONE', #28772, 7.999999999999979572 ) ;
#34466=DIRECTION ( 'NONE',  ( 1.000000000000000000, 0.000000000000000000, 0.000000000000000000 ) ) ;
#34468=EDGE_LOOP ( 'NONE', ( #29710, #27951, #10919, #33715 ) ) ;
#34469=VECTOR ( 'NONE', #5008, 1000.000000000000000 ) ;
#34474=EDGE_CURVE ( 'NONE', #31695, #5771, #5157, .T. ) ;
#34475=ORIENTED_EDGE ( 'NONE', *, *, #22711, .F. ) ;
#34488=CARTESIAN_POINT ( 'NONE',  ( -418.0000000000000000, 105.0000000000000142, -109.9999999999999574 ) ) ;
#34490=DIRECTION ( 'NONE',  ( 0.000000000000000000, 1.000000000000000000, 5.053935297177146739E-49 ) ) ;
#34491=ORIENTED_EDGE ( 'NONE', *, *, #31891, .F. ) ;
#34496=CARTESIAN_POINT ( 'NONE',  ( -499.9999999999998863, -109.0000000000000142, -162.9999999999999716 ) ) ;
#34504=EDGE_CURVE ( 'NONE', #28875, #31191, #10707, .T. ) ;
#34506=CYLINDRICAL_SURFACE ( 'NONE', #16801, 3.999999999999976019 ) ;
#34509=ORIENTED_EDGE ( 'NONE', *, *, #3289, .F. ) ;
#34514=AXIS2_PLACEMENT_3D ( 'NONE', #23933, #11304, #19150 ) ;
#34516=VECTOR ( 'NONE', #27006, 1000.000000000000000 ) ;
#34518=DIRECTION ( 'NONE',  ( 0.000000000000000000, 2.309213040847544338E-50, 1.000000000000000000 ) ) ;
#34520=ADVANCED_FACE ( 'NONE', ( #23693 ), #32749, .F. ) ;
#34521=VERTEX_POINT ( 'NONE', #11047 ) ;
#34523=EDGE_CURVE ( 'NONE', #17865, #32956, #22433, .T. ) ;
#34527=DIRECTION ( 'NONE',  ( -0.000000000000000000, 1.000000000000000000, -0.000000000000000000 ) ) ;
#34532=CARTESIAN_POINT ( 'NONE',  ( -12.00000000000001066, -145.0000000000000000, -194.9999999999999432 ) ) ;
#34533=CARTESIAN_POINT ( 'NONE',  ( 11.99999999999999645, -105.0000000000000142, 155.0000000000000000 ) ) ;
#34534=EDGE_LOOP ( 'NONE', ( #18540, #32714, #20433, #30804 ) ) ;
#34535=CARTESIAN_POINT ( 'NONE',  ( -430.0000000000000000, 116.9999999999999858, 126.0000000000000000 ) ) ;
#34537=ORIENTED_EDGE ( 'NONE', *, *, #30540, .T. ) ;
#34553=ORIENTED_EDGE ( 'NONE', *, *, #24368, .F. ) ;
#34555=ADVANCED_FACE ( 'NONE', ( #22614, #32922, #33099 ), #372, .T. ) ;
#34556=VECTOR ( 'NONE', #9128, 1000.000000000000000 ) ;
#34559=EDGE_CURVE ( 'NONE', #31620, #15103, #2847, .T. ) ;
#34561=VERTEX_POINT ( 'NONE', #25081 ) ;
#34570=DIRECTION ( 'NONE',  ( 0.000000000000000000, -3.374343856708137958E-53, 1.000000000000000000 ) ) ;
#34577=CARTESIAN_POINT ( 'NONE',  ( 15.99999999999998579, -124.9999999999999432, -162.9999999999999432 ) ) ;
#34578=ADVANCED_FACE ( 'NONE', ( #24548 ), #30256, .F. ) ;
#34579=FACE_OUTER_BOUND ( 'NONE', #13815, .T. ) ;
#34580=ORIENTED_EDGE ( 'NONE', *, *, #6730, .T. ) ;
#34581=AXIS2_PLACEMENT_3D ( 'NONE', #26199, #9662, #31206 ) ;
#34583=CYLINDRICAL_SURFACE ( 'NONE', #28735, 8.000000000000007105 ) ;
#34584=MANIFOLD_SOLID_BREP ( 'Trim/Extend6[2]', #4816 ) ;
#34588=VECTOR ( 'NONE', #25639, 1000.000000000000000 ) ;
#34589=DIRECTION ( 'NONE',  ( 1.000000000000000000, 0.000000000000000000, -1.848892746611746966E-32 ) ) ;
#34592=EDGE_CURVE ( 'NONE', #10121, #28865, #30442, .T. ) ;
#34594=ADVANCED_FACE ( 'NONE', ( #11584 ), #33283, .T. ) ;
#34595=LINE ( 'NONE', #15556, #4758 ) ;
#34600=EDGE_CURVE ( 'NONE', #34561, #25561, #14355, .T. ) ;
#34601=VERTEX_POINT ( 'NONE', #31308 ) ;
#34602=CARTESIAN_POINT ( 'NONE',  ( -442.0000000000000000, -109.0000000000000142, -174.9999999999999716 ) ) ;
#34607=EDGE_CURVE ( 'NONE', #18155, #5682, #26238, .T. ) ;
#34608=ORIENTED_EDGE ( 'NONE', *, *, #30823, .T. ) ;
#34610=ORIENTED_EDGE ( 'NONE', *, *, #209, .F. ) ;
#34612=LINE ( 'NONE', #21075, #12213 ) ;
#34614=DIRECTION ( 'NONE',  ( 0.000000000000000000, 0.000000000000000000, -1.000000000000000000 ) ) ;
#34615=FACE_OUTER_BOUND ( 'NONE', #34440, .T. ) ;
#34617=ORIENTED_EDGE ( 'NONE', *, *, #13869, .T. ) ;
#34618=CARTESIAN_POINT ( 'NONE',  ( -500.0000000000000000, -137.0000000000000000, 159.0000000000000000 ) ) ;
#34619=DIRECTION ( 'NONE',  ( 1.000000000000000000, 0.000000000000000000, 0.000000000000000000 ) ) ;
#34628=CARTESIAN_POINT ( 'NONE',  ( -355.0000000000000000, -133.0000000000000000, 126.0000000000000000 ) ) ;
#34631=ORIENTED_EDGE ( 'NONE', *, *, #19184, .F. ) ;
#34632=AXIS2_PLACEMENT_3D ( 'NONE', #2393, #24444, #21274 ) ;
#34634=LINE ( 'NONE', #2400, #25148 ) ;
#34635=EDGE_LOOP ( 'NONE', ( #5042, #10592, #1458, #29076 ) ) ;
#34636=EDGE_CURVE ( 'NONE', #19987, #13518, #7087, .T. ) ;
#34637=PLANE ( 'NONE',  #32006 ) ;
#34641=EDGE_CURVE ( 'NONE', #18838, #11597, #28470, .T. ) ;
#34642=VECTOR ( 'NONE', #9501, 1000.000000000000000 ) ;
#34645=LINE ( 'NONE', #10254, #27950 ) ;
#34646=EDGE_CURVE ( 'NONE', #22648, #8601, #34332, .T. ) ;
#34652=CARTESIAN_POINT ( 'NONE',  ( -361.0000000000000000, -135.0000000000000000, 112.0000000000000000 ) ) ;
#34653=ORIENTED_EDGE ( 'NONE', *, *, #31366, .T. ) ;
#34661=VERTEX_POINT ( 'NONE', #22961 ) ;
#34663=ADVANCED_FACE ( 'NONE', ( #25793 ), #1242, .T. ) ;
#34666=CARTESIAN_POINT ( 'NONE',  ( -20.00000000000004619, 136.9999999999999432, 155.0000000000000000 ) ) ;
#34667=AXIS2_PLACEMENT_3D ( 'NONE', #25288, #8921, #14280 ) ;
#34668=DIRECTION ( 'NONE',  ( -1.000000000000000000, 0.000000000000000000, -1.300283923313630633E-47 ) ) ;
#34669=CARTESIAN_POINT ( 'NONE',  ( 19.99999999999996092, -134.9999999999999716, -162.9999999999999432 ) ) ;
#34674=ADVANCED_FACE ( 'NONE', ( #1760, #12116 ), #31148, .T. ) ;
#34675=CARTESIAN_POINT ( 'NONE',  ( -418.0000000000000000, 144.9999999999999716, 154.9999999999999716 ) ) ;
#34676=ORIENTED_EDGE ( 'NONE', *, *, #17822, .T. ) ;
#34677=EDGE_CURVE ( 'NONE', #19207, #18227, #19456, .T. ) ;
#34679=EDGE_LOOP ( 'NONE', ( #29380, #29487, #5958, #31820 ) ) ;
#34681=AXIS2_PLACEMENT_3D ( 'NONE', #10347, #26893, #2506 ) ;
#34686=ORIENTED_EDGE ( 'NONE', *, *, #11551, .T. ) ;
#34687=VERTEX_POINT ( 'NONE', #6913 ) ;
#34691=DIRECTION ( 'NONE',  ( 0.000000000000000000, 0.000000000000000000, 1.000000000000000000 ) ) ;
#34693=DIRECTION ( 'NONE',  ( 1.000000000000000000, 0.000000000000000000, 5.546364386991661285E-52 ) ) ;
#34697=MANIFOLD_SOLID_BREP ( 'Square tube 40 X 40 X 4(1)[10]', #2561 ) ;
#34703=EDGE_LOOP ( 'NONE', ( #33330, #13092, #11721, #9543 ) ) ;
#34704=LINE ( 'NONE', #2297, #2072 ) ;
#34705=EDGE_CURVE ( 'NONE', #15586, #24825, #25615, .T. ) ;
#34708=CARTESIAN_POINT ( 'NONE',  ( -20.00000000000007461, -113.0000000000000000, -155.0000000000000000 ) ) ;
#34709=DIRECTION ( 'NONE',  ( 0.000000000000000000, 1.000000000000000000, 5.053935297177146739E-49 ) ) ;
#34711=CARTESIAN_POINT ( 'NONE',  ( -361.0000000000000000, -125.0000000000000284, 113.9999999999999858 ) ) ;
#34712=EDGE_CURVE ( 'NONE', #28310, #2702, #26669, .T. ) ;
#34713=VECTOR ( 'NONE', #11610, 1000.000000000000000 ) ;
#34716=EDGE_LOOP ( 'NONE', ( #2552, #4759, #31993, #24899 ) ) ;
#34719=( LENGTH_UNIT ( ) NAMED_UNIT ( * ) SI_UNIT ( .MILLI., .METRE. ) );
#34723=DIRECTION ( 'NONE',  ( -0.000000000000000000, 1.000000000000000000, 0.000000000000000000 ) ) ;
#34727=EDGE_CURVE ( 'NONE', #25708, #3173, #21514, .T. ) ;
#34728=AXIS2_PLACEMENT_3D ( 'NONE', #33207, #25187, #9010 ) ;
#34729=ORIENTED_EDGE ( 'NONE', *, *, #17932, .F. ) ;
#34733=ADVANCED_BREP_SHAPE_REPRESENTATION ( '', ( #21945, #34697, #22717, #100, #10767, #11835, #12482, #24685, #11234, #22940, #10172, #22535, #34343, #23516, #10344, #34584, #11180, #1117, #28566 ), #4098 ) ;
#34737=VECTOR ( 'NONE', #26492, 1000.000000000000000 ) ;
#34738=ORIENTED_EDGE ( 'NONE', *, *, #28166, .T. ) ;
#34740=VERTEX_POINT ( 'NONE', #2633 ) ;
#34746=ORIENTED_EDGE ( 'NONE', *, *, #25574, .T. ) ;
#34751=EDGE_CURVE ( 'NONE', #10828, #8531, #17760, .T. ) ;
#34758=LINE ( 'NONE', #7330, #21925 ) ;
#34766=AXIS2_PLACEMENT_3D ( 'NONE', #30280, #14460, #567 ) ;
#34769=CIRCLE ( 'NONE', #1803, 7.999999999999986677 ) ;
#34771=CIRCLE ( 'NONE', #31356, 7.999999999999979572 ) ;
#34773=CARTESIAN_POINT ( 'NONE',  ( -15.99999999999998579, -145.0000000000000000, -186.9999999999999716 ) ) ;
#34777=ORIENTED_EDGE ( 'NONE', *, *, #19098, .T. ) ;
#34778=SHAPE_REPRESENTATION_RELATIONSHIP ( 'NONE' , 'NONE' ,  #47, #34733 ) ;
#34784=EDGE_LOOP ( 'NONE', ( #26128, #29223, #30652, #10346 ) ) ;
#34785=ORIENTED_EDGE ( 'NONE', *, *, #25045, .F. ) ;
#34786=LINE ( 'NONE', #18602, #24700 ) ;
#34789=DIRECTION ( 'NONE',  ( -1.000000000000000000, 0.000000000000000000, 1.848892746611746966E-32 ) ) ;
#34790=EDGE_CURVE ( 'NONE', #2780, #13396, #5117, .T. ) ;
#34791=AXIS2_PLACEMENT_3D ( 'NONE', #10645, #18498, #7249 ) ;
#34792=DIRECTION ( 'NONE',  ( -0.000000000000000000, -0.000000000000000000, -1.000000000000000000 ) ) ;
#34793=ORIENTED_EDGE ( 'NONE', *, *, #5518, .T. ) ;
#34795=AXIS2_PLACEMENT_3D ( 'NONE', #16668, #27674, #3112 ) ;
#34799=LINE ( 'NONE', #13089, #12419 ) ;
#34801=CARTESIAN_POINT ( 'NONE',  ( -445.9999999999999432, -105.0000000000000142, 107.9999999999999858 ) ) ;
#34803=CARTESIAN_POINT ( 'NONE',  ( -345.0000000000000000, 134.9999999999999716, 126.0000000000000000 ) ) ;
#34808=LINE ( 'NONE', #12282, #19744 ) ;
#34809=VERTEX_POINT ( 'NONE', #29350 ) ;
#34810=CARTESIAN_POINT ( 'NONE',  ( 12.00000000000001066, -60.99999999999997158, 154.9999999999999716 ) ) ;
#34813=ADVANCED_FACE ( 'NONE', ( #13157 ), #10483, .F. ) ;
#34815=CLOSED_SHELL ( 'NONE', ( #31937, #13035, #7493, #23229, #14079, #31575, #2318, #32571, #7996, #10860, #33760, #35082, #12948, #23944, #2080, #1746, #35043, #7991 ) ) ;
#34822=VECTOR ( 'NONE', #33891, 1000.000000000000000 ) ;
#34825=VECTOR ( 'NONE', #20584, 1000.000000000000000 ) ;
#34827=CARTESIAN_POINT ( 'NONE',  ( -414.0000000000000568, 113.0000000000000000, -175.0000000000000000 ) ) ;
#34828=ORIENTED_EDGE ( 'NONE', *, *, #13691, .T. ) ;
#34830=ORIENTED_EDGE ( 'NONE', *, *, #10566, .F. ) ;
#34831=DIRECTION ( 'NONE',  ( -0.000000000000000000, -1.000000000000000000, -0.000000000000000000 ) ) ;
#34832=ORIENTED_EDGE ( 'NONE', *, *, #25835, .F. ) ;
#34833=DIRECTION ( 'NONE',  ( 1.000000000000000000, 0.000000000000000000, 0.000000000000000000 ) ) ;
#34835=EDGE_CURVE ( 'NONE', #27012, #4827, #697, .T. ) ;
#34836=DIRECTION ( 'NONE',  ( 0.000000000000000000, -1.000000000000000000, -1.310824597558155437E-49 ) ) ;
#34837=EDGE_CURVE ( 'NONE', #34245, #13771, #27022, .T. ) ;
#34839=DIRECTION ( 'NONE',  ( 1.300283923313630633E-47, 0.000000000000000000, -1.000000000000000000 ) ) ;
#34841=EDGE_LOOP ( 'NONE', ( #6811, #3043, #31576, #16535 ) ) ;
#34843=EDGE_LOOP ( 'NONE', ( #32144, #27081, #11254, #10042 ) ) ;
#34846=EDGE_CURVE ( 'NONE', #24518, #32005, #21852, .T. ) ;
#34847=DIRECTION ( 'NONE',  ( 0.000000000000000000, -1.000000000000000000, -2.465190328815662439E-32 ) ) ;
#34850=ADVANCED_FACE ( 'NONE', ( #8503 ), #19552, .T. ) ;
#34855=AXIS2_PLACEMENT_3D ( 'NONE', #32429, #8047, #24243 ) ;
#34856=CARTESIAN_POINT ( 'NONE',  ( -442.0000000000000000, -141.0000000000000000, -175.0000000000000000 ) ) ;
#34857=ORIENTED_EDGE ( 'NONE', *, *, #17901, .F. ) ;
#34858=LINE ( 'NONE', #19014, #33308 ) ;
#34867=VECTOR ( 'NONE', #29814, 1000.000000000000000 ) ;
#34868=ORIENTED_EDGE ( 'NONE', *, *, #2870, .T. ) ;
#34880=EDGE_CURVE ( 'NONE', #32120, #34561, #32708, .T. ) ;
#34883=CARTESIAN_POINT ( 'NONE',  ( -410.0000000000000568, -104.9999999999999005, -77.99999999999997158 ) ) ;
#34884=FACE_BOUND ( 'NONE', #5661, .T. ) ;
#34886=DIRECTION ( 'NONE',  ( 0.000000000000000000, -1.000000000000000000, -2.465190328815662439E-32 ) ) ;
#34887=AXIS2_PLACEMENT_3D ( 'NONE', #32713, #2983, #32885 ) ;
#34891=ORIENTED_EDGE ( 'NONE', *, *, #8634, .F. ) ;
#34893=ORIENTED_EDGE ( 'NONE', *, *, #20893, .T. ) ;
#34894=CARTESIAN_POINT ( 'NONE',  ( -361.0000000000000000, -125.0000000000000284, 166.9999999999999716 ) ) ;
#34895=CARTESIAN_POINT ( 'NONE',  ( -349.0000000000000000, -125.0000000000000284, 109.9999999999999858 ) ) ;
#34904=DIRECTION ( 'NONE',  ( 1.000000000000000000, 3.040835319149746090E-31, 1.232595164407830946E-32 ) ) ;
#34905=DIRECTION ( 'NONE',  ( 0.000000000000000000, 0.000000000000000000, 1.000000000000000000 ) ) ;
#34906=CARTESIAN_POINT ( 'NONE',  ( 15.99999999999998579, 4.559999999999908127, -172.9900000000000091 ) ) ;
#34907=DIRECTION ( 'NONE',  ( 0.000000000000000000, 1.000000000000000000, 5.053935297177146739E-49 ) ) ;
#34909=LINE ( 'NONE', #6955, #25068 ) ;
#34910=DIRECTION ( 'NONE',  ( 0.000000000000000000, 0.000000000000000000, -1.000000000000000000 ) ) ;
#34912=VECTOR ( 'NONE', #12082, 1000.000000000000000 ) ;
#34918=VECTOR ( 'NONE', #1605, 1000.000000000000000 ) ;
#34919=ORIENTED_EDGE ( 'NONE', *, *, #23046, .T. ) ;
#34927=EDGE_CURVE ( 'NONE', #14045, #35, #8327, .T. ) ;
#34929=LINE ( 'NONE', #25723, #13034 ) ;
#34930=AXIS2_PLACEMENT_3D ( 'NONE', #32965, #27466, #3077 ) ;
#34933=ORIENTED_EDGE ( 'NONE', *, *, #22548, .F. ) ;
#34937=CARTESIAN_POINT ( 'NONE',  ( -430.0000000000000000, -133.0000000000000000, 113.9999999999999858 ) ) ;
#34938=PLANE ( 'NONE',  #19959 ) ;
#34942=CARTESIAN_POINT ( 'NONE',  ( -442.0000000000000000, -137.0000000000000000, -175.0000000000000000 ) ) ;
#34943=CIRCLE ( 'NONE', #25829, 3.999999999999976019 ) ;
#34944=CARTESIAN_POINT ( 'NONE',  ( -361.0000000000000000, -125.0000000000000284, 164.9999999999999716 ) ) ;
#34945=CARTESIAN_POINT ( 'NONE',  ( 12.00000000000001066, -134.9999999999999716, 162.9999999999999716 ) ) ;
#34946=FACE_OUTER_BOUND ( 'NONE', #31378, .T. ) ;
#34948=CARTESIAN_POINT ( 'NONE',  ( -418.0000000000000000, 144.9999999999999716, -155.0000000000000000 ) ) ;
#34950=LINE ( 'NONE', #21938, #16261 ) ;
#34951=DIRECTION ( 'NONE',  ( 1.000000000000000000, 0.000000000000000000, -1.232595164407831220E-32 ) ) ;
#34957=EDGE_LOOP ( 'NONE', ( #13066, #1369, #21972, #9700, #19408, #4192, #32851, #1514 ) ) ;
#34959=VERTEX_POINT ( 'NONE', #21677 ) ;
#34960=EDGE_CURVE ( 'NONE', #2214, #17376, #27544, .T. ) ;
#34961=AXIS2_PLACEMENT_3D ( 'NONE', #6444, #20348, #1471 ) ;
#34963=FACE_BOUND ( 'NONE', #19028, .T. ) ;
#34966=EDGE_CURVE ( 'NONE', #20509, #4608, #677, .T. ) ;
#34976=ADVANCED_FACE ( 'NONE', ( #30399 ), #27722, .T. ) ;
#34977=EDGE_LOOP ( 'NONE', ( #17956, #26204, #28305, #20734 ) ) ;
#34978=VECTOR ( 'NONE', #11583, 1000.000000000000000 ) ;
#34979=DIRECTION ( 'NONE',  ( 0.000000000000000000, 0.000000000000000000, 1.000000000000000000 ) ) ;
#34984=FACE_OUTER_BOUND ( 'NONE', #358, .T. ) ;
#34985=VERTEX_POINT ( 'NONE', #5994 ) ;
#34986=LINE ( 'NONE', #10599, #16253 ) ;
#34991=CYLINDRICAL_SURFACE ( 'NONE', #13485, 7.999999999999986677 ) ;
#34993=LINE ( 'NONE', #20928, #34825 ) ;
#35001=AXIS2_PLACEMENT_3D ( 'NONE', #33217, #33394, #19886 ) ;
#35005=CARTESIAN_POINT ( 'NONE',  ( -361.0000000000000000, 134.9999999999999716, 113.9999999999999858 ) ) ;
#35010=CARTESIAN_POINT ( 'NONE',  ( -19.99999999999998934, 124.9999999999999716, 162.9999999999999716 ) ) ;
#35012=CARTESIAN_POINT ( 'NONE',  ( -410.0000000000000568, -137.0000000000000000, -155.0000000000000000 ) ) ;
#35013=ADVANCED_FACE ( 'NONE', ( #30576 ), #11539, .T. ) ;
#35014=DIRECTION ( 'NONE',  ( 1.000000000000000000, 0.000000000000000000, 0.000000000000000000 ) ) ;
#35026=CARTESIAN_POINT ( 'NONE',  ( 11.99999999999999645, 144.9999999999999147, 155.0000000000000000 ) ) ;
#35029=CARTESIAN_POINT ( 'NONE',  ( 11.99999999999999645, -24.99999999999999289, 154.9999999999999716 ) ) ;
#35030=CARTESIAN_POINT ( 'NONE',  ( -70.00000000000000000, 4.559999999999909015, 177.7400000000000091 ) ) ;
#35039=VERTEX_POINT ( 'NONE', #9034 ) ;
#35042=CARTESIAN_POINT ( 'NONE',  ( -418.0000000000000000, -125.0000000000000000, 187.0000000000000000 ) ) ;
#35043=ADVANCED_FACE ( 'NONE', ( #12903, #20896 ), #28255, .T. ) ;
#35045=LINE ( 'NONE', #32183, #24502 ) ;
#35050=ORIENTED_EDGE ( 'NONE', *, *, #2197, .T. ) ;
#35051=EDGE_LOOP ( 'NONE', ( #6451, #9944, #3076, #1509 ) ) ;
#35053=PLANE ( 'NONE',  #34319 ) ;
#35055=AXIS2_PLACEMENT_3D ( 'NONE', #14873, #25527, #20210 ) ;
#35062=VERTEX_POINT ( 'NONE', #9211 ) ;
#35064=AXIS2_PLACEMENT_3D ( 'NONE', #25642, #1271, #3403 ) ;
#35065=AXIS2_PLACEMENT_3D ( 'NONE', #12448, #8877, #1399 ) ;
#35066=DIRECTION ( 'NONE',  ( 0.000000000000000000, 0.000000000000000000, -1.000000000000000000 ) ) ;
#35068=EDGE_LOOP ( 'NONE', ( #15215, #4888, #3916, #563 ) ) ;
#35069=VERTEX_POINT ( 'NONE', #30746 ) ;
#35071=ORIENTED_EDGE ( 'NONE', *, *, #20376, .T. ) ;
#35072=CARTESIAN_POINT ( 'NONE',  ( -430.0000000000000000, -131.0000000000000000, 126.0000000000000000 ) ) ;
#35077=PLANE ( 'NONE',  #1303 ) ;
#35080=FACE_OUTER_BOUND ( 'NONE', #27853, .T. ) ;
#35082=ADVANCED_FACE ( 'NONE', ( #14569 ), #25398, .T. ) ;
#35083=DIRECTION ( 'NONE',  ( 1.000000000000000000, 3.040835319149746090E-31, 1.232595164407830946E-32 ) ) ;
#35089=VECTOR ( 'NONE', #24056, 1000.000000000000000 ) ;
#35090=VECTOR ( 'NONE', #11263, 1000.000000000000000 ) ;
#35248=COLOUR_RGB('Dark Blue',0.08,0.2,0.34);
#35249=FILL_AREA_STYLE_COLOUR('',#35248);
#35250=FILL_AREA_STYLE('',(#35249));
#35251=SURFACE_STYLE_FILL_AREA(#35250);
#35252=SURFACE_SIDE_STYLE('',(#35251));
#35253=SURFACE_STYLE_USAGE(.BOTH.,#35252);
#35254=PRESENTATION_STYLE_ASSIGNMENT((#35253));
ENDSEC;
END-ISO-10303-21;
